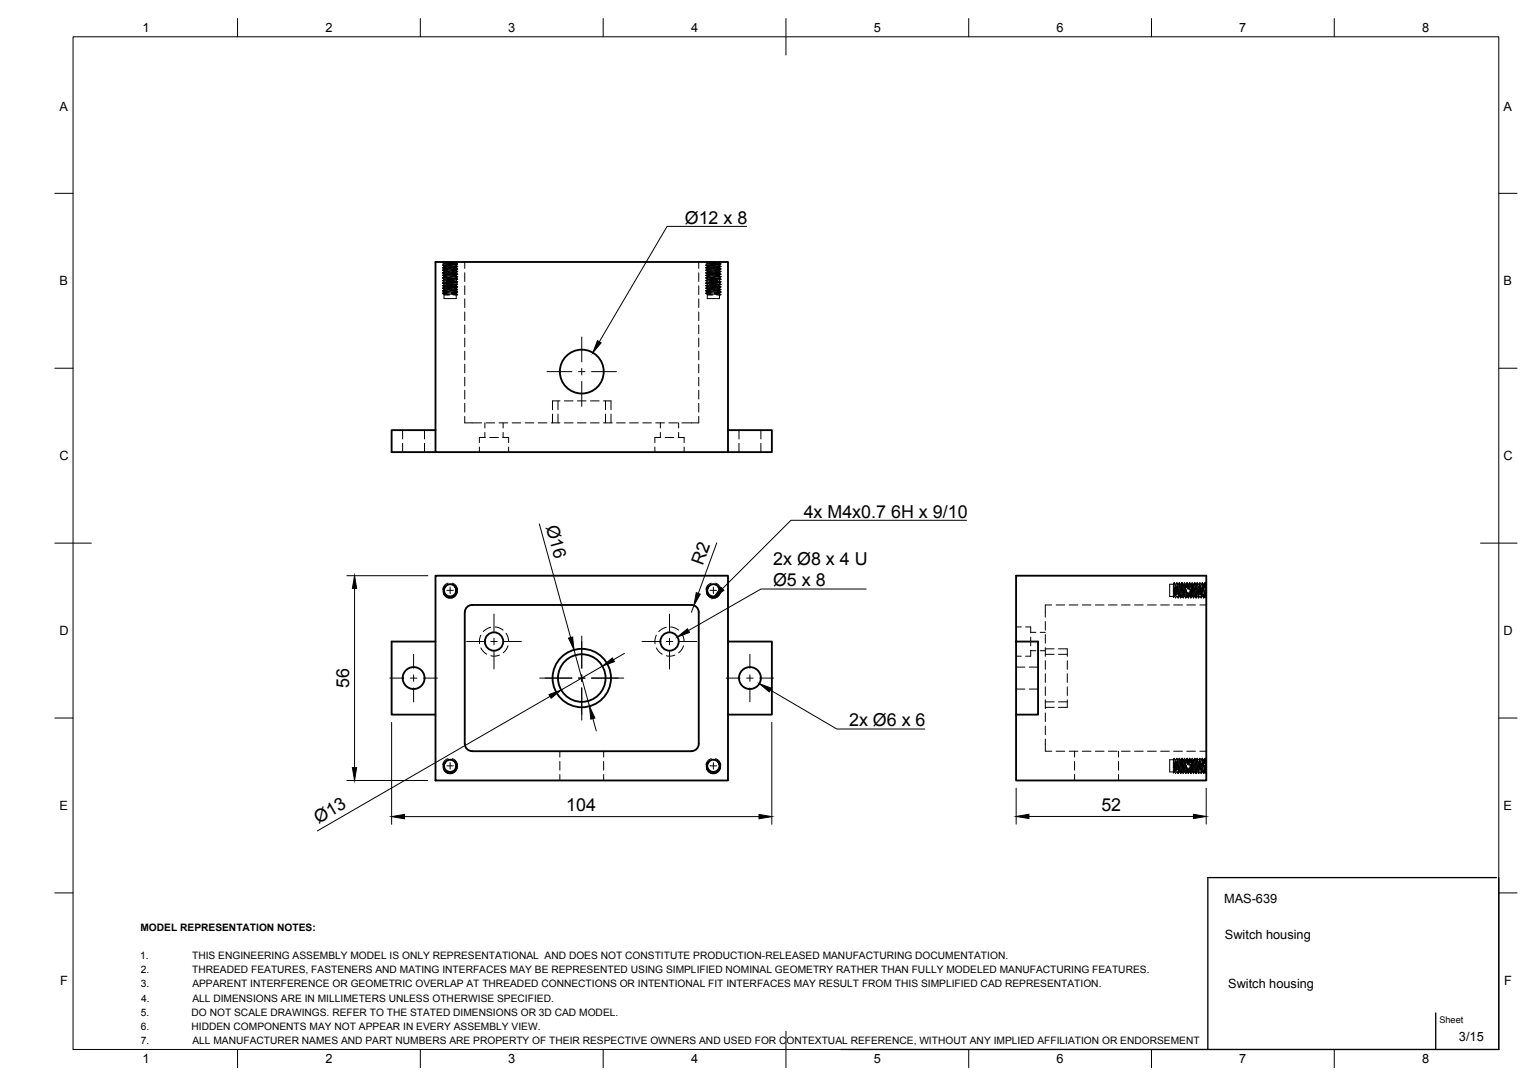
ISO-10303-21;
HEADER;
/* Generated by software containing ST-Developer
 * from STEP Tools, Inc. (www.steptools.com) 
 */

FILE_DESCRIPTION(
/* description */ ('Independent maintained push-to-latch/pull-to-reset mushroom-operator 
CAD. Two opposed spring-loaded ball detents in turned circular seats b
ias both travel stops; direct normally-closed bridge opens6mm when pre
ssed. Rounded palm/pull rim, captured head screw, removable detent clo
sures, native Coil spring families, insulated shared terminals and ord
inary machining features. Manual geometric states and ideal same-mater
ial spring-energy direction only; no electrical/safety certification, 
force/contact dynamics, wear, load or life rating. Requested blue/gray
 visual palette, not safety identification. External wiring/anchors an
d application engineering omitted.'),
/* implementation_level */ '2;1');

FILE_NAME(
/* name */ 'Switch housing.step',
/* time_stamp */ '2026-11-08T17:54:26-08:00',
/* author */ (''),
/* organization */ (''),
/* preprocessor_version */ 'ST-DEVELOPER v20.2',
/* originating_system */ 'Autodesk Translation Framework v15.17.0.0',
/* authorisation */ '');

FILE_SCHEMA (('AUTOMOTIVE_DESIGN { 1 0 10303 214 3 1 1 }'));
ENDSEC;

DATA;
#10=MECHANICAL_DESIGN_GEOMETRIC_PRESENTATION_REPRESENTATION('',(#190),#43980);
#156=SHAPE_REPRESENTATION_RELATIONSHIP('SRR','None',#44056,#173);
#173=ADVANCED_BREP_SHAPE_REPRESENTATION('',(#207),#43963);
#190=STYLED_ITEM('',(#44150),#207);
#207=MANIFOLD_SOLID_BREP('Body1',#11231);
#224=B_SPLINE_SURFACE_WITH_KNOTS('',3,3,((#18348,#18349,#18350,#18351,#18352,
#18353,#18354,#18355,#18356,#18357,#18358,#18359,#18360,#18361,#18362,#18363,
#18364,#18365,#18366,#18367,#18368,#18369,#18370,#18371,#18372,#18373,#18374,
#18375,#18376,#18377,#18378,#18379,#18380,#18381,#18382,#18383,#18384,#18385,
#18386,#18387,#18388,#18389,#18390,#18391,#18392,#18393,#18394,#18395,#18396,
#18397,#18398,#18399,#18400,#18401,#18402,#18403,#18404,#18405,#18406,#18407,
#18408,#18409,#18410,#18411,#18412,#18413,#18414,#18415,#18416,#18417,#18418,
#18419,#18420,#18421,#18422,#18423,#18424,#18425,#18426,#18427,#18428,#18429,
#18430,#18431,#18432,#18433),(#18434,#18435,#18436,#18437,#18438,#18439,
#18440,#18441,#18442,#18443,#18444,#18445,#18446,#18447,#18448,#18449,#18450,
#18451,#18452,#18453,#18454,#18455,#18456,#18457,#18458,#18459,#18460,#18461,
#18462,#18463,#18464,#18465,#18466,#18467,#18468,#18469,#18470,#18471,#18472,
#18473,#18474,#18475,#18476,#18477,#18478,#18479,#18480,#18481,#18482,#18483,
#18484,#18485,#18486,#18487,#18488,#18489,#18490,#18491,#18492,#18493,#18494,
#18495,#18496,#18497,#18498,#18499,#18500,#18501,#18502,#18503,#18504,#18505,
#18506,#18507,#18508,#18509,#18510,#18511,#18512,#18513,#18514,#18515,#18516,
#18517,#18518,#18519),(#18520,#18521,#18522,#18523,#18524,#18525,#18526,
#18527,#18528,#18529,#18530,#18531,#18532,#18533,#18534,#18535,#18536,#18537,
#18538,#18539,#18540,#18541,#18542,#18543,#18544,#18545,#18546,#18547,#18548,
#18549,#18550,#18551,#18552,#18553,#18554,#18555,#18556,#18557,#18558,#18559,
#18560,#18561,#18562,#18563,#18564,#18565,#18566,#18567,#18568,#18569,#18570,
#18571,#18572,#18573,#18574,#18575,#18576,#18577,#18578,#18579,#18580,#18581,
#18582,#18583,#18584,#18585,#18586,#18587,#18588,#18589,#18590,#18591,#18592,
#18593,#18594,#18595,#18596,#18597,#18598,#18599,#18600,#18601,#18602,#18603,
#18604,#18605),(#18606,#18607,#18608,#18609,#18610,#18611,#18612,#18613,
#18614,#18615,#18616,#18617,#18618,#18619,#18620,#18621,#18622,#18623,#18624,
#18625,#18626,#18627,#18628,#18629,#18630,#18631,#18632,#18633,#18634,#18635,
#18636,#18637,#18638,#18639,#18640,#18641,#18642,#18643,#18644,#18645,#18646,
#18647,#18648,#18649,#18650,#18651,#18652,#18653,#18654,#18655,#18656,#18657,
#18658,#18659,#18660,#18661,#18662,#18663,#18664,#18665,#18666,#18667,#18668,
#18669,#18670,#18671,#18672,#18673,#18674,#18675,#18676,#18677,#18678,#18679,
#18680,#18681,#18682,#18683,#18684,#18685,#18686,#18687,#18688,#18689,#18690,
#18691)),.UNSPECIFIED.,.F.,.F.,.F.,(4,4),(4,1,1,1,1,1,1,1,1,1,1,1,1,1,1,
1,1,1,1,1,1,1,1,1,1,1,1,1,1,1,1,1,1,1,1,1,1,1,1,1,1,1,1,1,1,1,1,1,1,1,1,
1,1,1,1,1,1,1,1,1,1,1,1,1,1,1,1,1,1,1,1,1,1,1,1,1,1,1,1,1,1,1,1,4),(0.,
0.0448889834294937),(11.8615800042567,12.8591513772396,13.8567227502226,
14.8542941232055,15.8518654961884,16.8494368691714,17.8470082421543,18.8445796151372,
19.8421509881202,20.8397223611031,21.837293734086,22.834865107069,23.8324364800519,
24.8300078530348,25.8275792260178,26.8251505990007,27.8227219719836,28.8202933449666,
29.8178647179495,30.8154360909324,31.8130074639154,32.8105788368983,33.8081502098812,
34.8057215828642,35.8032929558471,36.80086432883,37.798435701813,38.7960070747959,
39.7935784477789,40.7911498207618,41.7887211937447,42.7862925667277,43.7838639397106,
44.7814353126935,45.7790066856765,46.7765780586594,47.7741494316423,48.7717208046253,
49.7692921776082,50.7668635505911,51.7644349235741,52.762006296557,53.7595776695399,
54.7571490425229,55.7547204155058,56.7522917884887,57.7498631614717,58.7474345344546,
59.7450059074375,60.7425772804205,61.7401486534034,62.7377200263864,63.7352913993693,
64.7328627723522,65.7304341453352,66.7280055183181,67.725576891301,68.723148264284,
69.7207196372669,70.7182910102498,71.7158623832328,72.7134337562157,73.7110051291986,
74.7085765021816,75.7061478751645,76.7037192481474,77.7012906211304,78.6988619941133,
79.6964333670962,80.6940047400792,81.6915761130621,82.689147486045,83.686718859028,
84.6842902320109,85.6818616049939,86.6794329779768,87.6770043509597,88.6745757239427,
89.6721470969256,90.6697184699085,91.6672898428915,92.6648612158744,93.6624325888573,
94.6600039618403),.UNSPECIFIED.);
#225=B_SPLINE_SURFACE_WITH_KNOTS('',3,3,((#18769,#18770,#18771,#18772,#18773,
#18774,#18775,#18776,#18777,#18778,#18779,#18780,#18781,#18782,#18783,#18784,
#18785,#18786,#18787,#18788,#18789,#18790,#18791,#18792,#18793,#18794,#18795,
#18796,#18797,#18798,#18799,#18800,#18801,#18802,#18803,#18804,#18805,#18806,
#18807,#18808,#18809,#18810,#18811,#18812,#18813,#18814,#18815,#18816,#18817,
#18818,#18819,#18820,#18821,#18822,#18823,#18824,#18825,#18826,#18827,#18828,
#18829,#18830,#18831,#18832,#18833,#18834,#18835,#18836,#18837,#18838,#18839,
#18840,#18841,#18842,#18843,#18844,#18845,#18846,#18847,#18848,#18849,#18850,
#18851,#18852,#18853,#18854),(#18855,#18856,#18857,#18858,#18859,#18860,
#18861,#18862,#18863,#18864,#18865,#18866,#18867,#18868,#18869,#18870,#18871,
#18872,#18873,#18874,#18875,#18876,#18877,#18878,#18879,#18880,#18881,#18882,
#18883,#18884,#18885,#18886,#18887,#18888,#18889,#18890,#18891,#18892,#18893,
#18894,#18895,#18896,#18897,#18898,#18899,#18900,#18901,#18902,#18903,#18904,
#18905,#18906,#18907,#18908,#18909,#18910,#18911,#18912,#18913,#18914,#18915,
#18916,#18917,#18918,#18919,#18920,#18921,#18922,#18923,#18924,#18925,#18926,
#18927,#18928,#18929,#18930,#18931,#18932,#18933,#18934,#18935,#18936,#18937,
#18938,#18939,#18940),(#18941,#18942,#18943,#18944,#18945,#18946,#18947,
#18948,#18949,#18950,#18951,#18952,#18953,#18954,#18955,#18956,#18957,#18958,
#18959,#18960,#18961,#18962,#18963,#18964,#18965,#18966,#18967,#18968,#18969,
#18970,#18971,#18972,#18973,#18974,#18975,#18976,#18977,#18978,#18979,#18980,
#18981,#18982,#18983,#18984,#18985,#18986,#18987,#18988,#18989,#18990,#18991,
#18992,#18993,#18994,#18995,#18996,#18997,#18998,#18999,#19000,#19001,#19002,
#19003,#19004,#19005,#19006,#19007,#19008,#19009,#19010,#19011,#19012,#19013,
#19014,#19015,#19016,#19017,#19018,#19019,#19020,#19021,#19022,#19023,#19024,
#19025,#19026),(#19027,#19028,#19029,#19030,#19031,#19032,#19033,#19034,
#19035,#19036,#19037,#19038,#19039,#19040,#19041,#19042,#19043,#19044,#19045,
#19046,#19047,#19048,#19049,#19050,#19051,#19052,#19053,#19054,#19055,#19056,
#19057,#19058,#19059,#19060,#19061,#19062,#19063,#19064,#19065,#19066,#19067,
#19068,#19069,#19070,#19071,#19072,#19073,#19074,#19075,#19076,#19077,#19078,
#19079,#19080,#19081,#19082,#19083,#19084,#19085,#19086,#19087,#19088,#19089,
#19090,#19091,#19092,#19093,#19094,#19095,#19096,#19097,#19098,#19099,#19100,
#19101,#19102,#19103,#19104,#19105,#19106,#19107,#19108,#19109,#19110,#19111,
#19112)),.UNSPECIFIED.,.F.,.F.,.F.,(4,4),(4,1,1,1,1,1,1,1,1,1,1,1,1,1,1,
1,1,1,1,1,1,1,1,1,1,1,1,1,1,1,1,1,1,1,1,1,1,1,1,1,1,1,1,1,1,1,1,1,1,1,1,
1,1,1,1,1,1,1,1,1,1,1,1,1,1,1,1,1,1,1,1,1,1,1,1,1,1,1,1,1,1,1,1,4),(0.,
0.0448889834294937),(14.3981410127769,15.3957123857599,16.3932837587428,
17.3908551317257,18.3884265047087,19.3859978776916,20.3835692506745,21.3811406236575,
22.3787119966404,23.3762833696233,24.3738547426063,25.3714261155892,26.3689974885721,
27.3665688615551,28.364140234538,29.3617116075209,30.3592829805039,31.3568543534868,
32.3544257264697,33.3519970994527,34.3495684724356,35.3471398454185,36.3447112184015,
37.3422825913844,38.3398539643674,39.3374253373503,40.3349967103332,41.3325680833162,
42.3301394562991,43.327710829282,44.325282202265,45.3228535752479,46.3204249482308,
47.3179963212138,48.3155676941967,49.3131390671796,50.3107104401626,51.3082818131455,
52.3058531861284,53.3034245591114,54.3009959320943,55.2985673050772,56.2961386780602,
57.2937100510431,58.291281424026,59.288852797009,60.2864241699919,61.2839955429748,
62.2815669159578,63.2791382889407,64.2767096619236,65.2742810349066,66.2718524078895,
67.2694237808725,68.2669951538554,69.2645665268383,70.2621378998213,71.2597092728042,
72.2572806457871,73.2548520187701,74.252423391753,75.2499947647359,76.2475661377189,
77.2451375107018,78.2427088836847,79.2402802566677,80.2378516296506,81.2354230026336,
82.2329943756165,83.2305657485994,84.2281371215823,85.2257084945653,86.2232798675482,
87.2208512405312,88.2184226135141,89.215993986497,90.21356535948,91.2111367324629,
92.2087081054458,93.2062794784288,94.2038508514117,95.2014222243946,96.1989935973776,
97.1965649703605),.UNSPECIFIED.);
#226=B_SPLINE_SURFACE_WITH_KNOTS('',3,3,((#19321,#19322,#19323,#19324,#19325,
#19326,#19327,#19328,#19329,#19330,#19331,#19332,#19333,#19334,#19335,#19336,
#19337,#19338,#19339,#19340,#19341,#19342,#19343,#19344,#19345,#19346,#19347,
#19348,#19349,#19350,#19351,#19352,#19353,#19354,#19355,#19356,#19357,#19358,
#19359,#19360,#19361,#19362,#19363,#19364,#19365,#19366,#19367,#19368,#19369,
#19370,#19371,#19372,#19373,#19374,#19375,#19376,#19377,#19378,#19379,#19380,
#19381,#19382,#19383,#19384,#19385,#19386,#19387,#19388,#19389,#19390,#19391,
#19392,#19393,#19394,#19395,#19396,#19397,#19398,#19399,#19400,#19401,#19402,
#19403,#19404,#19405,#19406),(#19407,#19408,#19409,#19410,#19411,#19412,
#19413,#19414,#19415,#19416,#19417,#19418,#19419,#19420,#19421,#19422,#19423,
#19424,#19425,#19426,#19427,#19428,#19429,#19430,#19431,#19432,#19433,#19434,
#19435,#19436,#19437,#19438,#19439,#19440,#19441,#19442,#19443,#19444,#19445,
#19446,#19447,#19448,#19449,#19450,#19451,#19452,#19453,#19454,#19455,#19456,
#19457,#19458,#19459,#19460,#19461,#19462,#19463,#19464,#19465,#19466,#19467,
#19468,#19469,#19470,#19471,#19472,#19473,#19474,#19475,#19476,#19477,#19478,
#19479,#19480,#19481,#19482,#19483,#19484,#19485,#19486,#19487,#19488,#19489,
#19490,#19491,#19492),(#19493,#19494,#19495,#19496,#19497,#19498,#19499,
#19500,#19501,#19502,#19503,#19504,#19505,#19506,#19507,#19508,#19509,#19510,
#19511,#19512,#19513,#19514,#19515,#19516,#19517,#19518,#19519,#19520,#19521,
#19522,#19523,#19524,#19525,#19526,#19527,#19528,#19529,#19530,#19531,#19532,
#19533,#19534,#19535,#19536,#19537,#19538,#19539,#19540,#19541,#19542,#19543,
#19544,#19545,#19546,#19547,#19548,#19549,#19550,#19551,#19552,#19553,#19554,
#19555,#19556,#19557,#19558,#19559,#19560,#19561,#19562,#19563,#19564,#19565,
#19566,#19567,#19568,#19569,#19570,#19571,#19572,#19573,#19574,#19575,#19576,
#19577,#19578),(#19579,#19580,#19581,#19582,#19583,#19584,#19585,#19586,
#19587,#19588,#19589,#19590,#19591,#19592,#19593,#19594,#19595,#19596,#19597,
#19598,#19599,#19600,#19601,#19602,#19603,#19604,#19605,#19606,#19607,#19608,
#19609,#19610,#19611,#19612,#19613,#19614,#19615,#19616,#19617,#19618,#19619,
#19620,#19621,#19622,#19623,#19624,#19625,#19626,#19627,#19628,#19629,#19630,
#19631,#19632,#19633,#19634,#19635,#19636,#19637,#19638,#19639,#19640,#19641,
#19642,#19643,#19644,#19645,#19646,#19647,#19648,#19649,#19650,#19651,#19652,
#19653,#19654,#19655,#19656,#19657,#19658,#19659,#19660,#19661,#19662,#19663,
#19664)),.UNSPECIFIED.,.F.,.F.,.F.,(4,4),(4,1,1,1,1,1,1,1,1,1,1,1,1,1,1,
1,1,1,1,1,1,1,1,1,1,1,1,1,1,1,1,1,1,1,1,1,1,1,1,1,1,1,1,1,1,1,1,1,1,1,1,
1,1,1,1,1,1,1,1,1,1,1,1,1,1,1,1,1,1,1,1,1,1,1,1,1,1,1,1,1,1,1,1,4),(0.,
0.0448889834294937),(11.8615800042567,12.8591513772396,13.8567227502225,
14.8542941232055,15.8518654961884,16.8494368691713,17.8470082421543,18.8445796151372,
19.8421509881202,20.8397223611031,21.837293734086,22.834865107069,23.8324364800519,
24.8300078530348,25.8275792260178,26.8251505990007,27.8227219719836,28.8202933449666,
29.8178647179495,30.8154360909324,31.8130074639154,32.8105788368983,33.8081502098812,
34.8057215828642,35.8032929558471,36.80086432883,37.798435701813,38.7960070747959,
39.7935784477788,40.7911498207618,41.7887211937447,42.7862925667276,43.7838639397106,
44.7814353126935,45.7790066856764,46.7765780586594,47.7741494316423,48.7717208046252,
49.7692921776082,50.7668635505911,51.764434923574,52.762006296557,53.7595776695399,
54.7571490425228,55.7547204155058,56.7522917884887,57.7498631614716,58.7474345344546,
59.7450059074375,60.7425772804204,61.7401486534034,62.7377200263863,63.7352913993692,
64.7328627723522,65.7304341453351,66.728005518318,67.725576891301,68.7231482642839,
69.7207196372669,70.7182910102498,71.7158623832327,72.7134337562156,73.7110051291986,
74.7085765021815,75.7061478751644,76.7037192481474,77.7012906211303,78.6988619941132,
79.6964333670962,80.6940047400791,81.6915761130621,82.689147486045,83.6867188590279,
84.6842902320109,85.6818616049938,86.6794329779767,87.6770043509596,88.6745757239426,
89.6721470969255,90.6697184699085,91.6672898428914,92.6648612158743,93.6624325888573,
94.6600039618402),.UNSPECIFIED.);
#227=B_SPLINE_SURFACE_WITH_KNOTS('',3,3,((#19742,#19743,#19744,#19745,#19746,
#19747,#19748,#19749,#19750,#19751,#19752,#19753,#19754,#19755,#19756,#19757,
#19758,#19759,#19760,#19761,#19762,#19763,#19764,#19765,#19766,#19767,#19768,
#19769,#19770,#19771,#19772,#19773,#19774,#19775,#19776,#19777,#19778,#19779,
#19780,#19781,#19782,#19783,#19784,#19785,#19786,#19787,#19788,#19789,#19790,
#19791,#19792,#19793,#19794,#19795,#19796,#19797,#19798,#19799,#19800,#19801,
#19802,#19803,#19804,#19805,#19806,#19807,#19808,#19809,#19810,#19811,#19812,
#19813,#19814,#19815,#19816,#19817,#19818,#19819,#19820,#19821,#19822,#19823,
#19824,#19825,#19826,#19827),(#19828,#19829,#19830,#19831,#19832,#19833,
#19834,#19835,#19836,#19837,#19838,#19839,#19840,#19841,#19842,#19843,#19844,
#19845,#19846,#19847,#19848,#19849,#19850,#19851,#19852,#19853,#19854,#19855,
#19856,#19857,#19858,#19859,#19860,#19861,#19862,#19863,#19864,#19865,#19866,
#19867,#19868,#19869,#19870,#19871,#19872,#19873,#19874,#19875,#19876,#19877,
#19878,#19879,#19880,#19881,#19882,#19883,#19884,#19885,#19886,#19887,#19888,
#19889,#19890,#19891,#19892,#19893,#19894,#19895,#19896,#19897,#19898,#19899,
#19900,#19901,#19902,#19903,#19904,#19905,#19906,#19907,#19908,#19909,#19910,
#19911,#19912,#19913),(#19914,#19915,#19916,#19917,#19918,#19919,#19920,
#19921,#19922,#19923,#19924,#19925,#19926,#19927,#19928,#19929,#19930,#19931,
#19932,#19933,#19934,#19935,#19936,#19937,#19938,#19939,#19940,#19941,#19942,
#19943,#19944,#19945,#19946,#19947,#19948,#19949,#19950,#19951,#19952,#19953,
#19954,#19955,#19956,#19957,#19958,#19959,#19960,#19961,#19962,#19963,#19964,
#19965,#19966,#19967,#19968,#19969,#19970,#19971,#19972,#19973,#19974,#19975,
#19976,#19977,#19978,#19979,#19980,#19981,#19982,#19983,#19984,#19985,#19986,
#19987,#19988,#19989,#19990,#19991,#19992,#19993,#19994,#19995,#19996,#19997,
#19998,#19999),(#20000,#20001,#20002,#20003,#20004,#20005,#20006,#20007,
#20008,#20009,#20010,#20011,#20012,#20013,#20014,#20015,#20016,#20017,#20018,
#20019,#20020,#20021,#20022,#20023,#20024,#20025,#20026,#20027,#20028,#20029,
#20030,#20031,#20032,#20033,#20034,#20035,#20036,#20037,#20038,#20039,#20040,
#20041,#20042,#20043,#20044,#20045,#20046,#20047,#20048,#20049,#20050,#20051,
#20052,#20053,#20054,#20055,#20056,#20057,#20058,#20059,#20060,#20061,#20062,
#20063,#20064,#20065,#20066,#20067,#20068,#20069,#20070,#20071,#20072,#20073,
#20074,#20075,#20076,#20077,#20078,#20079,#20080,#20081,#20082,#20083,#20084,
#20085)),.UNSPECIFIED.,.F.,.F.,.F.,(4,4),(4,1,1,1,1,1,1,1,1,1,1,1,1,1,1,
1,1,1,1,1,1,1,1,1,1,1,1,1,1,1,1,1,1,1,1,1,1,1,1,1,1,1,1,1,1,1,1,1,1,1,1,
1,1,1,1,1,1,1,1,1,1,1,1,1,1,1,1,1,1,1,1,1,1,1,1,1,1,1,1,1,1,1,1,4),(0.,
0.0448889834294937),(14.3981410127769,15.3957123857599,16.3932837587428,
17.3908551317257,18.3884265047087,19.3859978776916,20.3835692506745,21.3811406236575,
22.3787119966404,23.3762833696233,24.3738547426063,25.3714261155892,26.3689974885721,
27.3665688615551,28.364140234538,29.3617116075209,30.3592829805039,31.3568543534868,
32.3544257264697,33.3519970994527,34.3495684724356,35.3471398454185,36.3447112184015,
37.3422825913844,38.3398539643673,39.3374253373503,40.3349967103332,41.3325680833161,
42.3301394562991,43.327710829282,44.3252822022649,45.3228535752479,46.3204249482308,
47.3179963212137,48.3155676941967,49.3131390671796,50.3107104401625,51.3082818131455,
52.3058531861284,53.3034245591113,54.3009959320943,55.2985673050772,56.2961386780601,
57.2937100510431,58.291281424026,59.2888527970089,60.2864241699919,61.2839955429748,
62.2815669159577,63.2791382889407,64.2767096619236,65.2742810349065,66.2718524078895,
67.2694237808724,68.2669951538553,69.2645665268383,70.2621378998212,71.2597092728041,
72.2572806457871,73.25485201877,74.2524233917529,75.2499947647359,76.2475661377188,
77.2451375107017,78.2427088836847,79.2402802566676,80.2378516296505,81.2354230026335,
82.2329943756164,83.2305657485993,84.2281371215823,85.2257084945652,86.2232798675481,
87.2208512405311,88.218422613514,89.2159939864969,90.2135653594799,91.2111367324628,
92.2087081054457,93.2062794784287,94.2038508514116,95.2014222243945,96.1989935973775,
97.1965649703604),.UNSPECIFIED.);
#228=B_SPLINE_SURFACE_WITH_KNOTS('',3,3,((#20294,#20295,#20296,#20297,#20298,
#20299,#20300,#20301,#20302,#20303,#20304,#20305,#20306,#20307,#20308,#20309,
#20310,#20311,#20312,#20313,#20314,#20315,#20316,#20317,#20318,#20319,#20320,
#20321,#20322,#20323,#20324,#20325,#20326,#20327,#20328,#20329,#20330,#20331,
#20332,#20333,#20334,#20335,#20336,#20337,#20338,#20339,#20340,#20341,#20342,
#20343,#20344,#20345,#20346,#20347,#20348,#20349,#20350,#20351,#20352,#20353,
#20354,#20355,#20356,#20357,#20358,#20359,#20360,#20361,#20362,#20363,#20364,
#20365,#20366,#20367,#20368,#20369,#20370,#20371,#20372,#20373,#20374,#20375,
#20376,#20377,#20378,#20379),(#20380,#20381,#20382,#20383,#20384,#20385,
#20386,#20387,#20388,#20389,#20390,#20391,#20392,#20393,#20394,#20395,#20396,
#20397,#20398,#20399,#20400,#20401,#20402,#20403,#20404,#20405,#20406,#20407,
#20408,#20409,#20410,#20411,#20412,#20413,#20414,#20415,#20416,#20417,#20418,
#20419,#20420,#20421,#20422,#20423,#20424,#20425,#20426,#20427,#20428,#20429,
#20430,#20431,#20432,#20433,#20434,#20435,#20436,#20437,#20438,#20439,#20440,
#20441,#20442,#20443,#20444,#20445,#20446,#20447,#20448,#20449,#20450,#20451,
#20452,#20453,#20454,#20455,#20456,#20457,#20458,#20459,#20460,#20461,#20462,
#20463,#20464,#20465),(#20466,#20467,#20468,#20469,#20470,#20471,#20472,
#20473,#20474,#20475,#20476,#20477,#20478,#20479,#20480,#20481,#20482,#20483,
#20484,#20485,#20486,#20487,#20488,#20489,#20490,#20491,#20492,#20493,#20494,
#20495,#20496,#20497,#20498,#20499,#20500,#20501,#20502,#20503,#20504,#20505,
#20506,#20507,#20508,#20509,#20510,#20511,#20512,#20513,#20514,#20515,#20516,
#20517,#20518,#20519,#20520,#20521,#20522,#20523,#20524,#20525,#20526,#20527,
#20528,#20529,#20530,#20531,#20532,#20533,#20534,#20535,#20536,#20537,#20538,
#20539,#20540,#20541,#20542,#20543,#20544,#20545,#20546,#20547,#20548,#20549,
#20550,#20551),(#20552,#20553,#20554,#20555,#20556,#20557,#20558,#20559,
#20560,#20561,#20562,#20563,#20564,#20565,#20566,#20567,#20568,#20569,#20570,
#20571,#20572,#20573,#20574,#20575,#20576,#20577,#20578,#20579,#20580,#20581,
#20582,#20583,#20584,#20585,#20586,#20587,#20588,#20589,#20590,#20591,#20592,
#20593,#20594,#20595,#20596,#20597,#20598,#20599,#20600,#20601,#20602,#20603,
#20604,#20605,#20606,#20607,#20608,#20609,#20610,#20611,#20612,#20613,#20614,
#20615,#20616,#20617,#20618,#20619,#20620,#20621,#20622,#20623,#20624,#20625,
#20626,#20627,#20628,#20629,#20630,#20631,#20632,#20633,#20634,#20635,#20636,
#20637)),.UNSPECIFIED.,.F.,.F.,.F.,(4,4),(4,1,1,1,1,1,1,1,1,1,1,1,1,1,1,
1,1,1,1,1,1,1,1,1,1,1,1,1,1,1,1,1,1,1,1,1,1,1,1,1,1,1,1,1,1,1,1,1,1,1,1,
1,1,1,1,1,1,1,1,1,1,1,1,1,1,1,1,1,1,1,1,1,1,1,1,1,1,1,1,1,1,1,1,4),(0.,
0.0448889834294937),(11.8615800042567,12.8591513772396,13.8567227502225,
14.8542941232055,15.8518654961884,16.8494368691713,17.8470082421543,18.8445796151372,
19.8421509881201,20.8397223611031,21.837293734086,22.8348651070689,23.8324364800519,
24.8300078530348,25.8275792260178,26.8251505990007,27.8227219719836,28.8202933449666,
29.8178647179495,30.8154360909324,31.8130074639154,32.8105788368983,33.8081502098812,
34.8057215828642,35.8032929558471,36.80086432883,37.798435701813,38.7960070747959,
39.7935784477788,40.7911498207618,41.7887211937447,42.7862925667276,43.7838639397106,
44.7814353126935,45.7790066856764,46.7765780586594,47.7741494316423,48.7717208046252,
49.7692921776082,50.7668635505911,51.764434923574,52.762006296557,53.7595776695399,
54.7571490425228,55.7547204155058,56.7522917884887,57.7498631614716,58.7474345344546,
59.7450059074375,60.7425772804204,61.7401486534034,62.7377200263863,63.7352913993692,
64.7328627723522,65.7304341453351,66.728005518318,67.725576891301,68.7231482642839,
69.7207196372668,70.7182910102498,71.7158623832327,72.7134337562156,73.7110051291986,
74.7085765021815,75.7061478751644,76.7037192481474,77.7012906211303,78.6988619941132,
79.6964333670962,80.6940047400791,81.6915761130621,82.689147486045,83.6867188590279,
84.6842902320109,85.6818616049938,86.6794329779767,87.6770043509596,88.6745757239426,
89.6721470969255,90.6697184699085,91.6672898428914,92.6648612158743,93.6624325888573,
94.6600039618402),.UNSPECIFIED.);
#229=B_SPLINE_SURFACE_WITH_KNOTS('',3,3,((#20715,#20716,#20717,#20718,#20719,
#20720,#20721,#20722,#20723,#20724,#20725,#20726,#20727,#20728,#20729,#20730,
#20731,#20732,#20733,#20734,#20735,#20736,#20737,#20738,#20739,#20740,#20741,
#20742,#20743,#20744,#20745,#20746,#20747,#20748,#20749,#20750,#20751,#20752,
#20753,#20754,#20755,#20756,#20757,#20758,#20759,#20760,#20761,#20762,#20763,
#20764,#20765,#20766,#20767,#20768,#20769,#20770,#20771,#20772,#20773,#20774,
#20775,#20776,#20777,#20778,#20779,#20780,#20781,#20782,#20783,#20784,#20785,
#20786,#20787,#20788,#20789,#20790,#20791,#20792,#20793,#20794,#20795,#20796,
#20797,#20798,#20799,#20800),(#20801,#20802,#20803,#20804,#20805,#20806,
#20807,#20808,#20809,#20810,#20811,#20812,#20813,#20814,#20815,#20816,#20817,
#20818,#20819,#20820,#20821,#20822,#20823,#20824,#20825,#20826,#20827,#20828,
#20829,#20830,#20831,#20832,#20833,#20834,#20835,#20836,#20837,#20838,#20839,
#20840,#20841,#20842,#20843,#20844,#20845,#20846,#20847,#20848,#20849,#20850,
#20851,#20852,#20853,#20854,#20855,#20856,#20857,#20858,#20859,#20860,#20861,
#20862,#20863,#20864,#20865,#20866,#20867,#20868,#20869,#20870,#20871,#20872,
#20873,#20874,#20875,#20876,#20877,#20878,#20879,#20880,#20881,#20882,#20883,
#20884,#20885,#20886),(#20887,#20888,#20889,#20890,#20891,#20892,#20893,
#20894,#20895,#20896,#20897,#20898,#20899,#20900,#20901,#20902,#20903,#20904,
#20905,#20906,#20907,#20908,#20909,#20910,#20911,#20912,#20913,#20914,#20915,
#20916,#20917,#20918,#20919,#20920,#20921,#20922,#20923,#20924,#20925,#20926,
#20927,#20928,#20929,#20930,#20931,#20932,#20933,#20934,#20935,#20936,#20937,
#20938,#20939,#20940,#20941,#20942,#20943,#20944,#20945,#20946,#20947,#20948,
#20949,#20950,#20951,#20952,#20953,#20954,#20955,#20956,#20957,#20958,#20959,
#20960,#20961,#20962,#20963,#20964,#20965,#20966,#20967,#20968,#20969,#20970,
#20971,#20972),(#20973,#20974,#20975,#20976,#20977,#20978,#20979,#20980,
#20981,#20982,#20983,#20984,#20985,#20986,#20987,#20988,#20989,#20990,#20991,
#20992,#20993,#20994,#20995,#20996,#20997,#20998,#20999,#21000,#21001,#21002,
#21003,#21004,#21005,#21006,#21007,#21008,#21009,#21010,#21011,#21012,#21013,
#21014,#21015,#21016,#21017,#21018,#21019,#21020,#21021,#21022,#21023,#21024,
#21025,#21026,#21027,#21028,#21029,#21030,#21031,#21032,#21033,#21034,#21035,
#21036,#21037,#21038,#21039,#21040,#21041,#21042,#21043,#21044,#21045,#21046,
#21047,#21048,#21049,#21050,#21051,#21052,#21053,#21054,#21055,#21056,#21057,
#21058)),.UNSPECIFIED.,.F.,.F.,.F.,(4,4),(4,1,1,1,1,1,1,1,1,1,1,1,1,1,1,
1,1,1,1,1,1,1,1,1,1,1,1,1,1,1,1,1,1,1,1,1,1,1,1,1,1,1,1,1,1,1,1,1,1,1,1,
1,1,1,1,1,1,1,1,1,1,1,1,1,1,1,1,1,1,1,1,1,1,1,1,1,1,1,1,1,1,1,1,4),(0.,
0.0448889834294937),(14.3981410127769,15.3957123857599,16.3932837587428,
17.3908551317257,18.3884265047087,19.3859978776916,20.3835692506745,21.3811406236575,
22.3787119966404,23.3762833696233,24.3738547426063,25.3714261155892,26.3689974885721,
27.3665688615551,28.364140234538,29.3617116075209,30.3592829805039,31.3568543534868,
32.3544257264697,33.3519970994527,34.3495684724356,35.3471398454185,36.3447112184015,
37.3422825913844,38.3398539643673,39.3374253373503,40.3349967103332,41.3325680833161,
42.3301394562991,43.327710829282,44.3252822022649,45.3228535752479,46.3204249482308,
47.3179963212137,48.3155676941967,49.3131390671796,50.3107104401625,51.3082818131455,
52.3058531861284,53.3034245591113,54.3009959320943,55.2985673050772,56.2961386780601,
57.2937100510431,58.291281424026,59.2888527970089,60.2864241699919,61.2839955429748,
62.2815669159577,63.2791382889407,64.2767096619236,65.2742810349065,66.2718524078895,
67.2694237808724,68.2669951538553,69.2645665268383,70.2621378998212,71.2597092728041,
72.2572806457871,73.25485201877,74.2524233917529,75.2499947647359,76.2475661377188,
77.2451375107017,78.2427088836847,79.2402802566676,80.2378516296505,81.2354230026335,
82.2329943756164,83.2305657485993,84.2281371215823,85.2257084945652,86.2232798675481,
87.2208512405311,88.218422613514,89.2159939864969,90.2135653594799,91.2111367324628,
92.2087081054457,93.2062794784287,94.2038508514116,95.2014222243945,96.1989935973775,
97.1965649703604),.UNSPECIFIED.);
#230=B_SPLINE_SURFACE_WITH_KNOTS('',3,3,((#21267,#21268,#21269,#21270,#21271,
#21272,#21273,#21274,#21275,#21276,#21277,#21278,#21279,#21280,#21281,#21282,
#21283,#21284,#21285,#21286,#21287,#21288,#21289,#21290,#21291,#21292,#21293,
#21294,#21295,#21296,#21297,#21298,#21299,#21300,#21301,#21302,#21303,#21304,
#21305,#21306,#21307,#21308,#21309,#21310,#21311,#21312,#21313,#21314,#21315,
#21316,#21317,#21318,#21319,#21320,#21321,#21322,#21323,#21324,#21325,#21326,
#21327,#21328,#21329,#21330,#21331,#21332,#21333,#21334,#21335,#21336,#21337,
#21338,#21339,#21340,#21341,#21342,#21343,#21344,#21345,#21346,#21347,#21348,
#21349,#21350,#21351,#21352),(#21353,#21354,#21355,#21356,#21357,#21358,
#21359,#21360,#21361,#21362,#21363,#21364,#21365,#21366,#21367,#21368,#21369,
#21370,#21371,#21372,#21373,#21374,#21375,#21376,#21377,#21378,#21379,#21380,
#21381,#21382,#21383,#21384,#21385,#21386,#21387,#21388,#21389,#21390,#21391,
#21392,#21393,#21394,#21395,#21396,#21397,#21398,#21399,#21400,#21401,#21402,
#21403,#21404,#21405,#21406,#21407,#21408,#21409,#21410,#21411,#21412,#21413,
#21414,#21415,#21416,#21417,#21418,#21419,#21420,#21421,#21422,#21423,#21424,
#21425,#21426,#21427,#21428,#21429,#21430,#21431,#21432,#21433,#21434,#21435,
#21436,#21437,#21438),(#21439,#21440,#21441,#21442,#21443,#21444,#21445,
#21446,#21447,#21448,#21449,#21450,#21451,#21452,#21453,#21454,#21455,#21456,
#21457,#21458,#21459,#21460,#21461,#21462,#21463,#21464,#21465,#21466,#21467,
#21468,#21469,#21470,#21471,#21472,#21473,#21474,#21475,#21476,#21477,#21478,
#21479,#21480,#21481,#21482,#21483,#21484,#21485,#21486,#21487,#21488,#21489,
#21490,#21491,#21492,#21493,#21494,#21495,#21496,#21497,#21498,#21499,#21500,
#21501,#21502,#21503,#21504,#21505,#21506,#21507,#21508,#21509,#21510,#21511,
#21512,#21513,#21514,#21515,#21516,#21517,#21518,#21519,#21520,#21521,#21522,
#21523,#21524),(#21525,#21526,#21527,#21528,#21529,#21530,#21531,#21532,
#21533,#21534,#21535,#21536,#21537,#21538,#21539,#21540,#21541,#21542,#21543,
#21544,#21545,#21546,#21547,#21548,#21549,#21550,#21551,#21552,#21553,#21554,
#21555,#21556,#21557,#21558,#21559,#21560,#21561,#21562,#21563,#21564,#21565,
#21566,#21567,#21568,#21569,#21570,#21571,#21572,#21573,#21574,#21575,#21576,
#21577,#21578,#21579,#21580,#21581,#21582,#21583,#21584,#21585,#21586,#21587,
#21588,#21589,#21590,#21591,#21592,#21593,#21594,#21595,#21596,#21597,#21598,
#21599,#21600,#21601,#21602,#21603,#21604,#21605,#21606,#21607,#21608,#21609,
#21610)),.UNSPECIFIED.,.F.,.F.,.F.,(4,4),(4,1,1,1,1,1,1,1,1,1,1,1,1,1,1,
1,1,1,1,1,1,1,1,1,1,1,1,1,1,1,1,1,1,1,1,1,1,1,1,1,1,1,1,1,1,1,1,1,1,1,1,
1,1,1,1,1,1,1,1,1,1,1,1,1,1,1,1,1,1,1,1,1,1,1,1,1,1,1,1,1,1,1,1,4),(0.,
0.0448889834294937),(11.8615800042567,12.8591513772396,13.8567227502226,
14.8542941232055,15.8518654961884,16.8494368691714,17.8470082421543,18.8445796151372,
19.8421509881202,20.8397223611031,21.837293734086,22.834865107069,23.8324364800519,
24.8300078530348,25.8275792260178,26.8251505990007,27.8227219719836,28.8202933449666,
29.8178647179495,30.8154360909324,31.8130074639154,32.8105788368983,33.8081502098812,
34.8057215828642,35.8032929558471,36.80086432883,37.798435701813,38.7960070747959,
39.7935784477789,40.7911498207618,41.7887211937447,42.7862925667277,43.7838639397106,
44.7814353126935,45.7790066856765,46.7765780586594,47.7741494316423,48.7717208046253,
49.7692921776082,50.7668635505911,51.7644349235741,52.762006296557,53.7595776695399,
54.7571490425229,55.7547204155058,56.7522917884887,57.7498631614717,58.7474345344546,
59.7450059074375,60.7425772804205,61.7401486534034,62.7377200263864,63.7352913993693,
64.7328627723522,65.7304341453352,66.7280055183181,67.725576891301,68.723148264284,
69.7207196372669,70.7182910102498,71.7158623832328,72.7134337562157,73.7110051291986,
74.7085765021816,75.7061478751645,76.7037192481474,77.7012906211304,78.6988619941133,
79.6964333670962,80.6940047400792,81.6915761130621,82.689147486045,83.686718859028,
84.6842902320109,85.6818616049939,86.6794329779768,87.6770043509597,88.6745757239427,
89.6721470969256,90.6697184699085,91.6672898428915,92.6648612158744,93.6624325888573,
94.6600039618403),.UNSPECIFIED.);
#231=B_SPLINE_SURFACE_WITH_KNOTS('',3,3,((#21688,#21689,#21690,#21691,#21692,
#21693,#21694,#21695,#21696,#21697,#21698,#21699,#21700,#21701,#21702,#21703,
#21704,#21705,#21706,#21707,#21708,#21709,#21710,#21711,#21712,#21713,#21714,
#21715,#21716,#21717,#21718,#21719,#21720,#21721,#21722,#21723,#21724,#21725,
#21726,#21727,#21728,#21729,#21730,#21731,#21732,#21733,#21734,#21735,#21736,
#21737,#21738,#21739,#21740,#21741,#21742,#21743,#21744,#21745,#21746,#21747,
#21748,#21749,#21750,#21751,#21752,#21753,#21754,#21755,#21756,#21757,#21758,
#21759,#21760,#21761,#21762,#21763,#21764,#21765,#21766,#21767,#21768,#21769,
#21770,#21771,#21772,#21773),(#21774,#21775,#21776,#21777,#21778,#21779,
#21780,#21781,#21782,#21783,#21784,#21785,#21786,#21787,#21788,#21789,#21790,
#21791,#21792,#21793,#21794,#21795,#21796,#21797,#21798,#21799,#21800,#21801,
#21802,#21803,#21804,#21805,#21806,#21807,#21808,#21809,#21810,#21811,#21812,
#21813,#21814,#21815,#21816,#21817,#21818,#21819,#21820,#21821,#21822,#21823,
#21824,#21825,#21826,#21827,#21828,#21829,#21830,#21831,#21832,#21833,#21834,
#21835,#21836,#21837,#21838,#21839,#21840,#21841,#21842,#21843,#21844,#21845,
#21846,#21847,#21848,#21849,#21850,#21851,#21852,#21853,#21854,#21855,#21856,
#21857,#21858,#21859),(#21860,#21861,#21862,#21863,#21864,#21865,#21866,
#21867,#21868,#21869,#21870,#21871,#21872,#21873,#21874,#21875,#21876,#21877,
#21878,#21879,#21880,#21881,#21882,#21883,#21884,#21885,#21886,#21887,#21888,
#21889,#21890,#21891,#21892,#21893,#21894,#21895,#21896,#21897,#21898,#21899,
#21900,#21901,#21902,#21903,#21904,#21905,#21906,#21907,#21908,#21909,#21910,
#21911,#21912,#21913,#21914,#21915,#21916,#21917,#21918,#21919,#21920,#21921,
#21922,#21923,#21924,#21925,#21926,#21927,#21928,#21929,#21930,#21931,#21932,
#21933,#21934,#21935,#21936,#21937,#21938,#21939,#21940,#21941,#21942,#21943,
#21944,#21945),(#21946,#21947,#21948,#21949,#21950,#21951,#21952,#21953,
#21954,#21955,#21956,#21957,#21958,#21959,#21960,#21961,#21962,#21963,#21964,
#21965,#21966,#21967,#21968,#21969,#21970,#21971,#21972,#21973,#21974,#21975,
#21976,#21977,#21978,#21979,#21980,#21981,#21982,#21983,#21984,#21985,#21986,
#21987,#21988,#21989,#21990,#21991,#21992,#21993,#21994,#21995,#21996,#21997,
#21998,#21999,#22000,#22001,#22002,#22003,#22004,#22005,#22006,#22007,#22008,
#22009,#22010,#22011,#22012,#22013,#22014,#22015,#22016,#22017,#22018,#22019,
#22020,#22021,#22022,#22023,#22024,#22025,#22026,#22027,#22028,#22029,#22030,
#22031)),.UNSPECIFIED.,.F.,.F.,.F.,(4,4),(4,1,1,1,1,1,1,1,1,1,1,1,1,1,1,
1,1,1,1,1,1,1,1,1,1,1,1,1,1,1,1,1,1,1,1,1,1,1,1,1,1,1,1,1,1,1,1,1,1,1,1,
1,1,1,1,1,1,1,1,1,1,1,1,1,1,1,1,1,1,1,1,1,1,1,1,1,1,1,1,1,1,1,1,4),(0.,
0.0448889834294937),(14.3981410127769,15.3957123857599,16.3932837587428,
17.3908551317257,18.3884265047087,19.3859978776916,20.3835692506745,21.3811406236575,
22.3787119966404,23.3762833696233,24.3738547426063,25.3714261155892,26.3689974885721,
27.3665688615551,28.364140234538,29.3617116075209,30.3592829805039,31.3568543534868,
32.3544257264697,33.3519970994527,34.3495684724356,35.3471398454185,36.3447112184015,
37.3422825913844,38.3398539643674,39.3374253373503,40.3349967103332,41.3325680833162,
42.3301394562991,43.327710829282,44.325282202265,45.3228535752479,46.3204249482308,
47.3179963212138,48.3155676941967,49.3131390671796,50.3107104401626,51.3082818131455,
52.3058531861284,53.3034245591114,54.3009959320943,55.2985673050772,56.2961386780602,
57.2937100510431,58.291281424026,59.288852797009,60.2864241699919,61.2839955429748,
62.2815669159578,63.2791382889407,64.2767096619237,65.2742810349066,66.2718524078895,
67.2694237808725,68.2669951538554,69.2645665268383,70.2621378998213,71.2597092728042,
72.2572806457871,73.2548520187701,74.252423391753,75.2499947647359,76.2475661377189,
77.2451375107018,78.2427088836847,79.2402802566677,80.2378516296506,81.2354230026336,
82.2329943756165,83.2305657485994,84.2281371215823,85.2257084945653,86.2232798675482,
87.2208512405312,88.2184226135141,89.215993986497,90.21356535948,91.2111367324629,
92.2087081054458,93.2062794784288,94.2038508514117,95.2014222243946,96.1989935973776,
97.1965649703605),.UNSPECIFIED.);
#258=FACE_BOUND('',#1208,.T.);
#259=FACE_BOUND('',#1212,.T.);
#260=FACE_BOUND('',#1245,.T.);
#261=FACE_BOUND('',#1250,.T.);
#262=FACE_BOUND('',#1254,.T.);
#263=FACE_BOUND('',#1256,.T.);
#264=FACE_BOUND('',#1257,.T.);
#265=FACE_BOUND('',#1258,.T.);
#266=FACE_BOUND('',#1266,.T.);
#267=FACE_BOUND('',#1272,.T.);
#268=FACE_BOUND('',#1275,.T.);
#269=FACE_BOUND('',#1276,.T.);
#270=FACE_BOUND('',#1277,.T.);
#271=FACE_BOUND('',#1278,.T.);
#272=FACE_BOUND('',#1279,.T.);
#273=FACE_BOUND('',#1281,.T.);
#274=FACE_BOUND('',#1282,.T.);
#275=FACE_BOUND('',#1283,.T.);
#276=FACE_BOUND('',#1284,.T.);
#331=PLANE('',#11561);
#332=PLANE('',#11568);
#333=PLANE('',#11575);
#334=PLANE('',#11578);
#335=PLANE('',#11581);
#336=PLANE('',#11584);
#337=PLANE('',#11587);
#338=PLANE('',#11588);
#339=PLANE('',#11589);
#340=PLANE('',#11590);
#341=PLANE('',#11597);
#342=PLANE('',#11598);
#343=PLANE('',#11599);
#344=PLANE('',#11600);
#345=PLANE('',#11601);
#346=PLANE('',#11602);
#347=PLANE('',#11603);
#348=PLANE('',#11604);
#349=PLANE('',#11611);
#350=PLANE('',#11612);
#351=PLANE('',#11619);
#352=PLANE('',#11622);
#353=PLANE('',#11625);
#354=PLANE('',#11626);
#355=PLANE('',#11629);
#356=PLANE('',#11630);
#357=PLANE('',#11631);
#358=PLANE('',#11632);
#359=PLANE('',#11633);
#360=PLANE('',#11634);
#361=PLANE('',#11635);
#484=FACE_OUTER_BOUND('',#1106,.T.);
#485=FACE_OUTER_BOUND('',#1107,.T.);
#486=FACE_OUTER_BOUND('',#1108,.T.);
#487=FACE_OUTER_BOUND('',#1109,.T.);
#488=FACE_OUTER_BOUND('',#1110,.T.);
#489=FACE_OUTER_BOUND('',#1111,.T.);
#490=FACE_OUTER_BOUND('',#1112,.T.);
#491=FACE_OUTER_BOUND('',#1113,.T.);
#492=FACE_OUTER_BOUND('',#1114,.T.);
#493=FACE_OUTER_BOUND('',#1115,.T.);
#494=FACE_OUTER_BOUND('',#1116,.T.);
#495=FACE_OUTER_BOUND('',#1117,.T.);
#496=FACE_OUTER_BOUND('',#1118,.T.);
#497=FACE_OUTER_BOUND('',#1119,.T.);
#498=FACE_OUTER_BOUND('',#1120,.T.);
#499=FACE_OUTER_BOUND('',#1121,.T.);
#500=FACE_OUTER_BOUND('',#1122,.T.);
#501=FACE_OUTER_BOUND('',#1123,.T.);
#502=FACE_OUTER_BOUND('',#1124,.T.);
#503=FACE_OUTER_BOUND('',#1125,.T.);
#504=FACE_OUTER_BOUND('',#1126,.T.);
#505=FACE_OUTER_BOUND('',#1127,.T.);
#506=FACE_OUTER_BOUND('',#1128,.T.);
#507=FACE_OUTER_BOUND('',#1129,.T.);
#508=FACE_OUTER_BOUND('',#1130,.T.);
#509=FACE_OUTER_BOUND('',#1131,.T.);
#510=FACE_OUTER_BOUND('',#1132,.T.);
#511=FACE_OUTER_BOUND('',#1133,.T.);
#512=FACE_OUTER_BOUND('',#1134,.T.);
#513=FACE_OUTER_BOUND('',#1135,.T.);
#514=FACE_OUTER_BOUND('',#1136,.T.);
#515=FACE_OUTER_BOUND('',#1137,.T.);
#516=FACE_OUTER_BOUND('',#1138,.T.);
#517=FACE_OUTER_BOUND('',#1139,.T.);
#518=FACE_OUTER_BOUND('',#1140,.T.);
#519=FACE_OUTER_BOUND('',#1141,.T.);
#520=FACE_OUTER_BOUND('',#1142,.T.);
#521=FACE_OUTER_BOUND('',#1143,.T.);
#522=FACE_OUTER_BOUND('',#1144,.T.);
#523=FACE_OUTER_BOUND('',#1145,.T.);
#524=FACE_OUTER_BOUND('',#1146,.T.);
#525=FACE_OUTER_BOUND('',#1147,.T.);
#526=FACE_OUTER_BOUND('',#1148,.T.);
#527=FACE_OUTER_BOUND('',#1149,.T.);
#528=FACE_OUTER_BOUND('',#1150,.T.);
#529=FACE_OUTER_BOUND('',#1151,.T.);
#530=FACE_OUTER_BOUND('',#1152,.T.);
#531=FACE_OUTER_BOUND('',#1153,.T.);
#532=FACE_OUTER_BOUND('',#1154,.T.);
#533=FACE_OUTER_BOUND('',#1155,.T.);
#534=FACE_OUTER_BOUND('',#1156,.T.);
#535=FACE_OUTER_BOUND('',#1157,.T.);
#536=FACE_OUTER_BOUND('',#1158,.T.);
#537=FACE_OUTER_BOUND('',#1159,.T.);
#538=FACE_OUTER_BOUND('',#1160,.T.);
#539=FACE_OUTER_BOUND('',#1161,.T.);
#540=FACE_OUTER_BOUND('',#1162,.T.);
#541=FACE_OUTER_BOUND('',#1163,.T.);
#542=FACE_OUTER_BOUND('',#1164,.T.);
#543=FACE_OUTER_BOUND('',#1165,.T.);
#544=FACE_OUTER_BOUND('',#1166,.T.);
#545=FACE_OUTER_BOUND('',#1167,.T.);
#546=FACE_OUTER_BOUND('',#1168,.T.);
#547=FACE_OUTER_BOUND('',#1169,.T.);
#548=FACE_OUTER_BOUND('',#1170,.T.);
#549=FACE_OUTER_BOUND('',#1171,.T.);
#550=FACE_OUTER_BOUND('',#1172,.T.);
#551=FACE_OUTER_BOUND('',#1173,.T.);
#552=FACE_OUTER_BOUND('',#1174,.T.);
#553=FACE_OUTER_BOUND('',#1175,.T.);
#554=FACE_OUTER_BOUND('',#1176,.T.);
#555=FACE_OUTER_BOUND('',#1177,.T.);
#556=FACE_OUTER_BOUND('',#1178,.T.);
#557=FACE_OUTER_BOUND('',#1179,.T.);
#558=FACE_OUTER_BOUND('',#1180,.T.);
#559=FACE_OUTER_BOUND('',#1181,.T.);
#560=FACE_OUTER_BOUND('',#1182,.T.);
#561=FACE_OUTER_BOUND('',#1183,.T.);
#562=FACE_OUTER_BOUND('',#1184,.T.);
#563=FACE_OUTER_BOUND('',#1185,.T.);
#564=FACE_OUTER_BOUND('',#1186,.T.);
#565=FACE_OUTER_BOUND('',#1187,.T.);
#566=FACE_OUTER_BOUND('',#1188,.T.);
#567=FACE_OUTER_BOUND('',#1189,.T.);
#568=FACE_OUTER_BOUND('',#1190,.T.);
#569=FACE_OUTER_BOUND('',#1191,.T.);
#570=FACE_OUTER_BOUND('',#1192,.T.);
#571=FACE_OUTER_BOUND('',#1193,.T.);
#572=FACE_OUTER_BOUND('',#1194,.T.);
#573=FACE_OUTER_BOUND('',#1195,.T.);
#574=FACE_OUTER_BOUND('',#1196,.T.);
#575=FACE_OUTER_BOUND('',#1197,.T.);
#576=FACE_OUTER_BOUND('',#1198,.T.);
#577=FACE_OUTER_BOUND('',#1199,.T.);
#578=FACE_OUTER_BOUND('',#1200,.T.);
#579=FACE_OUTER_BOUND('',#1201,.T.);
#580=FACE_OUTER_BOUND('',#1202,.T.);
#581=FACE_OUTER_BOUND('',#1203,.T.);
#582=FACE_OUTER_BOUND('',#1204,.T.);
#583=FACE_OUTER_BOUND('',#1205,.T.);
#584=FACE_OUTER_BOUND('',#1206,.T.);
#585=FACE_OUTER_BOUND('',#1207,.T.);
#586=FACE_OUTER_BOUND('',#1209,.T.);
#587=FACE_OUTER_BOUND('',#1210,.T.);
#588=FACE_OUTER_BOUND('',#1211,.T.);
#589=FACE_OUTER_BOUND('',#1213,.T.);
#590=FACE_OUTER_BOUND('',#1214,.T.);
#591=FACE_OUTER_BOUND('',#1215,.T.);
#592=FACE_OUTER_BOUND('',#1216,.T.);
#593=FACE_OUTER_BOUND('',#1217,.T.);
#594=FACE_OUTER_BOUND('',#1218,.T.);
#595=FACE_OUTER_BOUND('',#1219,.T.);
#596=FACE_OUTER_BOUND('',#1220,.T.);
#597=FACE_OUTER_BOUND('',#1221,.T.);
#598=FACE_OUTER_BOUND('',#1222,.T.);
#599=FACE_OUTER_BOUND('',#1223,.T.);
#600=FACE_OUTER_BOUND('',#1224,.T.);
#601=FACE_OUTER_BOUND('',#1225,.T.);
#602=FACE_OUTER_BOUND('',#1226,.T.);
#603=FACE_OUTER_BOUND('',#1227,.T.);
#604=FACE_OUTER_BOUND('',#1228,.T.);
#605=FACE_OUTER_BOUND('',#1229,.T.);
#606=FACE_OUTER_BOUND('',#1230,.T.);
#607=FACE_OUTER_BOUND('',#1231,.T.);
#608=FACE_OUTER_BOUND('',#1232,.T.);
#609=FACE_OUTER_BOUND('',#1233,.T.);
#610=FACE_OUTER_BOUND('',#1234,.T.);
#611=FACE_OUTER_BOUND('',#1235,.T.);
#612=FACE_OUTER_BOUND('',#1236,.T.);
#613=FACE_OUTER_BOUND('',#1237,.T.);
#614=FACE_OUTER_BOUND('',#1238,.T.);
#615=FACE_OUTER_BOUND('',#1239,.T.);
#616=FACE_OUTER_BOUND('',#1240,.T.);
#617=FACE_OUTER_BOUND('',#1241,.T.);
#618=FACE_OUTER_BOUND('',#1242,.T.);
#619=FACE_OUTER_BOUND('',#1243,.T.);
#620=FACE_OUTER_BOUND('',#1244,.T.);
#621=FACE_OUTER_BOUND('',#1246,.T.);
#622=FACE_OUTER_BOUND('',#1247,.T.);
#623=FACE_OUTER_BOUND('',#1248,.T.);
#624=FACE_OUTER_BOUND('',#1249,.T.);
#625=FACE_OUTER_BOUND('',#1251,.T.);
#626=FACE_OUTER_BOUND('',#1252,.T.);
#627=FACE_OUTER_BOUND('',#1253,.T.);
#628=FACE_OUTER_BOUND('',#1255,.T.);
#629=FACE_OUTER_BOUND('',#1259,.T.);
#630=FACE_OUTER_BOUND('',#1260,.T.);
#631=FACE_OUTER_BOUND('',#1261,.T.);
#632=FACE_OUTER_BOUND('',#1262,.T.);
#633=FACE_OUTER_BOUND('',#1263,.T.);
#634=FACE_OUTER_BOUND('',#1264,.T.);
#635=FACE_OUTER_BOUND('',#1265,.T.);
#636=FACE_OUTER_BOUND('',#1267,.T.);
#637=FACE_OUTER_BOUND('',#1268,.T.);
#638=FACE_OUTER_BOUND('',#1269,.T.);
#639=FACE_OUTER_BOUND('',#1270,.T.);
#640=FACE_OUTER_BOUND('',#1271,.T.);
#641=FACE_OUTER_BOUND('',#1273,.T.);
#642=FACE_OUTER_BOUND('',#1274,.T.);
#643=FACE_OUTER_BOUND('',#1280,.T.);
#1106=EDGE_LOOP('',(#6861,#6862,#6863,#6864,#6865,#6866,#6867,#6868));
#1107=EDGE_LOOP('',(#6869,#6870,#6871,#6872));
#1108=EDGE_LOOP('',(#6873,#6874,#6875,#6876));
#1109=EDGE_LOOP('',(#6877,#6878,#6879,#6880));
#1110=EDGE_LOOP('',(#6881,#6882,#6883,#6884));
#1111=EDGE_LOOP('',(#6885,#6886,#6887,#6888));
#1112=EDGE_LOOP('',(#6889,#6890,#6891,#6892));
#1113=EDGE_LOOP('',(#6893,#6894,#6895,#6896));
#1114=EDGE_LOOP('',(#6897,#6898,#6899,#6900));
#1115=EDGE_LOOP('',(#6901,#6902,#6903,#6904));
#1116=EDGE_LOOP('',(#6905,#6906,#6907,#6908));
#1117=EDGE_LOOP('',(#6909,#6910,#6911,#6912));
#1118=EDGE_LOOP('',(#6913,#6914,#6915,#6916));
#1119=EDGE_LOOP('',(#6917,#6918,#6919,#6920));
#1120=EDGE_LOOP('',(#6921,#6922,#6923,#6924));
#1121=EDGE_LOOP('',(#6925,#6926,#6927,#6928));
#1122=EDGE_LOOP('',(#6929,#6930,#6931,#6932));
#1123=EDGE_LOOP('',(#6933,#6934,#6935,#6936));
#1124=EDGE_LOOP('',(#6937,#6938,#6939,#6940));
#1125=EDGE_LOOP('',(#6941,#6942,#6943,#6944));
#1126=EDGE_LOOP('',(#6945,#6946,#6947,#6948));
#1127=EDGE_LOOP('',(#6949,#6950,#6951,#6952));
#1128=EDGE_LOOP('',(#6953,#6954,#6955,#6956));
#1129=EDGE_LOOP('',(#6957,#6958,#6959,#6960));
#1130=EDGE_LOOP('',(#6961,#6962,#6963,#6964));
#1131=EDGE_LOOP('',(#6965,#6966,#6967,#6968,#6969,#6970,#6971,#6972));
#1132=EDGE_LOOP('',(#6973,#6974,#6975,#6976));
#1133=EDGE_LOOP('',(#6977,#6978,#6979,#6980));
#1134=EDGE_LOOP('',(#6981,#6982,#6983,#6984));
#1135=EDGE_LOOP('',(#6985,#6986,#6987,#6988));
#1136=EDGE_LOOP('',(#6989,#6990,#6991,#6992));
#1137=EDGE_LOOP('',(#6993,#6994,#6995,#6996));
#1138=EDGE_LOOP('',(#6997,#6998,#6999,#7000));
#1139=EDGE_LOOP('',(#7001,#7002,#7003,#7004));
#1140=EDGE_LOOP('',(#7005,#7006,#7007,#7008));
#1141=EDGE_LOOP('',(#7009,#7010,#7011,#7012));
#1142=EDGE_LOOP('',(#7013,#7014,#7015,#7016));
#1143=EDGE_LOOP('',(#7017,#7018,#7019,#7020));
#1144=EDGE_LOOP('',(#7021,#7022,#7023,#7024));
#1145=EDGE_LOOP('',(#7025,#7026,#7027,#7028));
#1146=EDGE_LOOP('',(#7029,#7030,#7031,#7032));
#1147=EDGE_LOOP('',(#7033,#7034,#7035,#7036));
#1148=EDGE_LOOP('',(#7037,#7038,#7039,#7040));
#1149=EDGE_LOOP('',(#7041,#7042,#7043,#7044));
#1150=EDGE_LOOP('',(#7045,#7046,#7047,#7048));
#1151=EDGE_LOOP('',(#7049,#7050,#7051,#7052));
#1152=EDGE_LOOP('',(#7053,#7054,#7055,#7056));
#1153=EDGE_LOOP('',(#7057,#7058,#7059,#7060));
#1154=EDGE_LOOP('',(#7061,#7062,#7063,#7064));
#1155=EDGE_LOOP('',(#7065,#7066,#7067,#7068));
#1156=EDGE_LOOP('',(#7069,#7070,#7071,#7072,#7073,#7074,#7075,#7076));
#1157=EDGE_LOOP('',(#7077,#7078,#7079,#7080));
#1158=EDGE_LOOP('',(#7081,#7082,#7083,#7084));
#1159=EDGE_LOOP('',(#7085,#7086,#7087,#7088));
#1160=EDGE_LOOP('',(#7089,#7090,#7091,#7092));
#1161=EDGE_LOOP('',(#7093,#7094,#7095,#7096));
#1162=EDGE_LOOP('',(#7097,#7098,#7099,#7100));
#1163=EDGE_LOOP('',(#7101,#7102,#7103,#7104));
#1164=EDGE_LOOP('',(#7105,#7106,#7107,#7108));
#1165=EDGE_LOOP('',(#7109,#7110,#7111,#7112));
#1166=EDGE_LOOP('',(#7113,#7114,#7115,#7116));
#1167=EDGE_LOOP('',(#7117,#7118,#7119,#7120));
#1168=EDGE_LOOP('',(#7121,#7122,#7123,#7124));
#1169=EDGE_LOOP('',(#7125,#7126,#7127,#7128));
#1170=EDGE_LOOP('',(#7129,#7130,#7131,#7132));
#1171=EDGE_LOOP('',(#7133,#7134,#7135,#7136));
#1172=EDGE_LOOP('',(#7137,#7138,#7139,#7140));
#1173=EDGE_LOOP('',(#7141,#7142,#7143,#7144));
#1174=EDGE_LOOP('',(#7145,#7146,#7147,#7148));
#1175=EDGE_LOOP('',(#7149,#7150,#7151,#7152));
#1176=EDGE_LOOP('',(#7153,#7154,#7155,#7156));
#1177=EDGE_LOOP('',(#7157,#7158,#7159,#7160));
#1178=EDGE_LOOP('',(#7161,#7162,#7163,#7164));
#1179=EDGE_LOOP('',(#7165,#7166,#7167,#7168));
#1180=EDGE_LOOP('',(#7169,#7170,#7171,#7172));
#1181=EDGE_LOOP('',(#7173,#7174,#7175,#7176,#7177,#7178,#7179,#7180));
#1182=EDGE_LOOP('',(#7181,#7182,#7183,#7184));
#1183=EDGE_LOOP('',(#7185,#7186,#7187,#7188));
#1184=EDGE_LOOP('',(#7189,#7190,#7191,#7192));
#1185=EDGE_LOOP('',(#7193,#7194,#7195,#7196));
#1186=EDGE_LOOP('',(#7197,#7198,#7199,#7200));
#1187=EDGE_LOOP('',(#7201,#7202,#7203,#7204));
#1188=EDGE_LOOP('',(#7205,#7206,#7207,#7208));
#1189=EDGE_LOOP('',(#7209,#7210,#7211,#7212));
#1190=EDGE_LOOP('',(#7213,#7214,#7215,#7216));
#1191=EDGE_LOOP('',(#7217,#7218,#7219,#7220));
#1192=EDGE_LOOP('',(#7221,#7222,#7223,#7224));
#1193=EDGE_LOOP('',(#7225,#7226,#7227,#7228));
#1194=EDGE_LOOP('',(#7229,#7230,#7231,#7232));
#1195=EDGE_LOOP('',(#7233,#7234,#7235,#7236));
#1196=EDGE_LOOP('',(#7237,#7238,#7239,#7240));
#1197=EDGE_LOOP('',(#7241,#7242,#7243,#7244));
#1198=EDGE_LOOP('',(#7245,#7246,#7247,#7248));
#1199=EDGE_LOOP('',(#7249,#7250,#7251,#7252));
#1200=EDGE_LOOP('',(#7253,#7254,#7255,#7256));
#1201=EDGE_LOOP('',(#7257,#7258,#7259,#7260));
#1202=EDGE_LOOP('',(#7261,#7262,#7263,#7264));
#1203=EDGE_LOOP('',(#7265,#7266,#7267,#7268));
#1204=EDGE_LOOP('',(#7269,#7270,#7271,#7272));
#1205=EDGE_LOOP('',(#7273,#7274,#7275,#7276));
#1206=EDGE_LOOP('',(#7277,#7278,#7279,#7280));
#1207=EDGE_LOOP('',(#7281));
#1208=EDGE_LOOP('',(#7282));
#1209=EDGE_LOOP('',(#7283,#7284,#7285,#7286));
#1210=EDGE_LOOP('',(#7287,#7288,#7289,#7290));
#1211=EDGE_LOOP('',(#7291));
#1212=EDGE_LOOP('',(#7292));
#1213=EDGE_LOOP('',(#7293,#7294,#7295,#7296));
#1214=EDGE_LOOP('',(#7297,#7298,#7299,#7300));
#1215=EDGE_LOOP('',(#7301,#7302,#7303,#7304));
#1216=EDGE_LOOP('',(#7305,#7306,#7307,#7308));
#1217=EDGE_LOOP('',(#7309,#7310,#7311,#7312,#7313,#7314,#7315,#7316,#7317,
#7318,#7319,#7320,#7321,#7322,#7323,#7324,#7325,#7326,#7327,#7328,#7329,
#7330,#7331,#7332,#7333,#7334,#7335,#7336,#7337,#7338));
#1218=EDGE_LOOP('',(#7339,#7340,#7341,#7342,#7343,#7344,#7345,#7346,#7347,
#7348,#7349,#7350,#7351,#7352,#7353,#7354,#7355,#7356,#7357,#7358,#7359,
#7360,#7361,#7362,#7363,#7364,#7365,#7366,#7367));
#1219=EDGE_LOOP('',(#7368,#7369,#7370,#7371));
#1220=EDGE_LOOP('',(#7372,#7373,#7374,#7375));
#1221=EDGE_LOOP('',(#7376,#7377,#7378,#7379));
#1222=EDGE_LOOP('',(#7380,#7381,#7382,#7383,#7384,#7385,#7386,#7387,#7388,
#7389,#7390,#7391,#7392,#7393,#7394,#7395,#7396,#7397,#7398,#7399,#7400,
#7401,#7402,#7403,#7404,#7405,#7406,#7407,#7408,#7409));
#1223=EDGE_LOOP('',(#7410,#7411,#7412,#7413,#7414,#7415,#7416,#7417,#7418,
#7419,#7420,#7421,#7422,#7423,#7424,#7425,#7426,#7427,#7428,#7429,#7430,
#7431,#7432,#7433,#7434,#7435,#7436,#7437,#7438));
#1224=EDGE_LOOP('',(#7439,#7440,#7441,#7442));
#1225=EDGE_LOOP('',(#7443,#7444,#7445,#7446));
#1226=EDGE_LOOP('',(#7447,#7448,#7449,#7450));
#1227=EDGE_LOOP('',(#7451,#7452,#7453,#7454,#7455,#7456,#7457,#7458,#7459,
#7460,#7461,#7462,#7463,#7464,#7465,#7466,#7467,#7468,#7469,#7470,#7471,
#7472,#7473,#7474,#7475,#7476,#7477,#7478,#7479,#7480));
#1228=EDGE_LOOP('',(#7481,#7482,#7483,#7484,#7485,#7486,#7487,#7488,#7489,
#7490,#7491,#7492,#7493,#7494,#7495,#7496,#7497,#7498,#7499,#7500,#7501,
#7502,#7503,#7504,#7505,#7506,#7507,#7508,#7509));
#1229=EDGE_LOOP('',(#7510,#7511,#7512,#7513));
#1230=EDGE_LOOP('',(#7514,#7515,#7516,#7517));
#1231=EDGE_LOOP('',(#7518,#7519,#7520,#7521));
#1232=EDGE_LOOP('',(#7522,#7523,#7524,#7525,#7526,#7527,#7528,#7529,#7530,
#7531,#7532,#7533,#7534,#7535,#7536,#7537,#7538,#7539,#7540,#7541,#7542,
#7543,#7544,#7545,#7546,#7547,#7548,#7549,#7550,#7551));
#1233=EDGE_LOOP('',(#7552,#7553,#7554,#7555,#7556,#7557,#7558,#7559,#7560,
#7561,#7562,#7563,#7564,#7565,#7566,#7567,#7568,#7569,#7570,#7571,#7572,
#7573,#7574,#7575,#7576,#7577,#7578,#7579,#7580));
#1234=EDGE_LOOP('',(#7581,#7582,#7583,#7584));
#1235=EDGE_LOOP('',(#7585));
#1236=EDGE_LOOP('',(#7586));
#1237=EDGE_LOOP('',(#7587));
#1238=EDGE_LOOP('',(#7588));
#1239=EDGE_LOOP('',(#7589,#7590,#7591,#7592));
#1240=EDGE_LOOP('',(#7593,#7594,#7595,#7596));
#1241=EDGE_LOOP('',(#7597,#7598,#7599,#7600));
#1242=EDGE_LOOP('',(#7601,#7602,#7603,#7604));
#1243=EDGE_LOOP('',(#7605,#7606,#7607,#7608));
#1244=EDGE_LOOP('',(#7609,#7610,#7611,#7612));
#1245=EDGE_LOOP('',(#7613));
#1246=EDGE_LOOP('',(#7614,#7615,#7616,#7617));
#1247=EDGE_LOOP('',(#7618,#7619,#7620,#7621));
#1248=EDGE_LOOP('',(#7622,#7623,#7624,#7625));
#1249=EDGE_LOOP('',(#7626,#7627,#7628,#7629));
#1250=EDGE_LOOP('',(#7630));
#1251=EDGE_LOOP('',(#7631,#7632,#7633,#7634));
#1252=EDGE_LOOP('',(#7635,#7636,#7637,#7638));
#1253=EDGE_LOOP('',(#7639));
#1254=EDGE_LOOP('',(#7640));
#1255=EDGE_LOOP('',(#7641,#7642,#7643,#7644,#7645,#7646,#7647,#7648));
#1256=EDGE_LOOP('',(#7649));
#1257=EDGE_LOOP('',(#7650));
#1258=EDGE_LOOP('',(#7651));
#1259=EDGE_LOOP('',(#7652,#7653,#7654,#7655));
#1260=EDGE_LOOP('',(#7656,#7657,#7658,#7659));
#1261=EDGE_LOOP('',(#7660,#7661,#7662,#7663));
#1262=EDGE_LOOP('',(#7664,#7665,#7666,#7667));
#1263=EDGE_LOOP('',(#7668,#7669,#7670,#7671));
#1264=EDGE_LOOP('',(#7672));
#1265=EDGE_LOOP('',(#7673,#7674,#7675,#7676));
#1266=EDGE_LOOP('',(#7677));
#1267=EDGE_LOOP('',(#7678,#7679,#7680,#7681));
#1268=EDGE_LOOP('',(#7682,#7683,#7684,#7685));
#1269=EDGE_LOOP('',(#7686,#7687,#7688,#7689));
#1270=EDGE_LOOP('',(#7690,#7691,#7692,#7693,#7694,#7695,#7696,#7697));
#1271=EDGE_LOOP('',(#7698,#7699,#7700,#7701));
#1272=EDGE_LOOP('',(#7702));
#1273=EDGE_LOOP('',(#7703,#7704,#7705,#7706,#7707,#7708,#7709,#7710));
#1274=EDGE_LOOP('',(#7711,#7712,#7713,#7714));
#1275=EDGE_LOOP('',(#7715,#7716,#7717,#7718));
#1276=EDGE_LOOP('',(#7719,#7720,#7721,#7722));
#1277=EDGE_LOOP('',(#7723,#7724,#7725,#7726));
#1278=EDGE_LOOP('',(#7727,#7728,#7729,#7730));
#1279=EDGE_LOOP('',(#7731,#7732,#7733,#7734,#7735,#7736,#7737,#7738));
#1280=EDGE_LOOP('',(#7739,#7740,#7741,#7742,#7743,#7744,#7745,#7746,#7747,
#7748,#7749,#7750));
#1281=EDGE_LOOP('',(#7751));
#1282=EDGE_LOOP('',(#7752));
#1283=EDGE_LOOP('',(#7753));
#1284=EDGE_LOOP('',(#7754));
#1801=CIRCLE('',#11439,0.1666);
#1802=CIRCLE('',#11440,0.1666);
#1803=CIRCLE('',#11452,0.1666);
#1804=CIRCLE('',#11454,0.205475000000001);
#1805=CIRCLE('',#11467,0.205475000000001);
#1806=CIRCLE('',#11469,0.1666);
#1807=CIRCLE('',#11470,0.1666);
#1808=CIRCLE('',#11482,0.1666);
#1809=CIRCLE('',#11484,0.205475000000001);
#1810=CIRCLE('',#11497,0.205475000000001);
#1811=CIRCLE('',#11499,0.1666);
#1812=CIRCLE('',#11500,0.1666);
#1813=CIRCLE('',#11512,0.1666);
#1814=CIRCLE('',#11514,0.205475);
#1815=CIRCLE('',#11527,0.205475);
#1816=CIRCLE('',#11529,0.1666);
#1817=CIRCLE('',#11530,0.1666);
#1818=CIRCLE('',#11542,0.1666);
#1819=CIRCLE('',#11544,0.205475);
#1820=CIRCLE('',#11557,0.205475);
#1821=CIRCLE('',#11559,0.6);
#1822=CIRCLE('',#11560,0.6);
#1823=CIRCLE('',#11562,0.4);
#1824=CIRCLE('',#11563,0.25);
#1825=CIRCLE('',#11565,0.4);
#1826=CIRCLE('',#11567,0.25);
#1827=CIRCLE('',#11569,0.4);
#1828=CIRCLE('',#11570,0.25);
#1829=CIRCLE('',#11572,0.4);
#1830=CIRCLE('',#11574,0.25);
#1831=CIRCLE('',#11592,0.3);
#1832=CIRCLE('',#11593,0.3);
#1833=CIRCLE('',#11595,0.3);
#1834=CIRCLE('',#11596,0.3);
#1835=CIRCLE('',#11606,0.65);
#1836=CIRCLE('',#11607,0.65);
#1837=CIRCLE('',#11609,0.8);
#1838=CIRCLE('',#11610,0.8);
#1839=CIRCLE('',#11613,0.2);
#1840=CIRCLE('',#11614,0.2);
#1841=CIRCLE('',#11615,0.2);
#1842=CIRCLE('',#11616,0.2);
#1843=CIRCLE('',#11618,0.2);
#1844=CIRCLE('',#11621,0.2);
#1845=CIRCLE('',#11624,0.2);
#1846=CIRCLE('',#11628,0.2);
#1992=B_SPLINE_CURVE_WITH_KNOTS('',3,(#14568,#14569,#14570,#14571,#14572,
#14573,#14574,#14575,#14576,#14577,#14578,#14579,#14580,#14581,#14582,#14583,
#14584,#14585,#14586,#14587,#14588,#14589),.UNSPECIFIED.,.F.,.F.,(4,3,3,
3,3,3,3,4),(76.7080459413271,76.812995719686,77.8105670926689,78.8081384656519,
79.8057098386348,80.8032812116178,81.8008525846007,82.7984239575837),
 .UNSPECIFIED.);
#1993=B_SPLINE_CURVE_WITH_KNOTS('',3,(#14593,#14594,#14595,#14596,#14597,
#14598,#14599),.UNSPECIFIED.,.F.,.F.,(4,3,4),(-80.7838110923091,-79.8057098386348,
-79.2446069498473),.UNSPECIFIED.);
#1994=B_SPLINE_CURVE_WITH_KNOTS('',3,(#14603,#14604,#14605,#14606,#14607,
#14608,#14609,#14610,#14611,#14612,#14613,#14614,#14615,#14616,#14617,#14618,
#14619,#14620,#14621,#14622,#14623,#14624),.UNSPECIFIED.,.F.,.F.,(4,3,3,
3,3,3,3,4),(-79.2446069498473,-78.8081384656519,-77.8105670926689,-76.812995719686,
-75.815424346703,-74.8178529737201,-73.8202816007372,-72.9614216426678),
 .UNSPECIFIED.);
#1995=B_SPLINE_CURVE_WITH_KNOTS('',3,(#14629,#14630,#14631,#14632,#14633,
#14634,#14635,#14636,#14637,#14638,#14639,#14640,#14641,#14642,#14643,#14644,
#14645,#14646,#14647,#14648,#14649,#14650),.UNSPECIFIED.,.F.,.F.,(4,3,3,
3,3,3,3,4),(70.4248606341475,70.8275674817883,71.8251388547713,72.8227102277543,
73.8202816007372,74.8178529737201,75.815424346703,76.7080459413271),
 .UNSPECIFIED.);
#1996=B_SPLINE_CURVE_WITH_KNOTS('',3,(#14651,#14652,#14653,#14654,#14655,
#14656,#14657,#14658,#14659,#14660,#14661,#14662,#14663,#14664,#14665,#14666,
#14667,#14668,#14669,#14670,#14671,#14672,#14673,#14674,#14675),
 .UNSPECIFIED.,.F.,.F.,(4,3,3,3,3,3,3,3,4),(-72.9614216426678,-72.8227102277542,
-71.8251388547713,-70.8275674817884,-69.8299961088054,-68.8324247358225,
-67.8348533628396,-66.8372819898566,-66.6782363354882),.UNSPECIFIED.);
#1997=B_SPLINE_CURVE_WITH_KNOTS('',3,(#14680,#14681,#14682,#14683,#14684,
#14685,#14686,#14687,#14688,#14689,#14690,#14691,#14692,#14693,#14694,#14695,
#14696,#14697,#14698,#14699,#14700,#14701),.UNSPECIFIED.,.F.,.F.,(4,3,3,
3,3,3,3,4),(64.1416753269678,64.8421392438907,65.8397106168737,66.8372819898566,
67.8348533628396,68.8324247358225,69.8299961088054,70.4248606341475),
 .UNSPECIFIED.);
#1998=B_SPLINE_CURVE_WITH_KNOTS('',3,(#14702,#14703,#14704,#14705,#14706,
#14707,#14708,#14709,#14710,#14711,#14712,#14713,#14714,#14715,#14716,#14717,
#14718,#14719,#14720,#14721,#14722,#14723),.UNSPECIFIED.,.F.,.F.,(4,3,3,
3,3,3,3,4),(-66.6782363354882,-65.8397106168737,-64.8421392438908,-63.8445678709078,
-62.8469964979249,-61.849425124942,-60.851853751959,-60.3950510283085),
 .UNSPECIFIED.);
#1999=B_SPLINE_CURVE_WITH_KNOTS('',3,(#14728,#14729,#14730,#14731,#14732,
#14733,#14734,#14735,#14736,#14737,#14738,#14739,#14740,#14741,#14742,#14743,
#14744,#14745,#14746,#14747,#14748,#14749),.UNSPECIFIED.,.F.,.F.,(4,3,3,
3,3,3,3,4),(57.8584900197882,58.8567110059931,59.8542823789761,60.851853751959,
61.849425124942,62.8469964979249,63.8445678709078,64.1416753269678),
 .UNSPECIFIED.);
#2000=B_SPLINE_CURVE_WITH_KNOTS('',3,(#14750,#14751,#14752,#14753,#14754,
#14755,#14756,#14757,#14758,#14759,#14760,#14761,#14762,#14763,#14764,#14765,
#14766,#14767,#14768,#14769,#14770,#14771),.UNSPECIFIED.,.F.,.F.,(4,3,3,
3,3,3,3,4),(-60.3950510283085,-59.8542823789761,-58.8567110059932,-57.8591396330102,
-56.8615682600273,-55.8639968870443,-54.8664255140614,-54.1118657211289),
 .UNSPECIFIED.);
#2001=B_SPLINE_CURVE_WITH_KNOTS('',3,(#14776,#14777,#14778,#14779,#14780,
#14781,#14782,#14783,#14784,#14785,#14786,#14787,#14788,#14789,#14790,#14791,
#14792,#14793,#14794,#14795,#14796,#14797),.UNSPECIFIED.,.F.,.F.,(4,3,3,
3,3,3,3,4),(51.5753047126086,51.8737113951126,52.8712827680955,53.8688541410785,
54.8664255140614,55.8639968870444,56.8615682600273,57.8584900197882),
 .UNSPECIFIED.);
#2002=B_SPLINE_CURVE_WITH_KNOTS('',3,(#14798,#14799,#14800,#14801,#14802,
#14803,#14804,#14805,#14806,#14807,#14808,#14809,#14810,#14811,#14812,#14813,
#14814,#14815,#14816,#14817,#14818,#14819,#14820,#14821,#14822),
 .UNSPECIFIED.,.F.,.F.,(4,3,3,3,3,3,3,3,4),(-54.1118657211289,-53.8688541410785,
-52.8712827680955,-51.8737113951126,-50.8761400221297,-49.8785686491467,
-48.8809972761638,-47.8834259031809,-47.8286804139493),.UNSPECIFIED.);
#2003=B_SPLINE_CURVE_WITH_KNOTS('',3,(#14827,#14828,#14829,#14830,#14831,
#14832,#14833,#14834,#14835,#14836,#14837,#14838,#14839,#14840,#14841,#14842,
#14843,#14844,#14845,#14846,#14847,#14848),.UNSPECIFIED.,.F.,.F.,(4,3,3,
3,3,3,3,4),(45.2921194054291,45.888283157215,46.8858545301979,47.8834259031809,
48.8809972761638,49.8785686491467,50.8761400221297,51.5753047126086),
 .UNSPECIFIED.);
#2004=B_SPLINE_CURVE_WITH_KNOTS('',3,(#14849,#14850,#14851,#14852,#14853,
#14854,#14855,#14856,#14857,#14858,#14859,#14860,#14861,#14862,#14863,#14864,
#14865,#14866,#14867,#14868,#14869,#14870),.UNSPECIFIED.,.F.,.F.,(4,3,3,
3,3,3,3,4),(-47.8286804139493,-46.8858545301979,-45.888283157215,-44.8907117842321,
-43.8931404112491,-42.8955690382662,-41.8979976652833,-41.5454951067698),
 .UNSPECIFIED.);
#2005=B_SPLINE_CURVE_WITH_KNOTS('',3,(#14875,#14876,#14877,#14878,#14879,
#14880,#14881,#14882,#14883,#14884,#14885,#14886,#14887,#14888,#14889,#14890,
#14891,#14892,#14893,#14894,#14895,#14896),.UNSPECIFIED.,.F.,.F.,(4,3,3,
3,3,3,3,4),(39.0089340982495,39.9028549193174,40.9004262923003,41.8979976652833,
42.8955690382662,43.8931404112491,44.8907117842321,45.2921194054291),
 .UNSPECIFIED.);
#2006=B_SPLINE_CURVE_WITH_KNOTS('',3,(#14897,#14898,#14899,#14900,#14901,
#14902,#14903,#14904,#14905,#14906,#14907,#14908,#14909,#14910,#14911,#14912,
#14913,#14914,#14915,#14916,#14917,#14918),.UNSPECIFIED.,.F.,.F.,(4,3,3,
3,3,3,3,4),(-41.5454951067698,-40.9004262923003,-39.9028549193174,-38.9052835463345,
-37.9077121733515,-36.9101408003686,-35.9125694273856,-35.2623097995902),
 .UNSPECIFIED.);
#2007=B_SPLINE_CURVE_WITH_KNOTS('',3,(#14923,#14924,#14925,#14926,#14927,
#14928,#14929,#14930,#14931,#14932,#14933,#14934,#14935,#14936,#14937,#14938,
#14939,#14940,#14941,#14942,#14943,#14944,#14945,#14946,#14947),
 .UNSPECIFIED.,.F.,.F.,(4,3,3,3,3,3,3,3,4),(32.7257487910699,32.9198553084368,
33.9174266814198,34.9149980544027,35.9125694273856,36.9101408003686,37.9077121733515,
38.9052835463345,39.0089340982495),.UNSPECIFIED.);
#2008=B_SPLINE_CURVE_WITH_KNOTS('',3,(#14948,#14949,#14950,#14951,#14952,
#14953,#14954,#14955,#14956,#14957,#14958,#14959,#14960,#14961,#14962,#14963,
#14964,#14965,#14966,#14967,#14968,#14969),.UNSPECIFIED.,.F.,.F.,(4,3,3,
3,3,3,3,4),(-35.2623097995902,-34.9149980544027,-33.9174266814198,-32.9198553084368,
-31.9222839354539,-30.924712562471,-29.927141189488,-28.9791244924106),
 .UNSPECIFIED.);
#2009=B_SPLINE_CURVE_WITH_KNOTS('',3,(#14974,#14975,#14976,#14977,#14978,
#14979,#14980,#14981,#14982,#14983,#14984,#14985,#14986,#14987,#14988,#14989,
#14990,#14991,#14992,#14993,#14994,#14995),.UNSPECIFIED.,.F.,.F.,(4,3,3,
3,3,3,3,4),(26.4425634838903,26.9344270705392,27.9319984435222,28.9295698165051,
29.927141189488,30.924712562471,31.9222839354539,32.7257487910699),
 .UNSPECIFIED.);
#2010=B_SPLINE_CURVE_WITH_KNOTS('',3,(#14996,#14997,#14998,#14999,#15000,
#15001,#15002,#15003,#15004,#15005,#15006,#15007,#15008,#15009,#15010,#15011,
#15012,#15013,#15014,#15015,#15016,#15017,#15018,#15019,#15020),
 .UNSPECIFIED.,.F.,.F.,(4,3,3,3,3,3,3,3,4),(-28.9791244924106,-28.9295698165051,
-27.9319984435222,-26.9344270705392,-25.9368556975563,-24.9392843245734,
-23.9417129515904,-22.9441415786075,-22.695939185231),.UNSPECIFIED.);
#2011=B_SPLINE_CURVE_WITH_KNOTS('',3,(#15025,#15026,#15027,#15028,#15029,
#15030,#15031,#15032,#15033,#15034,#15035,#15036,#15037,#15038,#15039,#15040,
#15041,#15042,#15043,#15044,#15045,#15046),.UNSPECIFIED.,.F.,.F.,(4,3,3,
3,3,3,3,4),(20.1593781767107,20.9489988326416,21.9465702056246,22.9441415786075,
23.9417129515904,24.9392843245734,25.9368556975563,26.4425634838903),
 .UNSPECIFIED.);
#2012=B_SPLINE_CURVE_WITH_KNOTS('',3,(#15047,#15048,#15049,#15050,#15051,
#15052,#15053,#15054,#15055,#15056,#15057,#15058,#15059,#15060,#15061,#15062,
#15063,#15064,#15065,#15066,#15067,#15068),.UNSPECIFIED.,.F.,.F.,(4,3,3,
3,3,3,3,4),(-22.695939185231,-21.9465702056246,-20.9489988326416,-19.9514274596587,
-18.9538560866758,-17.9562847136928,-16.9587133407099,-16.4127538780514),
 .UNSPECIFIED.);
#2013=B_SPLINE_CURVE_WITH_KNOTS('',3,(#15073,#15074,#15075,#15076,#15077,
#15078,#15079,#15080,#15081,#15082,#15083,#15084,#15085,#15086,#15087,#15088,
#15089,#15090,#15091,#15092,#15093,#15094,#15095,#15096,#15097),
 .UNSPECIFIED.,.F.,.F.,(4,3,3,3,3,3,3,3,4),(13.8761928695311,13.9659992217611,
14.963570594744,15.961141967727,16.9587133407099,17.9562847136928,18.9538560866758,
19.9514274596587,20.1593781767107),.UNSPECIFIED.);
#2014=B_SPLINE_CURVE_WITH_KNOTS('',3,(#15098,#15099,#15100,#15101,#15102,
#15103,#15104,#15105,#15106,#15107,#15108,#15109,#15110,#15111,#15112,#15113,
#15114,#15115,#15116,#15117,#15118,#15119),.UNSPECIFIED.,.F.,.F.,(4,3,3,
3,3,3,3,4),(-16.4127538780514,-15.9611419677269,-14.963570594744,-13.9659992217611,
-12.9684278487781,-11.9708564757952,-10.9732851028123,-10.1295685708718),
 .UNSPECIFIED.);
#2015=B_SPLINE_CURVE_WITH_KNOTS('',3,(#15125,#15126,#15127,#15128,#15129,
#15130,#15131,#15132,#15133,#15134,#15135,#15136,#15137),.UNSPECIFIED.,
 .F.,.F.,(4,3,3,3,4),(-3.84638326369226,-2.9927141189488,-1.99514274596587,
-0.997571372982931,0.),.UNSPECIFIED.);
#2016=B_SPLINE_CURVE_WITH_KNOTS('',3,(#15140,#15141,#15142,#15143,#15144,
#15145,#15146,#15147,#15148,#15149,#15150,#15151,#15152,#15153,#15154,#15155,
#15156,#15157,#15158),.UNSPECIFIED.,.F.,.F.,(4,3,3,3,3,3,4),(2.01461286527457,
2.9927141189488,3.99028549193174,4.98785686491468,5.98542823789761,6.98299961088054,
7.59300756235157),.UNSPECIFIED.);
#2017=B_SPLINE_CURVE_WITH_KNOTS('',3,(#15164,#15165,#15166,#15167,#15168,
#15169,#15170),.UNSPECIFIED.,.F.,.F.,(4,1,1,1,4),(91.106186954104,91.6672898428915,
92.6648612158744,93.6624325888573,94.6600039618403),.UNSPECIFIED.);
#2018=B_SPLINE_CURVE_WITH_KNOTS('',3,(#15173,#15174,#15175,#15176,#15177,
#15178,#15179,#15180),.UNSPECIFIED.,.F.,.F.,(4,1,1,1,1,4),(91.106186954104,
91.2111367324629,92.2087081054458,93.2062794784288,94.2038508514117,95.181952105086),
 .UNSPECIFIED.);
#2019=B_SPLINE_CURVE_WITH_KNOTS('',3,(#15185,#15186,#15187,#15188,#15189,
#15190,#15191,#15192,#15193,#15194),.UNSPECIFIED.,.F.,.F.,(4,1,1,1,1,1,
1,4),(84.8230016469244,85.6818616049939,86.6794329779768,87.6770043509597,
88.6745757239427,89.6721470969256,90.6697184699085,91.106186954104),
 .UNSPECIFIED.);
#2020=B_SPLINE_CURVE_WITH_KNOTS('',3,(#15195,#15196,#15197,#15198,#15199,
#15200,#15201,#15202,#15203,#15204),.UNSPECIFIED.,.F.,.F.,(4,1,1,1,1,1,
1,4),(84.8230016469244,85.2257084945653,86.2232798675482,87.2208512405312,
88.2184226135141,89.215993986497,90.21356535948,91.106186954104),
 .UNSPECIFIED.);
#2021=B_SPLINE_CURVE_WITH_KNOTS('',3,(#15209,#15210,#15211,#15212,#15213,
#15214,#15215,#15216,#15217,#15218,#15219),.UNSPECIFIED.,.F.,.F.,(4,1,1,
1,1,1,1,1,4),(78.5398163397448,78.6988619941133,79.6964333670962,80.6940047400792,
81.6915761130621,82.689147486045,83.686718859028,84.6842902320109,84.8230016469244),
 .UNSPECIFIED.);
#2022=B_SPLINE_CURVE_WITH_KNOTS('',3,(#15220,#15221,#15222,#15223,#15224,
#15225,#15226,#15227,#15228,#15229),.UNSPECIFIED.,.F.,.F.,(4,1,1,1,1,1,
1,4),(78.5398163397448,79.2402802566677,80.2378516296506,81.2354230026336,
82.2329943756165,83.2305657485994,84.2281371215823,84.8230016469244),
 .UNSPECIFIED.);
#2023=B_SPLINE_CURVE_WITH_KNOTS('',3,(#15234,#15235,#15236,#15237,#15238,
#15239,#15240,#15241,#15242,#15243),.UNSPECIFIED.,.F.,.F.,(4,1,1,1,1,1,
1,4),(72.2566310325652,72.7134337562157,73.7110051291986,74.7085765021816,
75.7061478751645,76.7037192481474,77.7012906211304,78.5398163397448),
 .UNSPECIFIED.);
#2024=B_SPLINE_CURVE_WITH_KNOTS('',3,(#15244,#15245,#15246,#15247,#15248,
#15249,#15250,#15251,#15252,#15253,#15254),.UNSPECIFIED.,.F.,.F.,(4,1,1,
1,1,1,1,1,4),(72.2566310325652,72.2572806457871,73.2548520187701,74.252423391753,
75.2499947647359,76.2475661377189,77.2451375107018,78.2427088836847,78.5398163397448),
 .UNSPECIFIED.);
#2025=B_SPLINE_CURVE_WITH_KNOTS('',3,(#15259,#15260,#15261,#15262,#15263,
#15264,#15265,#15266,#15267,#15268),.UNSPECIFIED.,.F.,.F.,(4,1,1,1,1,1,
1,4),(65.9734457253856,66.7280055183181,67.725576891301,68.723148264284,
69.7207196372669,70.7182910102498,71.7158623832328,72.2566310325652),
 .UNSPECIFIED.);
#2026=B_SPLINE_CURVE_WITH_KNOTS('',3,(#15269,#15270,#15271,#15272,#15273,
#15274,#15275,#15276,#15277,#15278),.UNSPECIFIED.,.F.,.F.,(4,1,1,1,1,1,
1,4),(65.9734457253856,66.2718524078895,67.2694237808725,68.2669951538554,
69.2645665268383,70.2621378998213,71.2597092728042,72.2566310325652),
 .UNSPECIFIED.);
#2027=B_SPLINE_CURVE_WITH_KNOTS('',3,(#15283,#15284,#15285,#15286,#15287,
#15288,#15289,#15290,#15291,#15292,#15293),.UNSPECIFIED.,.F.,.F.,(4,1,1,
1,1,1,1,1,4),(59.690260418206,59.7450059074375,60.7425772804205,61.7401486534034,
62.7377200263864,63.7352913993693,64.7328627723522,65.7304341453352,65.9734457253856),
 .UNSPECIFIED.);
#2028=B_SPLINE_CURVE_WITH_KNOTS('',3,(#15294,#15295,#15296,#15297,#15298,
#15299,#15300,#15301,#15302,#15303),.UNSPECIFIED.,.F.,.F.,(4,1,1,1,1,1,
1,4),(59.690260418206,60.2864241699919,61.2839955429748,62.2815669159578,
63.2791382889407,64.2767096619237,65.2742810349066,65.9734457253856),
 .UNSPECIFIED.);
#2029=B_SPLINE_CURVE_WITH_KNOTS('',3,(#15308,#15309,#15310,#15311,#15312,
#15313,#15314,#15315,#15316,#15317),.UNSPECIFIED.,.F.,.F.,(4,1,1,1,1,1,
1,4),(53.4070751110264,53.7595776695399,54.7571490425229,55.7547204155058,
56.7522917884887,57.7498631614717,58.7474345344546,59.690260418206),
 .UNSPECIFIED.);
#2030=B_SPLINE_CURVE_WITH_KNOTS('',3,(#15318,#15319,#15320,#15321,#15322,
#15323,#15324,#15325,#15326,#15327),.UNSPECIFIED.,.F.,.F.,(4,1,1,1,1,1,
1,4),(53.4070751110264,54.3009959320943,55.2985673050772,56.2961386780602,
57.2937100510431,58.291281424026,59.288852797009,59.690260418206),
 .UNSPECIFIED.);
#2031=B_SPLINE_CURVE_WITH_KNOTS('',3,(#15332,#15333,#15334,#15335,#15336,
#15337,#15338,#15339,#15340,#15341),.UNSPECIFIED.,.F.,.F.,(4,1,1,1,1,1,
1,4),(47.1238898038469,47.7741494316423,48.7717208046253,49.7692921776082,
50.7668635505911,51.7644349235741,52.762006296557,53.4070751110264),
 .UNSPECIFIED.);
#2032=B_SPLINE_CURVE_WITH_KNOTS('',3,(#15342,#15343,#15344,#15345,#15346,
#15347,#15348,#15349,#15350,#15351,#15352),.UNSPECIFIED.,.F.,.F.,(4,1,1,
1,1,1,1,1,4),(47.1238898038469,47.3179963212138,48.3155676941967,49.3131390671796,
50.3107104401626,51.3082818131455,52.3058531861284,53.3034245591114,53.4070751110264),
 .UNSPECIFIED.);
#2033=B_SPLINE_CURVE_WITH_KNOTS('',3,(#15357,#15358,#15359,#15360,#15361,
#15362,#15363,#15364,#15365,#15366),.UNSPECIFIED.,.F.,.F.,(4,1,1,1,1,1,
1,4),(40.8407044966673,41.7887211937447,42.7862925667277,43.7838639397106,
44.7814353126935,45.7790066856765,46.7765780586594,47.1238898038469),
 .UNSPECIFIED.);
#2034=B_SPLINE_CURVE_WITH_KNOTS('',3,(#15367,#15368,#15369,#15370,#15371,
#15372,#15373,#15374,#15375,#15376),.UNSPECIFIED.,.F.,.F.,(4,1,1,1,1,1,
1,4),(40.8407044966673,41.3325680833162,42.3301394562991,43.327710829282,
44.325282202265,45.3228535752479,46.3204249482308,47.1238898038469),
 .UNSPECIFIED.);
#2035=B_SPLINE_CURVE_WITH_KNOTS('',3,(#15381,#15382,#15383,#15384,#15385,
#15386,#15387,#15388,#15389,#15390,#15391),.UNSPECIFIED.,.F.,.F.,(4,1,1,
1,1,1,1,1,4),(34.5575191894876,34.8057215828642,35.8032929558471,36.80086432883,
37.798435701813,38.7960070747959,39.7935784477789,40.7911498207618,40.8407044966673),
 .UNSPECIFIED.);
#2036=B_SPLINE_CURVE_WITH_KNOTS('',3,(#15392,#15393,#15394,#15395,#15396,
#15397,#15398,#15399,#15400,#15401),.UNSPECIFIED.,.F.,.F.,(4,1,1,1,1,1,
1,4),(34.5575191894876,35.3471398454185,36.3447112184015,37.3422825913844,
38.3398539643674,39.3374253373503,40.3349967103332,40.8407044966673),
 .UNSPECIFIED.);
#2037=B_SPLINE_CURVE_WITH_KNOTS('',3,(#15406,#15407,#15408,#15409,#15410,
#15411,#15412,#15413,#15414,#15415),.UNSPECIFIED.,.F.,.F.,(4,1,1,1,1,1,
1,4),(28.2743338823081,28.8202933449666,29.8178647179495,30.8154360909324,
31.8130074639154,32.8105788368983,33.8081502098812,34.5575191894876),
 .UNSPECIFIED.);
#2038=B_SPLINE_CURVE_WITH_KNOTS('',3,(#15416,#15417,#15418,#15419,#15420,
#15421,#15422,#15423,#15424,#15425,#15426),.UNSPECIFIED.,.F.,.F.,(4,1,1,
1,1,1,1,1,4),(28.2743338823081,28.364140234538,29.3617116075209,30.3592829805039,
31.3568543534868,32.3544257264697,33.3519970994527,34.3495684724356,34.5575191894876),
 .UNSPECIFIED.);
#2039=B_SPLINE_CURVE_WITH_KNOTS('',3,(#15431,#15432,#15433,#15434,#15435,
#15436,#15437,#15438,#15439,#15440),.UNSPECIFIED.,.F.,.F.,(4,1,1,1,1,1,
1,4),(21.9911485751285,22.834865107069,23.8324364800519,24.8300078530348,
25.8275792260178,26.8251505990007,27.8227219719836,28.2743338823081),
 .UNSPECIFIED.);
#2040=B_SPLINE_CURVE_WITH_KNOTS('',3,(#15441,#15442,#15443,#15444,#15445,
#15446,#15447,#15448,#15449,#15450),.UNSPECIFIED.,.F.,.F.,(4,1,1,1,1,1,
1,4),(21.9911485751285,22.3787119966404,23.3762833696233,24.3738547426063,
25.3714261155892,26.3689974885721,27.3665688615551,28.2743338823081),
 .UNSPECIFIED.);
#2041=B_SPLINE_CURVE_WITH_KNOTS('',3,(#15456,#15457,#15458,#15459,#15460),
 .UNSPECIFIED.,.F.,.F.,(4,1,4),(14.3981410127769,15.3957123857599,15.7079632679489),
 .UNSPECIFIED.);
#2042=B_SPLINE_CURVE_WITH_KNOTS('',3,(#15463,#15464,#15465,#15466,#15467),
 .UNSPECIFIED.,.F.,.F.,(4,1,4),(13.8761928695312,14.8542941232055,15.7079632679489),
 .UNSPECIFIED.);
#2043=B_SPLINE_CURVE_WITH_KNOTS('',3,(#15473,#15474,#15475,#15476,#15477,
#15478,#15479,#15480,#15481,#15482,#15483,#15484,#15485,#15486,#15487,#15488,
#15489,#15490,#15491,#15492,#15493,#15494),.UNSPECIFIED.,.F.,.F.,(4,3,3,
3,3,3,3,4),(76.7080459413271,76.8129957196859,77.8105670926688,78.8081384656517,
79.8057098386347,80.8032812116176,81.8008525846006,82.7984239575835),
 .UNSPECIFIED.);
#2044=B_SPLINE_CURVE_WITH_KNOTS('',3,(#15498,#15499,#15500,#15501,#15502,
#15503,#15504),.UNSPECIFIED.,.F.,.F.,(4,3,4),(-80.783811092309,-79.8057098386347,
-79.2446069498473),.UNSPECIFIED.);
#2045=B_SPLINE_CURVE_WITH_KNOTS('',3,(#15508,#15509,#15510,#15511,#15512,
#15513,#15514,#15515,#15516,#15517,#15518,#15519,#15520,#15521,#15522,#15523,
#15524,#15525,#15526,#15527,#15528,#15529),.UNSPECIFIED.,.F.,.F.,(4,3,3,
3,3,3,3,4),(-79.2446069498473,-78.8081384656518,-77.8105670926688,-76.8129957196859,
-75.815424346703,-74.81785297372,-73.8202816007371,-72.9614216426678),
 .UNSPECIFIED.);
#2046=B_SPLINE_CURVE_WITH_KNOTS('',3,(#15534,#15535,#15536,#15537,#15538,
#15539,#15540,#15541,#15542,#15543,#15544,#15545,#15546,#15547,#15548,#15549,
#15550,#15551,#15552,#15553,#15554,#15555),.UNSPECIFIED.,.F.,.F.,(4,3,3,
3,3,3,3,4),(70.4248606341475,70.8275674817883,71.8251388547712,72.8227102277542,
73.8202816007371,74.81785297372,75.815424346703,76.7080459413271),
 .UNSPECIFIED.);
#2047=B_SPLINE_CURVE_WITH_KNOTS('',3,(#15556,#15557,#15558,#15559,#15560,
#15561,#15562,#15563,#15564,#15565,#15566,#15567,#15568,#15569,#15570,#15571,
#15572,#15573,#15574,#15575,#15576,#15577,#15578,#15579,#15580),
 .UNSPECIFIED.,.F.,.F.,(4,3,3,3,3,3,3,3,4),(-72.9614216426678,-72.8227102277542,
-71.8251388547712,-70.8275674817883,-69.8299961088054,-68.8324247358224,
-67.8348533628395,-66.8372819898566,-66.6782363354882),.UNSPECIFIED.);
#2048=B_SPLINE_CURVE_WITH_KNOTS('',3,(#15585,#15586,#15587,#15588,#15589,
#15590,#15591,#15592,#15593,#15594,#15595,#15596,#15597,#15598,#15599,#15600,
#15601,#15602,#15603,#15604,#15605,#15606),.UNSPECIFIED.,.F.,.F.,(4,3,3,
3,3,3,3,4),(64.1416753269678,64.8421392438907,65.8397106168736,66.8372819898565,
67.8348533628395,68.8324247358224,69.8299961088054,70.4248606341475),
 .UNSPECIFIED.);
#2049=B_SPLINE_CURVE_WITH_KNOTS('',3,(#15607,#15608,#15609,#15610,#15611,
#15612,#15613,#15614,#15615,#15616,#15617,#15618,#15619,#15620,#15621,#15622,
#15623,#15624,#15625,#15626,#15627,#15628),.UNSPECIFIED.,.F.,.F.,(4,3,3,
3,3,3,3,4),(-66.6782363354882,-65.8397106168736,-64.8421392438907,-63.8445678709078,
-62.8469964979248,-61.8494251249419,-60.851853751959,-60.3950510283085),
 .UNSPECIFIED.);
#2050=B_SPLINE_CURVE_WITH_KNOTS('',3,(#15633,#15634,#15635,#15636,#15637,
#15638,#15639,#15640,#15641,#15642,#15643,#15644,#15645,#15646,#15647,#15648,
#15649,#15650,#15651,#15652,#15653,#15654),.UNSPECIFIED.,.F.,.F.,(4,3,3,
3,3,3,3,4),(57.8584900197882,58.8567110059931,59.854282378976,60.851853751959,
61.8494251249419,62.8469964979248,63.8445678709078,64.1416753269678),
 .UNSPECIFIED.);
#2051=B_SPLINE_CURVE_WITH_KNOTS('',3,(#15655,#15656,#15657,#15658,#15659,
#15660,#15661,#15662,#15663,#15664,#15665,#15666,#15667,#15668,#15669,#15670,
#15671,#15672,#15673,#15674,#15675,#15676),.UNSPECIFIED.,.F.,.F.,(4,3,3,
3,3,3,3,4),(-60.3950510283085,-59.854282378976,-58.8567110059931,-57.8591396330102,
-56.8615682600272,-55.8639968870443,-54.8664255140614,-54.1118657211289),
 .UNSPECIFIED.);
#2052=B_SPLINE_CURVE_WITH_KNOTS('',3,(#15681,#15682,#15683,#15684,#15685,
#15686,#15687,#15688,#15689,#15690,#15691,#15692,#15693,#15694,#15695,#15696,
#15697,#15698,#15699,#15700,#15701,#15702),.UNSPECIFIED.,.F.,.F.,(4,3,3,
3,3,3,3,4),(51.5753047126086,51.8737113951126,52.8712827680955,53.8688541410784,
54.8664255140613,55.8639968870443,56.8615682600272,57.8584900197882),
 .UNSPECIFIED.);
#2053=B_SPLINE_CURVE_WITH_KNOTS('',3,(#15703,#15704,#15705,#15706,#15707,
#15708,#15709,#15710,#15711,#15712,#15713,#15714,#15715,#15716,#15717,#15718,
#15719,#15720,#15721,#15722,#15723,#15724,#15725,#15726,#15727),
 .UNSPECIFIED.,.F.,.F.,(4,3,3,3,3,3,3,3,4),(-54.1118657211289,-53.8688541410784,
-52.8712827680955,-51.8737113951126,-50.8761400221296,-49.8785686491467,
-48.8809972761638,-47.8834259031808,-47.8286804139494),.UNSPECIFIED.);
#2054=B_SPLINE_CURVE_WITH_KNOTS('',3,(#15732,#15733,#15734,#15735,#15736,
#15737,#15738,#15739,#15740,#15741,#15742,#15743,#15744,#15745,#15746,#15747,
#15748,#15749,#15750,#15751,#15752,#15753),.UNSPECIFIED.,.F.,.F.,(4,3,3,
3,3,3,3,4),(45.2921194054291,45.8882831572149,46.8858545301979,47.8834259031808,
48.8809972761637,49.8785686491467,50.8761400221296,51.5753047126086),
 .UNSPECIFIED.);
#2055=B_SPLINE_CURVE_WITH_KNOTS('',3,(#15754,#15755,#15756,#15757,#15758,
#15759,#15760,#15761,#15762,#15763,#15764,#15765,#15766,#15767,#15768,#15769,
#15770,#15771,#15772,#15773,#15774,#15775),.UNSPECIFIED.,.F.,.F.,(4,3,3,
3,3,3,3,4),(-47.8286804139494,-46.8858545301979,-45.888283157215,-44.890711784232,
-43.8931404112491,-42.8955690382662,-41.8979976652832,-41.5454951067698),
 .UNSPECIFIED.);
#2056=B_SPLINE_CURVE_WITH_KNOTS('',3,(#15780,#15781,#15782,#15783,#15784,
#15785,#15786,#15787,#15788,#15789,#15790,#15791,#15792,#15793,#15794,#15795,
#15796,#15797,#15798,#15799,#15800,#15801),.UNSPECIFIED.,.F.,.F.,(4,3,3,
3,3,3,3,4),(39.0089340982495,39.9028549193173,40.9004262923003,41.8979976652832,
42.8955690382661,43.8931404112491,44.890711784232,45.2921194054291),
 .UNSPECIFIED.);
#2057=B_SPLINE_CURVE_WITH_KNOTS('',3,(#15802,#15803,#15804,#15805,#15806,
#15807,#15808,#15809,#15810,#15811,#15812,#15813,#15814,#15815,#15816,#15817,
#15818,#15819,#15820,#15821,#15822,#15823),.UNSPECIFIED.,.F.,.F.,(4,3,3,
3,3,3,3,4),(-41.5454951067698,-40.9004262923003,-39.9028549193174,-38.9052835463344,
-37.9077121733515,-36.9101408003686,-35.9125694273856,-35.2623097995902),
 .UNSPECIFIED.);
#2058=B_SPLINE_CURVE_WITH_KNOTS('',3,(#15828,#15829,#15830,#15831,#15832,
#15833,#15834,#15835,#15836,#15837,#15838,#15839,#15840,#15841,#15842,#15843,
#15844,#15845,#15846,#15847,#15848,#15849,#15850,#15851,#15852),
 .UNSPECIFIED.,.F.,.F.,(4,3,3,3,3,3,3,3,4),(32.7257487910699,32.9198553084368,
33.9174266814197,34.9149980544027,35.9125694273856,36.9101408003685,37.9077121733515,
38.9052835463344,39.0089340982495),.UNSPECIFIED.);
#2059=B_SPLINE_CURVE_WITH_KNOTS('',3,(#15853,#15854,#15855,#15856,#15857,
#15858,#15859,#15860,#15861,#15862,#15863,#15864,#15865,#15866,#15867,#15868,
#15869,#15870,#15871,#15872,#15873,#15874),.UNSPECIFIED.,.F.,.F.,(4,3,3,
3,3,3,3,4),(-35.2623097995902,-34.9149980544027,-33.9174266814198,-32.9198553084368,
-31.9222839354539,-30.924712562471,-29.927141189488,-28.9791244924106),
 .UNSPECIFIED.);
#2060=B_SPLINE_CURVE_WITH_KNOTS('',3,(#15879,#15880,#15881,#15882,#15883,
#15884,#15885,#15886,#15887,#15888,#15889,#15890,#15891,#15892,#15893,#15894,
#15895,#15896,#15897,#15898,#15899,#15900),.UNSPECIFIED.,.F.,.F.,(4,3,3,
3,3,3,3,4),(26.4425634838903,26.9344270705392,27.9319984435221,28.9295698165051,
29.927141189488,30.9247125624709,31.9222839354539,32.7257487910699),
 .UNSPECIFIED.);
#2061=B_SPLINE_CURVE_WITH_KNOTS('',3,(#15901,#15902,#15903,#15904,#15905,
#15906,#15907,#15908,#15909,#15910,#15911,#15912,#15913,#15914,#15915,#15916,
#15917,#15918,#15919,#15920,#15921,#15922,#15923,#15924,#15925),
 .UNSPECIFIED.,.F.,.F.,(4,3,3,3,3,3,3,3,4),(-28.9791244924106,-28.9295698165051,
-27.9319984435222,-26.9344270705392,-25.9368556975563,-24.9392843245733,
-23.9417129515904,-22.9441415786075,-22.695939185231),.UNSPECIFIED.);
#2062=B_SPLINE_CURVE_WITH_KNOTS('',3,(#15930,#15931,#15932,#15933,#15934,
#15935,#15936,#15937,#15938,#15939,#15940,#15941,#15942,#15943,#15944,#15945,
#15946,#15947,#15948,#15949,#15950,#15951),.UNSPECIFIED.,.F.,.F.,(4,3,3,
3,3,3,3,4),(20.1593781767107,20.9489988326416,21.9465702056245,22.9441415786075,
23.9417129515904,24.9392843245733,25.9368556975563,26.4425634838903),
 .UNSPECIFIED.);
#2063=B_SPLINE_CURVE_WITH_KNOTS('',3,(#15952,#15953,#15954,#15955,#15956,
#15957,#15958,#15959,#15960,#15961,#15962,#15963,#15964,#15965,#15966,#15967,
#15968,#15969,#15970,#15971,#15972,#15973),.UNSPECIFIED.,.F.,.F.,(4,3,3,
3,3,3,3,4),(-22.695939185231,-21.9465702056245,-20.9489988326416,-19.9514274596587,
-18.9538560866757,-17.9562847136928,-16.9587133407099,-16.4127538780514),
 .UNSPECIFIED.);
#2064=B_SPLINE_CURVE_WITH_KNOTS('',3,(#15978,#15979,#15980,#15981,#15982,
#15983,#15984,#15985,#15986,#15987,#15988,#15989,#15990,#15991,#15992,#15993,
#15994,#15995,#15996,#15997,#15998,#15999,#16000,#16001,#16002),
 .UNSPECIFIED.,.F.,.F.,(4,3,3,3,3,3,3,3,4),(13.8761928695311,13.9659992217611,
14.963570594744,15.9611419677269,16.9587133407099,17.9562847136928,18.9538560866757,
19.9514274596587,20.1593781767107),.UNSPECIFIED.);
#2065=B_SPLINE_CURVE_WITH_KNOTS('',3,(#16003,#16004,#16005,#16006,#16007,
#16008,#16009,#16010,#16011,#16012,#16013,#16014,#16015,#16016,#16017,#16018,
#16019,#16020,#16021,#16022,#16023,#16024),.UNSPECIFIED.,.F.,.F.,(4,3,3,
3,3,3,3,4),(-16.4127538780514,-15.9611419677269,-14.963570594744,-13.9659992217611,
-12.9684278487781,-11.9708564757952,-10.9732851028123,-10.1295685708718),
 .UNSPECIFIED.);
#2066=B_SPLINE_CURVE_WITH_KNOTS('',3,(#16030,#16031,#16032,#16033,#16034,
#16035,#16036,#16037,#16038,#16039,#16040,#16041,#16042),.UNSPECIFIED.,
 .F.,.F.,(4,3,3,3,4),(-3.84638326369226,-2.9927141189488,-1.99514274596587,
-0.997571372982934,0.),.UNSPECIFIED.);
#2067=B_SPLINE_CURVE_WITH_KNOTS('',3,(#16045,#16046,#16047,#16048,#16049,
#16050,#16051,#16052,#16053,#16054,#16055,#16056,#16057,#16058,#16059,#16060,
#16061,#16062,#16063),.UNSPECIFIED.,.F.,.F.,(4,3,3,3,3,3,4),(2.01461286527457,
2.9927141189488,3.99028549193173,4.98785686491467,5.9854282378976,6.98299961088054,
7.59300756235157),.UNSPECIFIED.);
#2068=B_SPLINE_CURVE_WITH_KNOTS('',3,(#16069,#16070,#16071,#16072,#16073,
#16074,#16075),.UNSPECIFIED.,.F.,.F.,(4,1,1,1,4),(91.106186954104,91.6672898428914,
92.6648612158743,93.6624325888573,94.6600039618402),.UNSPECIFIED.);
#2069=B_SPLINE_CURVE_WITH_KNOTS('',3,(#16078,#16079,#16080,#16081,#16082,
#16083,#16084,#16085),.UNSPECIFIED.,.F.,.F.,(4,1,1,1,1,4),(91.106186954104,
91.2111367324628,92.2087081054457,93.2062794784287,94.2038508514116,95.1819521050859),
 .UNSPECIFIED.);
#2070=B_SPLINE_CURVE_WITH_KNOTS('',3,(#16090,#16091,#16092,#16093,#16094,
#16095,#16096,#16097,#16098,#16099),.UNSPECIFIED.,.F.,.F.,(4,1,1,1,1,1,
1,4),(84.8230016469244,85.6818616049938,86.6794329779767,87.6770043509596,
88.6745757239426,89.6721470969255,90.6697184699085,91.106186954104),
 .UNSPECIFIED.);
#2071=B_SPLINE_CURVE_WITH_KNOTS('',3,(#16100,#16101,#16102,#16103,#16104,
#16105,#16106,#16107,#16108,#16109),.UNSPECIFIED.,.F.,.F.,(4,1,1,1,1,1,
1,4),(84.8230016469244,85.2257084945652,86.2232798675481,87.2208512405311,
88.218422613514,89.2159939864969,90.2135653594799,91.106186954104),
 .UNSPECIFIED.);
#2072=B_SPLINE_CURVE_WITH_KNOTS('',3,(#16114,#16115,#16116,#16117,#16118,
#16119,#16120,#16121,#16122,#16123,#16124),.UNSPECIFIED.,.F.,.F.,(4,1,1,
1,1,1,1,1,4),(78.5398163397448,78.6988619941132,79.6964333670962,80.6940047400791,
81.6915761130621,82.689147486045,83.6867188590279,84.6842902320109,84.8230016469244),
 .UNSPECIFIED.);
#2073=B_SPLINE_CURVE_WITH_KNOTS('',3,(#16125,#16126,#16127,#16128,#16129,
#16130,#16131,#16132,#16133,#16134),.UNSPECIFIED.,.F.,.F.,(4,1,1,1,1,1,
1,4),(78.5398163397448,79.2402802566676,80.2378516296505,81.2354230026335,
82.2329943756164,83.2305657485993,84.2281371215823,84.8230016469244),
 .UNSPECIFIED.);
#2074=B_SPLINE_CURVE_WITH_KNOTS('',3,(#16139,#16140,#16141,#16142,#16143,
#16144,#16145,#16146,#16147,#16148),.UNSPECIFIED.,.F.,.F.,(4,1,1,1,1,1,
1,4),(72.2566310325652,72.7134337562156,73.7110051291986,74.7085765021815,
75.7061478751644,76.7037192481474,77.7012906211303,78.5398163397448),
 .UNSPECIFIED.);
#2075=B_SPLINE_CURVE_WITH_KNOTS('',3,(#16149,#16150,#16151,#16152,#16153,
#16154,#16155,#16156,#16157,#16158,#16159),.UNSPECIFIED.,.F.,.F.,(4,1,1,
1,1,1,1,1,4),(72.2566310325652,72.2572806457871,73.25485201877,74.2524233917529,
75.2499947647359,76.2475661377188,77.2451375107017,78.2427088836847,78.5398163397448),
 .UNSPECIFIED.);
#2076=B_SPLINE_CURVE_WITH_KNOTS('',3,(#16164,#16165,#16166,#16167,#16168,
#16169,#16170,#16171,#16172,#16173),.UNSPECIFIED.,.F.,.F.,(4,1,1,1,1,1,
1,4),(65.9734457253856,66.728005518318,67.725576891301,68.7231482642839,
69.7207196372668,70.7182910102498,71.7158623832327,72.2566310325652),
 .UNSPECIFIED.);
#2077=B_SPLINE_CURVE_WITH_KNOTS('',3,(#16174,#16175,#16176,#16177,#16178,
#16179,#16180,#16181,#16182,#16183),.UNSPECIFIED.,.F.,.F.,(4,1,1,1,1,1,
1,4),(65.9734457253856,66.2718524078895,67.2694237808724,68.2669951538553,
69.2645665268383,70.2621378998212,71.2597092728041,72.2566310325652),
 .UNSPECIFIED.);
#2078=B_SPLINE_CURVE_WITH_KNOTS('',3,(#16188,#16189,#16190,#16191,#16192,
#16193,#16194,#16195,#16196,#16197,#16198),.UNSPECIFIED.,.F.,.F.,(4,1,1,
1,1,1,1,1,4),(59.690260418206,59.7450059074375,60.7425772804204,61.7401486534034,
62.7377200263863,63.7352913993692,64.7328627723522,65.7304341453351,65.9734457253856),
 .UNSPECIFIED.);
#2079=B_SPLINE_CURVE_WITH_KNOTS('',3,(#16199,#16200,#16201,#16202,#16203,
#16204,#16205,#16206,#16207,#16208),.UNSPECIFIED.,.F.,.F.,(4,1,1,1,1,1,
1,4),(59.690260418206,60.2864241699919,61.2839955429748,62.2815669159577,
63.2791382889407,64.2767096619236,65.2742810349065,65.9734457253856),
 .UNSPECIFIED.);
#2080=B_SPLINE_CURVE_WITH_KNOTS('',3,(#16213,#16214,#16215,#16216,#16217,
#16218,#16219,#16220,#16221,#16222),.UNSPECIFIED.,.F.,.F.,(4,1,1,1,1,1,
1,4),(53.4070751110264,53.7595776695399,54.7571490425228,55.7547204155058,
56.7522917884887,57.7498631614716,58.7474345344546,59.690260418206),
 .UNSPECIFIED.);
#2081=B_SPLINE_CURVE_WITH_KNOTS('',3,(#16223,#16224,#16225,#16226,#16227,
#16228,#16229,#16230,#16231,#16232),.UNSPECIFIED.,.F.,.F.,(4,1,1,1,1,1,
1,4),(53.4070751110264,54.3009959320943,55.2985673050772,56.2961386780601,
57.2937100510431,58.291281424026,59.2888527970089,59.690260418206),
 .UNSPECIFIED.);
#2082=B_SPLINE_CURVE_WITH_KNOTS('',3,(#16237,#16238,#16239,#16240,#16241,
#16242,#16243,#16244,#16245,#16246),.UNSPECIFIED.,.F.,.F.,(4,1,1,1,1,1,
1,4),(47.1238898038469,47.7741494316423,48.7717208046252,49.7692921776082,
50.7668635505911,51.764434923574,52.762006296557,53.4070751110264),
 .UNSPECIFIED.);
#2083=B_SPLINE_CURVE_WITH_KNOTS('',3,(#16247,#16248,#16249,#16250,#16251,
#16252,#16253,#16254,#16255,#16256,#16257),.UNSPECIFIED.,.F.,.F.,(4,1,1,
1,1,1,1,1,4),(47.1238898038469,47.3179963212137,48.3155676941967,49.3131390671796,
50.3107104401625,51.3082818131455,52.3058531861284,53.3034245591113,53.4070751110264),
 .UNSPECIFIED.);
#2084=B_SPLINE_CURVE_WITH_KNOTS('',3,(#16262,#16263,#16264,#16265,#16266,
#16267,#16268,#16269,#16270,#16271),.UNSPECIFIED.,.F.,.F.,(4,1,1,1,1,1,
1,4),(40.8407044966673,41.7887211937447,42.7862925667276,43.7838639397106,
44.7814353126935,45.7790066856764,46.7765780586594,47.1238898038469),
 .UNSPECIFIED.);
#2085=B_SPLINE_CURVE_WITH_KNOTS('',3,(#16272,#16273,#16274,#16275,#16276,
#16277,#16278,#16279,#16280,#16281),.UNSPECIFIED.,.F.,.F.,(4,1,1,1,1,1,
1,4),(40.8407044966673,41.3325680833161,42.3301394562991,43.327710829282,
44.3252822022649,45.3228535752479,46.3204249482308,47.1238898038469),
 .UNSPECIFIED.);
#2086=B_SPLINE_CURVE_WITH_KNOTS('',3,(#16286,#16287,#16288,#16289,#16290,
#16291,#16292,#16293,#16294,#16295,#16296),.UNSPECIFIED.,.F.,.F.,(4,1,1,
1,1,1,1,1,4),(34.5575191894876,34.8057215828642,35.8032929558471,36.80086432883,
37.798435701813,38.7960070747959,39.7935784477788,40.7911498207618,40.8407044966673),
 .UNSPECIFIED.);
#2087=B_SPLINE_CURVE_WITH_KNOTS('',3,(#16297,#16298,#16299,#16300,#16301,
#16302,#16303,#16304,#16305,#16306),.UNSPECIFIED.,.F.,.F.,(4,1,1,1,1,1,
1,4),(34.5575191894876,35.3471398454185,36.3447112184015,37.3422825913844,
38.3398539643673,39.3374253373503,40.3349967103332,40.8407044966673),
 .UNSPECIFIED.);
#2088=B_SPLINE_CURVE_WITH_KNOTS('',3,(#16311,#16312,#16313,#16314,#16315,
#16316,#16317,#16318,#16319,#16320),.UNSPECIFIED.,.F.,.F.,(4,1,1,1,1,1,
1,4),(28.2743338823081,28.8202933449666,29.8178647179495,30.8154360909324,
31.8130074639154,32.8105788368983,33.8081502098812,34.5575191894876),
 .UNSPECIFIED.);
#2089=B_SPLINE_CURVE_WITH_KNOTS('',3,(#16321,#16322,#16323,#16324,#16325,
#16326,#16327,#16328,#16329,#16330,#16331),.UNSPECIFIED.,.F.,.F.,(4,1,1,
1,1,1,1,1,4),(28.2743338823081,28.364140234538,29.3617116075209,30.3592829805039,
31.3568543534868,32.3544257264697,33.3519970994527,34.3495684724356,34.5575191894876),
 .UNSPECIFIED.);
#2090=B_SPLINE_CURVE_WITH_KNOTS('',3,(#16336,#16337,#16338,#16339,#16340,
#16341,#16342,#16343,#16344,#16345),.UNSPECIFIED.,.F.,.F.,(4,1,1,1,1,1,
1,4),(21.9911485751285,22.8348651070689,23.8324364800519,24.8300078530348,
25.8275792260178,26.8251505990007,27.8227219719836,28.2743338823081),
 .UNSPECIFIED.);
#2091=B_SPLINE_CURVE_WITH_KNOTS('',3,(#16346,#16347,#16348,#16349,#16350,
#16351,#16352,#16353,#16354,#16355),.UNSPECIFIED.,.F.,.F.,(4,1,1,1,1,1,
1,4),(21.9911485751285,22.3787119966404,23.3762833696233,24.3738547426063,
25.3714261155892,26.3689974885721,27.3665688615551,28.2743338823081),
 .UNSPECIFIED.);
#2092=B_SPLINE_CURVE_WITH_KNOTS('',3,(#16361,#16362,#16363,#16364,#16365),
 .UNSPECIFIED.,.F.,.F.,(4,1,4),(14.3981410127769,15.3957123857599,15.7079632679489),
 .UNSPECIFIED.);
#2093=B_SPLINE_CURVE_WITH_KNOTS('',3,(#16368,#16369,#16370,#16371,#16372),
 .UNSPECIFIED.,.F.,.F.,(4,1,4),(13.8761928695312,14.8542941232055,15.7079632679489),
 .UNSPECIFIED.);
#2094=B_SPLINE_CURVE_WITH_KNOTS('',3,(#16378,#16379,#16380,#16381,#16382,
#16383,#16384,#16385,#16386,#16387,#16388,#16389,#16390,#16391,#16392,#16393,
#16394,#16395,#16396,#16397,#16398,#16399),.UNSPECIFIED.,.F.,.F.,(4,3,3,
3,3,3,3,4),(76.708045941327,76.8129957196859,77.8105670926688,78.8081384656518,
79.8057098386347,80.8032812116176,81.8008525846006,82.7984239575835),
 .UNSPECIFIED.);
#2095=B_SPLINE_CURVE_WITH_KNOTS('',3,(#16403,#16404,#16405,#16406,#16407,
#16408,#16409),.UNSPECIFIED.,.F.,.F.,(4,3,4),(-80.783811092309,-79.8057098386347,
-79.2446069498473),.UNSPECIFIED.);
#2096=B_SPLINE_CURVE_WITH_KNOTS('',3,(#16413,#16414,#16415,#16416,#16417,
#16418,#16419,#16420,#16421,#16422,#16423,#16424,#16425,#16426,#16427,#16428,
#16429,#16430,#16431,#16432,#16433,#16434),.UNSPECIFIED.,.F.,.F.,(4,3,3,
3,3,3,3,4),(-79.2446069498473,-78.8081384656518,-77.8105670926688,-76.8129957196859,
-75.815424346703,-74.81785297372,-73.8202816007371,-72.9614216426678),
 .UNSPECIFIED.);
#2097=B_SPLINE_CURVE_WITH_KNOTS('',3,(#16439,#16440,#16441,#16442,#16443,
#16444,#16445,#16446,#16447,#16448,#16449,#16450,#16451,#16452,#16453,#16454,
#16455,#16456,#16457,#16458,#16459,#16460),.UNSPECIFIED.,.F.,.F.,(4,3,3,
3,3,3,3,4),(70.4248606341475,70.8275674817883,71.8251388547712,72.8227102277542,
73.8202816007371,74.81785297372,75.815424346703,76.708045941327),
 .UNSPECIFIED.);
#2098=B_SPLINE_CURVE_WITH_KNOTS('',3,(#16461,#16462,#16463,#16464,#16465,
#16466,#16467,#16468,#16469,#16470,#16471,#16472,#16473,#16474,#16475,#16476,
#16477,#16478,#16479,#16480,#16481,#16482,#16483,#16484,#16485),
 .UNSPECIFIED.,.F.,.F.,(4,3,3,3,3,3,3,3,4),(-72.9614216426678,-72.8227102277542,
-71.8251388547712,-70.8275674817883,-69.8299961088054,-68.8324247358224,
-67.8348533628395,-66.8372819898566,-66.6782363354882),.UNSPECIFIED.);
#2099=B_SPLINE_CURVE_WITH_KNOTS('',3,(#16490,#16491,#16492,#16493,#16494,
#16495,#16496,#16497,#16498,#16499,#16500,#16501,#16502,#16503,#16504,#16505,
#16506,#16507,#16508,#16509,#16510,#16511),.UNSPECIFIED.,.F.,.F.,(4,3,3,
3,3,3,3,4),(64.1416753269678,64.8421392438907,65.8397106168736,66.8372819898565,
67.8348533628395,68.8324247358224,69.8299961088054,70.4248606341475),
 .UNSPECIFIED.);
#2100=B_SPLINE_CURVE_WITH_KNOTS('',3,(#16512,#16513,#16514,#16515,#16516,
#16517,#16518,#16519,#16520,#16521,#16522,#16523,#16524,#16525,#16526,#16527,
#16528,#16529,#16530,#16531,#16532,#16533),.UNSPECIFIED.,.F.,.F.,(4,3,3,
3,3,3,3,4),(-66.6782363354882,-65.8397106168736,-64.8421392438907,-63.8445678709078,
-62.8469964979248,-61.8494251249419,-60.851853751959,-60.3950510283085),
 .UNSPECIFIED.);
#2101=B_SPLINE_CURVE_WITH_KNOTS('',3,(#16538,#16539,#16540,#16541,#16542,
#16543,#16544,#16545,#16546,#16547,#16548,#16549,#16550,#16551,#16552,#16553,
#16554,#16555,#16556,#16557,#16558,#16559),.UNSPECIFIED.,.F.,.F.,(4,3,3,
3,3,3,3,4),(57.8584900197882,58.8567110059931,59.854282378976,60.8518537519589,
61.8494251249419,62.8469964979248,63.8445678709078,64.1416753269678),
 .UNSPECIFIED.);
#2102=B_SPLINE_CURVE_WITH_KNOTS('',3,(#16560,#16561,#16562,#16563,#16564,
#16565,#16566,#16567,#16568,#16569,#16570,#16571,#16572,#16573,#16574,#16575,
#16576,#16577,#16578,#16579,#16580,#16581),.UNSPECIFIED.,.F.,.F.,(4,3,3,
3,3,3,3,4),(-60.3950510283085,-59.854282378976,-58.8567110059931,-57.8591396330102,
-56.8615682600272,-55.8639968870443,-54.8664255140614,-54.1118657211289),
 .UNSPECIFIED.);
#2103=B_SPLINE_CURVE_WITH_KNOTS('',3,(#16586,#16587,#16588,#16589,#16590,
#16591,#16592,#16593,#16594,#16595,#16596,#16597,#16598,#16599,#16600,#16601,
#16602,#16603,#16604,#16605,#16606,#16607),.UNSPECIFIED.,.F.,.F.,(4,3,3,
3,3,3,3,4),(51.5753047126087,51.8737113951126,52.8712827680955,53.8688541410784,
54.8664255140614,55.8639968870443,56.8615682600272,57.8584900197882),
 .UNSPECIFIED.);
#2104=B_SPLINE_CURVE_WITH_KNOTS('',3,(#16608,#16609,#16610,#16611,#16612,
#16613,#16614,#16615,#16616,#16617,#16618,#16619,#16620,#16621,#16622,#16623,
#16624,#16625,#16626,#16627,#16628,#16629,#16630,#16631,#16632),
 .UNSPECIFIED.,.F.,.F.,(4,3,3,3,3,3,3,3,4),(-54.1118657211289,-53.8688541410784,
-52.8712827680955,-51.8737113951126,-50.8761400221296,-49.8785686491467,
-48.8809972761638,-47.8834259031808,-47.8286804139493),.UNSPECIFIED.);
#2105=B_SPLINE_CURVE_WITH_KNOTS('',3,(#16637,#16638,#16639,#16640,#16641,
#16642,#16643,#16644,#16645,#16646,#16647,#16648,#16649,#16650,#16651,#16652,
#16653,#16654,#16655,#16656,#16657,#16658),.UNSPECIFIED.,.F.,.F.,(4,3,3,
3,3,3,3,4),(45.2921194054291,45.888283157215,46.8858545301979,47.8834259031808,
48.8809972761637,49.8785686491467,50.8761400221296,51.5753047126087),
 .UNSPECIFIED.);
#2106=B_SPLINE_CURVE_WITH_KNOTS('',3,(#16659,#16660,#16661,#16662,#16663,
#16664,#16665,#16666,#16667,#16668,#16669,#16670,#16671,#16672,#16673,#16674,
#16675,#16676,#16677,#16678,#16679,#16680),.UNSPECIFIED.,.F.,.F.,(4,3,3,
3,3,3,3,4),(-47.8286804139493,-46.8858545301979,-45.888283157215,-44.890711784232,
-43.8931404112491,-42.8955690382662,-41.8979976652832,-41.5454951067698),
 .UNSPECIFIED.);
#2107=B_SPLINE_CURVE_WITH_KNOTS('',3,(#16685,#16686,#16687,#16688,#16689,
#16690,#16691,#16692,#16693,#16694,#16695,#16696,#16697,#16698,#16699,#16700,
#16701,#16702,#16703,#16704,#16705,#16706),.UNSPECIFIED.,.F.,.F.,(4,3,3,
3,3,3,3,4),(39.0089340982495,39.9028549193174,40.9004262923003,41.8979976652832,
42.8955690382662,43.8931404112491,44.890711784232,45.2921194054291),
 .UNSPECIFIED.);
#2108=B_SPLINE_CURVE_WITH_KNOTS('',3,(#16707,#16708,#16709,#16710,#16711,
#16712,#16713,#16714,#16715,#16716,#16717,#16718,#16719,#16720,#16721,#16722,
#16723,#16724,#16725,#16726,#16727,#16728),.UNSPECIFIED.,.F.,.F.,(4,3,3,
3,3,3,3,4),(-41.5454951067698,-40.9004262923003,-39.9028549193174,-38.9052835463344,
-37.9077121733515,-36.9101408003686,-35.9125694273856,-35.2623097995902),
 .UNSPECIFIED.);
#2109=B_SPLINE_CURVE_WITH_KNOTS('',3,(#16733,#16734,#16735,#16736,#16737,
#16738,#16739,#16740,#16741,#16742,#16743,#16744,#16745,#16746,#16747,#16748,
#16749,#16750,#16751,#16752,#16753,#16754,#16755,#16756,#16757),
 .UNSPECIFIED.,.F.,.F.,(4,3,3,3,3,3,3,3,4),(32.7257487910699,32.9198553084368,
33.9174266814197,34.9149980544027,35.9125694273856,36.9101408003685,37.9077121733515,
38.9052835463344,39.0089340982495),.UNSPECIFIED.);
#2110=B_SPLINE_CURVE_WITH_KNOTS('',3,(#16758,#16759,#16760,#16761,#16762,
#16763,#16764,#16765,#16766,#16767,#16768,#16769,#16770,#16771,#16772,#16773,
#16774,#16775,#16776,#16777,#16778,#16779),.UNSPECIFIED.,.F.,.F.,(4,3,3,
3,3,3,3,4),(-35.2623097995902,-34.9149980544027,-33.9174266814198,-32.9198553084368,
-31.9222839354539,-30.924712562471,-29.927141189488,-28.9791244924106),
 .UNSPECIFIED.);
#2111=B_SPLINE_CURVE_WITH_KNOTS('',3,(#16784,#16785,#16786,#16787,#16788,
#16789,#16790,#16791,#16792,#16793,#16794,#16795,#16796,#16797,#16798,#16799,
#16800,#16801,#16802,#16803,#16804,#16805),.UNSPECIFIED.,.F.,.F.,(4,3,3,
3,3,3,3,4),(26.4425634838903,26.9344270705392,27.9319984435221,28.9295698165051,
29.927141189488,30.9247125624709,31.9222839354539,32.7257487910699),
 .UNSPECIFIED.);
#2112=B_SPLINE_CURVE_WITH_KNOTS('',3,(#16806,#16807,#16808,#16809,#16810,
#16811,#16812,#16813,#16814,#16815,#16816,#16817,#16818,#16819,#16820,#16821,
#16822,#16823,#16824,#16825,#16826,#16827,#16828,#16829,#16830),
 .UNSPECIFIED.,.F.,.F.,(4,3,3,3,3,3,3,3,4),(-28.9791244924106,-28.9295698165051,
-27.9319984435222,-26.9344270705392,-25.9368556975563,-24.9392843245734,
-23.9417129515904,-22.9441415786075,-22.695939185231),.UNSPECIFIED.);
#2113=B_SPLINE_CURVE_WITH_KNOTS('',3,(#16835,#16836,#16837,#16838,#16839,
#16840,#16841,#16842,#16843,#16844,#16845,#16846,#16847,#16848,#16849,#16850,
#16851,#16852,#16853,#16854,#16855,#16856),.UNSPECIFIED.,.F.,.F.,(4,3,3,
3,3,3,3,4),(20.1593781767107,20.9489988326416,21.9465702056245,22.9441415786075,
23.9417129515904,24.9392843245733,25.9368556975563,26.4425634838903),
 .UNSPECIFIED.);
#2114=B_SPLINE_CURVE_WITH_KNOTS('',3,(#16857,#16858,#16859,#16860,#16861,
#16862,#16863,#16864,#16865,#16866,#16867,#16868,#16869,#16870,#16871,#16872,
#16873,#16874,#16875,#16876,#16877,#16878),.UNSPECIFIED.,.F.,.F.,(4,3,3,
3,3,3,3,4),(-22.695939185231,-21.9465702056245,-20.9489988326416,-19.9514274596587,
-18.9538560866757,-17.9562847136928,-16.9587133407099,-16.4127538780514),
 .UNSPECIFIED.);
#2115=B_SPLINE_CURVE_WITH_KNOTS('',3,(#16883,#16884,#16885,#16886,#16887,
#16888,#16889,#16890,#16891,#16892,#16893,#16894,#16895,#16896,#16897,#16898,
#16899,#16900,#16901,#16902,#16903,#16904,#16905,#16906,#16907),
 .UNSPECIFIED.,.F.,.F.,(4,3,3,3,3,3,3,3,4),(13.8761928695311,13.9659992217611,
14.963570594744,15.9611419677269,16.9587133407099,17.9562847136928,18.9538560866757,
19.9514274596587,20.1593781767107),.UNSPECIFIED.);
#2116=B_SPLINE_CURVE_WITH_KNOTS('',3,(#16908,#16909,#16910,#16911,#16912,
#16913,#16914,#16915,#16916,#16917,#16918,#16919,#16920,#16921,#16922,#16923,
#16924,#16925,#16926,#16927,#16928,#16929),.UNSPECIFIED.,.F.,.F.,(4,3,3,
3,3,3,3,4),(-16.4127538780514,-15.9611419677269,-14.963570594744,-13.9659992217611,
-12.9684278487781,-11.9708564757952,-10.9732851028123,-10.1295685708718),
 .UNSPECIFIED.);
#2117=B_SPLINE_CURVE_WITH_KNOTS('',3,(#16935,#16936,#16937,#16938,#16939,
#16940,#16941,#16942,#16943,#16944,#16945,#16946,#16947),.UNSPECIFIED.,
 .F.,.F.,(4,3,3,3,4),(-3.84638326369226,-2.9927141189488,-1.99514274596587,
-0.997571372982934,0.),.UNSPECIFIED.);
#2118=B_SPLINE_CURVE_WITH_KNOTS('',3,(#16950,#16951,#16952,#16953,#16954,
#16955,#16956,#16957,#16958,#16959,#16960,#16961,#16962,#16963,#16964,#16965,
#16966,#16967,#16968),.UNSPECIFIED.,.F.,.F.,(4,3,3,3,3,3,4),(2.01461286527449,
2.9927141189488,3.99028549193174,4.98785686491467,5.9854282378976,6.98299961088054,
7.59300756235157),.UNSPECIFIED.);
#2119=B_SPLINE_CURVE_WITH_KNOTS('',3,(#16974,#16975,#16976,#16977,#16978,
#16979,#16980),.UNSPECIFIED.,.F.,.F.,(4,1,1,1,4),(91.106186954104,91.6672898428914,
92.6648612158743,93.6624325888573,94.6600039618402),.UNSPECIFIED.);
#2120=B_SPLINE_CURVE_WITH_KNOTS('',3,(#16983,#16984,#16985,#16986,#16987,
#16988,#16989,#16990),.UNSPECIFIED.,.F.,.F.,(4,1,1,1,1,4),(91.106186954104,
91.2111367324628,92.2087081054457,93.2062794784287,94.2038508514116,95.1819521050859),
 .UNSPECIFIED.);
#2121=B_SPLINE_CURVE_WITH_KNOTS('',3,(#16995,#16996,#16997,#16998,#16999,
#17000,#17001,#17002,#17003,#17004),.UNSPECIFIED.,.F.,.F.,(4,1,1,1,1,1,
1,4),(84.8230016469245,85.6818616049938,86.6794329779767,87.6770043509596,
88.6745757239426,89.6721470969255,90.6697184699085,91.106186954104),
 .UNSPECIFIED.);
#2122=B_SPLINE_CURVE_WITH_KNOTS('',3,(#17005,#17006,#17007,#17008,#17009,
#17010,#17011,#17012,#17013,#17014),.UNSPECIFIED.,.F.,.F.,(4,1,1,1,1,1,
1,4),(84.8230016469244,85.2257084945652,86.2232798675481,87.2208512405311,
88.218422613514,89.2159939864969,90.2135653594799,91.106186954104),
 .UNSPECIFIED.);
#2123=B_SPLINE_CURVE_WITH_KNOTS('',3,(#17019,#17020,#17021,#17022,#17023,
#17024,#17025,#17026,#17027,#17028,#17029),.UNSPECIFIED.,.F.,.F.,(4,1,1,
1,1,1,1,1,4),(78.5398163397448,78.6988619941132,79.6964333670962,80.6940047400791,
81.6915761130621,82.689147486045,83.6867188590279,84.6842902320109,84.8230016469245),
 .UNSPECIFIED.);
#2124=B_SPLINE_CURVE_WITH_KNOTS('',3,(#17030,#17031,#17032,#17033,#17034,
#17035,#17036,#17037,#17038,#17039),.UNSPECIFIED.,.F.,.F.,(4,1,1,1,1,1,
1,4),(78.5398163397448,79.2402802566676,80.2378516296505,81.2354230026335,
82.2329943756164,83.2305657485993,84.2281371215823,84.8230016469244),
 .UNSPECIFIED.);
#2125=B_SPLINE_CURVE_WITH_KNOTS('',3,(#17044,#17045,#17046,#17047,#17048,
#17049,#17050,#17051,#17052,#17053),.UNSPECIFIED.,.F.,.F.,(4,1,1,1,1,1,
1,4),(72.2566310325652,72.7134337562156,73.7110051291986,74.7085765021815,
75.7061478751644,76.7037192481474,77.7012906211303,78.5398163397448),
 .UNSPECIFIED.);
#2126=B_SPLINE_CURVE_WITH_KNOTS('',3,(#17054,#17055,#17056,#17057,#17058,
#17059,#17060,#17061,#17062,#17063,#17064),.UNSPECIFIED.,.F.,.F.,(4,1,1,
1,1,1,1,1,4),(72.2566310325652,72.2572806457871,73.25485201877,74.2524233917529,
75.2499947647359,76.2475661377188,77.2451375107017,78.2427088836847,78.5398163397448),
 .UNSPECIFIED.);
#2127=B_SPLINE_CURVE_WITH_KNOTS('',3,(#17069,#17070,#17071,#17072,#17073,
#17074,#17075,#17076,#17077,#17078),.UNSPECIFIED.,.F.,.F.,(4,1,1,1,1,1,
1,4),(65.9734457253856,66.728005518318,67.725576891301,68.7231482642839,
69.7207196372669,70.7182910102498,71.7158623832327,72.2566310325652),
 .UNSPECIFIED.);
#2128=B_SPLINE_CURVE_WITH_KNOTS('',3,(#17079,#17080,#17081,#17082,#17083,
#17084,#17085,#17086,#17087,#17088),.UNSPECIFIED.,.F.,.F.,(4,1,1,1,1,1,
1,4),(65.9734457253856,66.2718524078895,67.2694237808724,68.2669951538553,
69.2645665268383,70.2621378998212,71.2597092728041,72.2566310325652),
 .UNSPECIFIED.);
#2129=B_SPLINE_CURVE_WITH_KNOTS('',3,(#17093,#17094,#17095,#17096,#17097,
#17098,#17099,#17100,#17101,#17102,#17103),.UNSPECIFIED.,.F.,.F.,(4,1,1,
1,1,1,1,1,4),(59.690260418206,59.7450059074375,60.7425772804204,61.7401486534034,
62.7377200263863,63.7352913993692,64.7328627723522,65.7304341453351,65.9734457253856),
 .UNSPECIFIED.);
#2130=B_SPLINE_CURVE_WITH_KNOTS('',3,(#17104,#17105,#17106,#17107,#17108,
#17109,#17110,#17111,#17112,#17113),.UNSPECIFIED.,.F.,.F.,(4,1,1,1,1,1,
1,4),(59.690260418206,60.2864241699919,61.2839955429748,62.2815669159577,
63.2791382889407,64.2767096619236,65.2742810349065,65.9734457253856),
 .UNSPECIFIED.);
#2131=B_SPLINE_CURVE_WITH_KNOTS('',3,(#17118,#17119,#17120,#17121,#17122,
#17123,#17124,#17125,#17126,#17127),.UNSPECIFIED.,.F.,.F.,(4,1,1,1,1,1,
1,4),(53.4070751110265,53.7595776695399,54.7571490425228,55.7547204155058,
56.7522917884887,57.7498631614716,58.7474345344546,59.690260418206),
 .UNSPECIFIED.);
#2132=B_SPLINE_CURVE_WITH_KNOTS('',3,(#17128,#17129,#17130,#17131,#17132,
#17133,#17134,#17135,#17136,#17137),.UNSPECIFIED.,.F.,.F.,(4,1,1,1,1,1,
1,4),(53.4070751110264,54.3009959320943,55.2985673050772,56.2961386780601,
57.2937100510431,58.291281424026,59.2888527970089,59.690260418206),
 .UNSPECIFIED.);
#2133=B_SPLINE_CURVE_WITH_KNOTS('',3,(#17142,#17143,#17144,#17145,#17146,
#17147,#17148,#17149,#17150,#17151),.UNSPECIFIED.,.F.,.F.,(4,1,1,1,1,1,
1,4),(47.1238898038469,47.7741494316423,48.7717208046252,49.7692921776082,
50.7668635505911,51.764434923574,52.762006296557,53.4070751110265),
 .UNSPECIFIED.);
#2134=B_SPLINE_CURVE_WITH_KNOTS('',3,(#17152,#17153,#17154,#17155,#17156,
#17157,#17158,#17159,#17160,#17161,#17162),.UNSPECIFIED.,.F.,.F.,(4,1,1,
1,1,1,1,1,4),(47.1238898038469,47.3179963212137,48.3155676941967,49.3131390671796,
50.3107104401625,51.3082818131455,52.3058531861284,53.3034245591113,53.4070751110264),
 .UNSPECIFIED.);
#2135=B_SPLINE_CURVE_WITH_KNOTS('',3,(#17167,#17168,#17169,#17170,#17171,
#17172,#17173,#17174,#17175,#17176),.UNSPECIFIED.,.F.,.F.,(4,1,1,1,1,1,
1,4),(40.8407044966673,41.7887211937447,42.7862925667276,43.7838639397106,
44.7814353126935,45.7790066856764,46.7765780586594,47.1238898038469),
 .UNSPECIFIED.);
#2136=B_SPLINE_CURVE_WITH_KNOTS('',3,(#17177,#17178,#17179,#17180,#17181,
#17182,#17183,#17184,#17185,#17186),.UNSPECIFIED.,.F.,.F.,(4,1,1,1,1,1,
1,4),(40.8407044966673,41.3325680833161,42.3301394562991,43.327710829282,
44.3252822022649,45.3228535752479,46.3204249482308,47.1238898038469),
 .UNSPECIFIED.);
#2137=B_SPLINE_CURVE_WITH_KNOTS('',3,(#17191,#17192,#17193,#17194,#17195,
#17196,#17197,#17198,#17199,#17200,#17201),.UNSPECIFIED.,.F.,.F.,(4,1,1,
1,1,1,1,1,4),(34.5575191894876,34.8057215828642,35.8032929558471,36.80086432883,
37.798435701813,38.7960070747959,39.7935784477788,40.7911498207618,40.8407044966673),
 .UNSPECIFIED.);
#2138=B_SPLINE_CURVE_WITH_KNOTS('',3,(#17202,#17203,#17204,#17205,#17206,
#17207,#17208,#17209,#17210,#17211),.UNSPECIFIED.,.F.,.F.,(4,1,1,1,1,1,
1,4),(34.5575191894876,35.3471398454185,36.3447112184015,37.3422825913844,
38.3398539643673,39.3374253373503,40.3349967103332,40.8407044966673),
 .UNSPECIFIED.);
#2139=B_SPLINE_CURVE_WITH_KNOTS('',3,(#17216,#17217,#17218,#17219,#17220,
#17221,#17222,#17223,#17224,#17225),.UNSPECIFIED.,.F.,.F.,(4,1,1,1,1,1,
1,4),(28.2743338823081,28.8202933449666,29.8178647179495,30.8154360909324,
31.8130074639154,32.8105788368983,33.8081502098812,34.5575191894876),
 .UNSPECIFIED.);
#2140=B_SPLINE_CURVE_WITH_KNOTS('',3,(#17226,#17227,#17228,#17229,#17230,
#17231,#17232,#17233,#17234,#17235,#17236),.UNSPECIFIED.,.F.,.F.,(4,1,1,
1,1,1,1,1,4),(28.2743338823081,28.364140234538,29.3617116075209,30.3592829805039,
31.3568543534868,32.3544257264697,33.3519970994527,34.3495684724356,34.5575191894876),
 .UNSPECIFIED.);
#2141=B_SPLINE_CURVE_WITH_KNOTS('',3,(#17241,#17242,#17243,#17244,#17245,
#17246,#17247,#17248,#17249,#17250),.UNSPECIFIED.,.F.,.F.,(4,1,1,1,1,1,
1,4),(21.9911485751285,22.834865107069,23.8324364800519,24.8300078530348,
25.8275792260178,26.8251505990007,27.8227219719836,28.2743338823081),
 .UNSPECIFIED.);
#2142=B_SPLINE_CURVE_WITH_KNOTS('',3,(#17251,#17252,#17253,#17254,#17255,
#17256,#17257,#17258,#17259,#17260),.UNSPECIFIED.,.F.,.F.,(4,1,1,1,1,1,
1,4),(21.9911485751285,22.3787119966404,23.3762833696233,24.3738547426063,
25.3714261155892,26.3689974885721,27.3665688615551,28.2743338823081),
 .UNSPECIFIED.);
#2143=B_SPLINE_CURVE_WITH_KNOTS('',3,(#17266,#17267,#17268,#17269,#17270),
 .UNSPECIFIED.,.F.,.F.,(4,1,4),(14.3981410127769,15.3957123857599,15.7079632679489),
 .UNSPECIFIED.);
#2144=B_SPLINE_CURVE_WITH_KNOTS('',3,(#17273,#17274,#17275,#17276,#17277),
 .UNSPECIFIED.,.F.,.F.,(4,1,4),(13.8761928695312,14.8542941232055,15.7079632679489),
 .UNSPECIFIED.);
#2145=B_SPLINE_CURVE_WITH_KNOTS('',3,(#17283,#17284,#17285,#17286,#17287,
#17288,#17289,#17290,#17291,#17292,#17293,#17294,#17295,#17296,#17297,#17298,
#17299,#17300,#17301,#17302,#17303,#17304),.UNSPECIFIED.,.F.,.F.,(4,3,3,
3,3,3,3,4),(76.708045941327,76.812995719686,77.8105670926689,78.8081384656519,
79.8057098386348,80.8032812116177,81.8008525846006,82.7984239575836),
 .UNSPECIFIED.);
#2146=B_SPLINE_CURVE_WITH_KNOTS('',3,(#17308,#17309,#17310,#17311,#17312,
#17313,#17314),.UNSPECIFIED.,.F.,.F.,(4,3,4),(-80.7838110923091,-79.8057098386348,
-79.2446069498473),.UNSPECIFIED.);
#2147=B_SPLINE_CURVE_WITH_KNOTS('',3,(#17318,#17319,#17320,#17321,#17322,
#17323,#17324,#17325,#17326,#17327,#17328,#17329,#17330,#17331,#17332,#17333,
#17334,#17335,#17336,#17337,#17338,#17339),.UNSPECIFIED.,.F.,.F.,(4,3,3,
3,3,3,3,4),(-79.2446069498473,-78.8081384656519,-77.8105670926689,-76.812995719686,
-75.815424346703,-74.8178529737201,-73.8202816007372,-72.9614216426678),
 .UNSPECIFIED.);
#2148=B_SPLINE_CURVE_WITH_KNOTS('',3,(#17344,#17345,#17346,#17347,#17348,
#17349,#17350,#17351,#17352,#17353,#17354,#17355,#17356,#17357,#17358,#17359,
#17360,#17361,#17362,#17363,#17364,#17365),.UNSPECIFIED.,.F.,.F.,(4,3,3,
3,3,3,3,4),(70.4248606341475,70.8275674817884,71.8251388547713,72.8227102277542,
73.8202816007372,74.8178529737201,75.815424346703,76.708045941327),
 .UNSPECIFIED.);
#2149=B_SPLINE_CURVE_WITH_KNOTS('',3,(#17366,#17367,#17368,#17369,#17370,
#17371,#17372,#17373,#17374,#17375,#17376,#17377,#17378,#17379,#17380,#17381,
#17382,#17383,#17384,#17385,#17386,#17387,#17388,#17389,#17390),
 .UNSPECIFIED.,.F.,.F.,(4,3,3,3,3,3,3,3,4),(-72.9614216426678,-72.8227102277542,
-71.8251388547713,-70.8275674817884,-69.8299961088054,-68.8324247358225,
-67.8348533628396,-66.8372819898566,-66.6782363354882),.UNSPECIFIED.);
#2150=B_SPLINE_CURVE_WITH_KNOTS('',3,(#17395,#17396,#17397,#17398,#17399,
#17400,#17401,#17402,#17403,#17404,#17405,#17406,#17407,#17408,#17409,#17410,
#17411,#17412,#17413,#17414,#17415,#17416),.UNSPECIFIED.,.F.,.F.,(4,3,3,
3,3,3,3,4),(64.1416753269678,64.8421392438907,65.8397106168737,66.8372819898566,
67.8348533628396,68.8324247358225,69.8299961088054,70.4248606341475),
 .UNSPECIFIED.);
#2151=B_SPLINE_CURVE_WITH_KNOTS('',3,(#17417,#17418,#17419,#17420,#17421,
#17422,#17423,#17424,#17425,#17426,#17427,#17428,#17429,#17430,#17431,#17432,
#17433,#17434,#17435,#17436,#17437,#17438),.UNSPECIFIED.,.F.,.F.,(4,3,3,
3,3,3,3,4),(-66.6782363354882,-65.8397106168737,-64.8421392438908,-63.8445678709078,
-62.8469964979249,-61.849425124942,-60.851853751959,-60.3950510283085),
 .UNSPECIFIED.);
#2152=B_SPLINE_CURVE_WITH_KNOTS('',3,(#17443,#17444,#17445,#17446,#17447,
#17448,#17449,#17450,#17451,#17452,#17453,#17454,#17455,#17456,#17457,#17458,
#17459,#17460,#17461,#17462,#17463,#17464),.UNSPECIFIED.,.F.,.F.,(4,3,3,
3,3,3,3,4),(57.8584900197882,58.8567110059932,59.8542823789761,60.851853751959,
61.849425124942,62.8469964979249,63.8445678709078,64.1416753269678),
 .UNSPECIFIED.);
#2153=B_SPLINE_CURVE_WITH_KNOTS('',3,(#17465,#17466,#17467,#17468,#17469,
#17470,#17471,#17472,#17473,#17474,#17475,#17476,#17477,#17478,#17479,#17480,
#17481,#17482,#17483,#17484,#17485,#17486),.UNSPECIFIED.,.F.,.F.,(4,3,3,
3,3,3,3,4),(-60.3950510283085,-59.8542823789761,-58.8567110059932,-57.8591396330102,
-56.8615682600273,-55.8639968870443,-54.8664255140614,-54.1118657211289),
 .UNSPECIFIED.);
#2154=B_SPLINE_CURVE_WITH_KNOTS('',3,(#17491,#17492,#17493,#17494,#17495,
#17496,#17497,#17498,#17499,#17500,#17501,#17502,#17503,#17504,#17505,#17506,
#17507,#17508,#17509,#17510,#17511,#17512),.UNSPECIFIED.,.F.,.F.,(4,3,3,
3,3,3,3,4),(51.5753047126087,51.8737113951126,52.8712827680955,53.8688541410785,
54.8664255140614,55.8639968870443,56.8615682600273,57.8584900197882),
 .UNSPECIFIED.);
#2155=B_SPLINE_CURVE_WITH_KNOTS('',3,(#17513,#17514,#17515,#17516,#17517,
#17518,#17519,#17520,#17521,#17522,#17523,#17524,#17525,#17526,#17527,#17528,
#17529,#17530,#17531,#17532,#17533,#17534,#17535,#17536,#17537),
 .UNSPECIFIED.,.F.,.F.,(4,3,3,3,3,3,3,3,4),(-54.1118657211289,-53.8688541410785,
-52.8712827680955,-51.8737113951126,-50.8761400221297,-49.8785686491467,
-48.8809972761638,-47.8834259031809,-47.8286804139493),.UNSPECIFIED.);
#2156=B_SPLINE_CURVE_WITH_KNOTS('',3,(#17542,#17543,#17544,#17545,#17546,
#17547,#17548,#17549,#17550,#17551,#17552,#17553,#17554,#17555,#17556,#17557,
#17558,#17559,#17560,#17561,#17562,#17563),.UNSPECIFIED.,.F.,.F.,(4,3,3,
3,3,3,3,4),(45.2921194054291,45.888283157215,46.8858545301979,47.8834259031809,
48.8809972761638,49.8785686491467,50.8761400221297,51.5753047126087),
 .UNSPECIFIED.);
#2157=B_SPLINE_CURVE_WITH_KNOTS('',3,(#17564,#17565,#17566,#17567,#17568,
#17569,#17570,#17571,#17572,#17573,#17574,#17575,#17576,#17577,#17578,#17579,
#17580,#17581,#17582,#17583,#17584,#17585),.UNSPECIFIED.,.F.,.F.,(4,3,3,
3,3,3,3,4),(-47.8286804139493,-46.8858545301979,-45.888283157215,-44.8907117842321,
-43.8931404112491,-42.8955690382662,-41.8979976652833,-41.5454951067698),
 .UNSPECIFIED.);
#2158=B_SPLINE_CURVE_WITH_KNOTS('',3,(#17590,#17591,#17592,#17593,#17594,
#17595,#17596,#17597,#17598,#17599,#17600,#17601,#17602,#17603,#17604,#17605,
#17606,#17607,#17608,#17609,#17610,#17611),.UNSPECIFIED.,.F.,.F.,(4,3,3,
3,3,3,3,4),(39.0089340982495,39.9028549193174,40.9004262923003,41.8979976652833,
42.8955690382662,43.8931404112491,44.8907117842321,45.2921194054291),
 .UNSPECIFIED.);
#2159=B_SPLINE_CURVE_WITH_KNOTS('',3,(#17612,#17613,#17614,#17615,#17616,
#17617,#17618,#17619,#17620,#17621,#17622,#17623,#17624,#17625,#17626,#17627,
#17628,#17629,#17630,#17631,#17632,#17633),.UNSPECIFIED.,.F.,.F.,(4,3,3,
3,3,3,3,4),(-41.5454951067698,-40.9004262923003,-39.9028549193174,-38.9052835463345,
-37.9077121733515,-36.9101408003686,-35.9125694273856,-35.2623097995902),
 .UNSPECIFIED.);
#2160=B_SPLINE_CURVE_WITH_KNOTS('',3,(#17638,#17639,#17640,#17641,#17642,
#17643,#17644,#17645,#17646,#17647,#17648,#17649,#17650,#17651,#17652,#17653,
#17654,#17655,#17656,#17657,#17658,#17659,#17660,#17661,#17662),
 .UNSPECIFIED.,.F.,.F.,(4,3,3,3,3,3,3,3,4),(32.7257487910699,32.9198553084369,
33.9174266814198,34.9149980544027,35.9125694273857,36.9101408003686,37.9077121733515,
38.9052835463345,39.0089340982495),.UNSPECIFIED.);
#2161=B_SPLINE_CURVE_WITH_KNOTS('',3,(#17663,#17664,#17665,#17666,#17667,
#17668,#17669,#17670,#17671,#17672,#17673,#17674,#17675,#17676,#17677,#17678,
#17679,#17680,#17681,#17682,#17683,#17684),.UNSPECIFIED.,.F.,.F.,(4,3,3,
3,3,3,3,4),(-35.2623097995902,-34.9149980544027,-33.9174266814198,-32.9198553084368,
-31.9222839354539,-30.924712562471,-29.927141189488,-28.9791244924106),
 .UNSPECIFIED.);
#2162=B_SPLINE_CURVE_WITH_KNOTS('',3,(#17689,#17690,#17691,#17692,#17693,
#17694,#17695,#17696,#17697,#17698,#17699,#17700,#17701,#17702,#17703,#17704,
#17705,#17706,#17707,#17708,#17709,#17710),.UNSPECIFIED.,.F.,.F.,(4,3,3,
3,3,3,3,4),(26.4425634838903,26.9344270705392,27.9319984435222,28.9295698165051,
29.927141189488,30.924712562471,31.9222839354539,32.7257487910699),
 .UNSPECIFIED.);
#2163=B_SPLINE_CURVE_WITH_KNOTS('',3,(#17711,#17712,#17713,#17714,#17715,
#17716,#17717,#17718,#17719,#17720,#17721,#17722,#17723,#17724,#17725,#17726,
#17727,#17728,#17729,#17730,#17731,#17732,#17733,#17734,#17735),
 .UNSPECIFIED.,.F.,.F.,(4,3,3,3,3,3,3,3,4),(-28.9791244924106,-28.9295698165051,
-27.9319984435222,-26.9344270705392,-25.9368556975563,-24.9392843245734,
-23.9417129515904,-22.9441415786075,-22.695939185231),.UNSPECIFIED.);
#2164=B_SPLINE_CURVE_WITH_KNOTS('',3,(#17740,#17741,#17742,#17743,#17744,
#17745,#17746,#17747,#17748,#17749,#17750,#17751,#17752,#17753,#17754,#17755,
#17756,#17757,#17758,#17759,#17760,#17761),.UNSPECIFIED.,.F.,.F.,(4,3,3,
3,3,3,3,4),(20.1593781767107,20.9489988326416,21.9465702056246,22.9441415786075,
23.9417129515904,24.9392843245734,25.9368556975563,26.4425634838903),
 .UNSPECIFIED.);
#2165=B_SPLINE_CURVE_WITH_KNOTS('',3,(#17762,#17763,#17764,#17765,#17766,
#17767,#17768,#17769,#17770,#17771,#17772,#17773,#17774,#17775,#17776,#17777,
#17778,#17779,#17780,#17781,#17782,#17783),.UNSPECIFIED.,.F.,.F.,(4,3,3,
3,3,3,3,4),(-22.695939185231,-21.9465702056246,-20.9489988326416,-19.9514274596587,
-18.9538560866758,-17.9562847136928,-16.9587133407099,-16.4127538780514),
 .UNSPECIFIED.);
#2166=B_SPLINE_CURVE_WITH_KNOTS('',3,(#17788,#17789,#17790,#17791,#17792,
#17793,#17794,#17795,#17796,#17797,#17798,#17799,#17800,#17801,#17802,#17803,
#17804,#17805,#17806,#17807,#17808,#17809,#17810,#17811,#17812),
 .UNSPECIFIED.,.F.,.F.,(4,3,3,3,3,3,3,3,4),(13.8761928695311,13.9659992217611,
14.963570594744,15.961141967727,16.9587133407099,17.9562847136928,18.9538560866758,
19.9514274596587,20.1593781767107),.UNSPECIFIED.);
#2167=B_SPLINE_CURVE_WITH_KNOTS('',3,(#17813,#17814,#17815,#17816,#17817,
#17818,#17819,#17820,#17821,#17822,#17823,#17824,#17825,#17826,#17827,#17828,
#17829,#17830,#17831,#17832,#17833,#17834),.UNSPECIFIED.,.F.,.F.,(4,3,3,
3,3,3,3,4),(-16.4127538780514,-15.961141967727,-14.963570594744,-13.9659992217611,
-12.9684278487782,-11.9708564757952,-10.9732851028123,-10.1295685708718),
 .UNSPECIFIED.);
#2168=B_SPLINE_CURVE_WITH_KNOTS('',3,(#17840,#17841,#17842,#17843,#17844,
#17845,#17846,#17847,#17848,#17849,#17850,#17851,#17852),.UNSPECIFIED.,
 .F.,.F.,(4,3,3,3,4),(-3.84638326369226,-2.9927141189488,-1.99514274596587,
-0.997571372982934,0.),.UNSPECIFIED.);
#2169=B_SPLINE_CURVE_WITH_KNOTS('',3,(#17855,#17856,#17857,#17858,#17859,
#17860,#17861,#17862,#17863,#17864,#17865,#17866,#17867,#17868,#17869,#17870,
#17871,#17872,#17873),.UNSPECIFIED.,.F.,.F.,(4,3,3,3,3,3,4),(2.01461286527449,
2.99271411894881,3.99028549193174,4.98785686491468,5.98542823789761,6.98299961088054,
7.59300756235157),.UNSPECIFIED.);
#2170=B_SPLINE_CURVE_WITH_KNOTS('',3,(#17879,#17880,#17881,#17882,#17883,
#17884,#17885),.UNSPECIFIED.,.F.,.F.,(4,1,1,1,4),(91.106186954104,91.6672898428915,
92.6648612158744,93.6624325888573,94.6600039618403),.UNSPECIFIED.);
#2171=B_SPLINE_CURVE_WITH_KNOTS('',3,(#17888,#17889,#17890,#17891,#17892,
#17893,#17894,#17895),.UNSPECIFIED.,.F.,.F.,(4,1,1,1,1,4),(91.106186954104,
91.2111367324629,92.2087081054458,93.2062794784288,94.2038508514117,95.181952105086),
 .UNSPECIFIED.);
#2172=B_SPLINE_CURVE_WITH_KNOTS('',3,(#17900,#17901,#17902,#17903,#17904,
#17905,#17906,#17907,#17908,#17909),.UNSPECIFIED.,.F.,.F.,(4,1,1,1,1,1,
1,4),(84.8230016469245,85.6818616049939,86.6794329779768,87.6770043509597,
88.6745757239427,89.6721470969256,90.6697184699085,91.106186954104),
 .UNSPECIFIED.);
#2173=B_SPLINE_CURVE_WITH_KNOTS('',3,(#17910,#17911,#17912,#17913,#17914,
#17915,#17916,#17917,#17918,#17919),.UNSPECIFIED.,.F.,.F.,(4,1,1,1,1,1,
1,4),(84.8230016469244,85.2257084945653,86.2232798675482,87.2208512405312,
88.2184226135141,89.215993986497,90.21356535948,91.106186954104),
 .UNSPECIFIED.);
#2174=B_SPLINE_CURVE_WITH_KNOTS('',3,(#17924,#17925,#17926,#17927,#17928,
#17929,#17930,#17931,#17932,#17933,#17934),.UNSPECIFIED.,.F.,.F.,(4,1,1,
1,1,1,1,1,4),(78.5398163397448,78.6988619941133,79.6964333670962,80.6940047400792,
81.6915761130621,82.689147486045,83.686718859028,84.6842902320109,84.8230016469245),
 .UNSPECIFIED.);
#2175=B_SPLINE_CURVE_WITH_KNOTS('',3,(#17935,#17936,#17937,#17938,#17939,
#17940,#17941,#17942,#17943,#17944),.UNSPECIFIED.,.F.,.F.,(4,1,1,1,1,1,
1,4),(78.5398163397448,79.2402802566677,80.2378516296506,81.2354230026336,
82.2329943756165,83.2305657485994,84.2281371215823,84.8230016469244),
 .UNSPECIFIED.);
#2176=B_SPLINE_CURVE_WITH_KNOTS('',3,(#17949,#17950,#17951,#17952,#17953,
#17954,#17955,#17956,#17957,#17958),.UNSPECIFIED.,.F.,.F.,(4,1,1,1,1,1,
1,4),(72.2566310325652,72.7134337562157,73.7110051291986,74.7085765021816,
75.7061478751645,76.7037192481474,77.7012906211304,78.5398163397448),
 .UNSPECIFIED.);
#2177=B_SPLINE_CURVE_WITH_KNOTS('',3,(#17959,#17960,#17961,#17962,#17963,
#17964,#17965,#17966,#17967,#17968,#17969),.UNSPECIFIED.,.F.,.F.,(4,1,1,
1,1,1,1,1,4),(72.2566310325652,72.2572806457871,73.2548520187701,74.252423391753,
75.2499947647359,76.2475661377189,77.2451375107018,78.2427088836847,78.5398163397448),
 .UNSPECIFIED.);
#2178=B_SPLINE_CURVE_WITH_KNOTS('',3,(#17974,#17975,#17976,#17977,#17978,
#17979,#17980,#17981,#17982,#17983),.UNSPECIFIED.,.F.,.F.,(4,1,1,1,1,1,
1,4),(65.9734457253856,66.7280055183181,67.725576891301,68.723148264284,
69.7207196372669,70.7182910102498,71.7158623832328,72.2566310325652),
 .UNSPECIFIED.);
#2179=B_SPLINE_CURVE_WITH_KNOTS('',3,(#17984,#17985,#17986,#17987,#17988,
#17989,#17990,#17991,#17992,#17993),.UNSPECIFIED.,.F.,.F.,(4,1,1,1,1,1,
1,4),(65.9734457253856,66.2718524078895,67.2694237808725,68.2669951538554,
69.2645665268383,70.2621378998213,71.2597092728042,72.2566310325652),
 .UNSPECIFIED.);
#2180=B_SPLINE_CURVE_WITH_KNOTS('',3,(#17998,#17999,#18000,#18001,#18002,
#18003,#18004,#18005,#18006,#18007,#18008),.UNSPECIFIED.,.F.,.F.,(4,1,1,
1,1,1,1,1,4),(59.690260418206,59.7450059074375,60.7425772804205,61.7401486534034,
62.7377200263864,63.7352913993693,64.7328627723522,65.7304341453352,65.9734457253856),
 .UNSPECIFIED.);
#2181=B_SPLINE_CURVE_WITH_KNOTS('',3,(#18009,#18010,#18011,#18012,#18013,
#18014,#18015,#18016,#18017,#18018),.UNSPECIFIED.,.F.,.F.,(4,1,1,1,1,1,
1,4),(59.690260418206,60.2864241699919,61.2839955429748,62.2815669159578,
63.2791382889407,64.2767096619236,65.2742810349066,65.9734457253856),
 .UNSPECIFIED.);
#2182=B_SPLINE_CURVE_WITH_KNOTS('',3,(#18023,#18024,#18025,#18026,#18027,
#18028,#18029,#18030,#18031,#18032),.UNSPECIFIED.,.F.,.F.,(4,1,1,1,1,1,
1,4),(53.4070751110265,53.7595776695399,54.7571490425229,55.7547204155058,
56.7522917884887,57.7498631614717,58.7474345344546,59.690260418206),
 .UNSPECIFIED.);
#2183=B_SPLINE_CURVE_WITH_KNOTS('',3,(#18033,#18034,#18035,#18036,#18037,
#18038,#18039,#18040,#18041,#18042),.UNSPECIFIED.,.F.,.F.,(4,1,1,1,1,1,
1,4),(53.4070751110264,54.3009959320943,55.2985673050772,56.2961386780602,
57.2937100510431,58.291281424026,59.288852797009,59.690260418206),
 .UNSPECIFIED.);
#2184=B_SPLINE_CURVE_WITH_KNOTS('',3,(#18047,#18048,#18049,#18050,#18051,
#18052,#18053,#18054,#18055,#18056),.UNSPECIFIED.,.F.,.F.,(4,1,1,1,1,1,
1,4),(47.1238898038469,47.7741494316423,48.7717208046253,49.7692921776082,
50.7668635505911,51.7644349235741,52.762006296557,53.4070751110265),
 .UNSPECIFIED.);
#2185=B_SPLINE_CURVE_WITH_KNOTS('',3,(#18057,#18058,#18059,#18060,#18061,
#18062,#18063,#18064,#18065,#18066,#18067),.UNSPECIFIED.,.F.,.F.,(4,1,1,
1,1,1,1,1,4),(47.1238898038469,47.3179963212138,48.3155676941967,49.3131390671796,
50.3107104401626,51.3082818131455,52.3058531861284,53.3034245591114,53.4070751110264),
 .UNSPECIFIED.);
#2186=B_SPLINE_CURVE_WITH_KNOTS('',3,(#18072,#18073,#18074,#18075,#18076,
#18077,#18078,#18079,#18080,#18081),.UNSPECIFIED.,.F.,.F.,(4,1,1,1,1,1,
1,4),(40.8407044966673,41.7887211937447,42.7862925667277,43.7838639397106,
44.7814353126935,45.7790066856765,46.7765780586594,47.1238898038469),
 .UNSPECIFIED.);
#2187=B_SPLINE_CURVE_WITH_KNOTS('',3,(#18082,#18083,#18084,#18085,#18086,
#18087,#18088,#18089,#18090,#18091),.UNSPECIFIED.,.F.,.F.,(4,1,1,1,1,1,
1,4),(40.8407044966673,41.3325680833162,42.3301394562991,43.327710829282,
44.325282202265,45.3228535752479,46.3204249482308,47.1238898038469),
 .UNSPECIFIED.);
#2188=B_SPLINE_CURVE_WITH_KNOTS('',3,(#18096,#18097,#18098,#18099,#18100,
#18101,#18102,#18103,#18104,#18105,#18106),.UNSPECIFIED.,.F.,.F.,(4,1,1,
1,1,1,1,1,4),(34.5575191894876,34.8057215828642,35.8032929558471,36.80086432883,
37.798435701813,38.7960070747959,39.7935784477789,40.7911498207618,40.8407044966673),
 .UNSPECIFIED.);
#2189=B_SPLINE_CURVE_WITH_KNOTS('',3,(#18107,#18108,#18109,#18110,#18111,
#18112,#18113,#18114,#18115,#18116),.UNSPECIFIED.,.F.,.F.,(4,1,1,1,1,1,
1,4),(34.5575191894876,35.3471398454185,36.3447112184015,37.3422825913844,
38.3398539643674,39.3374253373503,40.3349967103332,40.8407044966673),
 .UNSPECIFIED.);
#2190=B_SPLINE_CURVE_WITH_KNOTS('',3,(#18121,#18122,#18123,#18124,#18125,
#18126,#18127,#18128,#18129,#18130),.UNSPECIFIED.,.F.,.F.,(4,1,1,1,1,1,
1,4),(28.2743338823081,28.8202933449666,29.8178647179495,30.8154360909324,
31.8130074639154,32.8105788368983,33.8081502098812,34.5575191894876),
 .UNSPECIFIED.);
#2191=B_SPLINE_CURVE_WITH_KNOTS('',3,(#18131,#18132,#18133,#18134,#18135,
#18136,#18137,#18138,#18139,#18140,#18141),.UNSPECIFIED.,.F.,.F.,(4,1,1,
1,1,1,1,1,4),(28.2743338823081,28.364140234538,29.3617116075209,30.3592829805039,
31.3568543534868,32.3544257264697,33.3519970994527,34.3495684724356,34.5575191894876),
 .UNSPECIFIED.);
#2192=B_SPLINE_CURVE_WITH_KNOTS('',3,(#18146,#18147,#18148,#18149,#18150,
#18151,#18152,#18153,#18154,#18155),.UNSPECIFIED.,.F.,.F.,(4,1,1,1,1,1,
1,4),(21.9911485751285,22.834865107069,23.8324364800519,24.8300078530348,
25.8275792260178,26.8251505990007,27.8227219719836,28.2743338823081),
 .UNSPECIFIED.);
#2193=B_SPLINE_CURVE_WITH_KNOTS('',3,(#18156,#18157,#18158,#18159,#18160,
#18161,#18162,#18163,#18164,#18165),.UNSPECIFIED.,.F.,.F.,(4,1,1,1,1,1,
1,4),(21.9911485751285,22.3787119966404,23.3762833696233,24.3738547426063,
25.3714261155892,26.3689974885721,27.3665688615551,28.2743338823081),
 .UNSPECIFIED.);
#2194=B_SPLINE_CURVE_WITH_KNOTS('',3,(#18171,#18172,#18173,#18174,#18175),
 .UNSPECIFIED.,.F.,.F.,(4,1,4),(14.3981410127769,15.3957123857599,15.7079632679489),
 .UNSPECIFIED.);
#2195=B_SPLINE_CURVE_WITH_KNOTS('',3,(#18178,#18179,#18180,#18181,#18182),
 .UNSPECIFIED.,.F.,.F.,(4,1,4),(13.8761928695312,14.8542941232055,15.7079632679489),
 .UNSPECIFIED.);
#2196=B_SPLINE_CURVE_WITH_KNOTS('',3,(#18216,#18217,#18218,#18219,#18220,
#18221,#18222,#18223,#18224,#18225,#18226,#18227,#18228,#18229,#18230,#18231,
#18232,#18233,#18234,#18235,#18236,#18237,#18238,#18239,#18240,#18241,#18242,
#18243,#18244,#18245,#18246,#18247,#18248,#18249,#18250,#18251,#18252,#18253,
#18254,#18255,#18256,#18257,#18258,#18259,#18260,#18261,#18262,#18263,#18264,
#18265,#18266,#18267,#18268,#18269,#18270),.UNSPECIFIED.,.F.,.F.,(4,3,3,
3,3,3,3,3,3,3,3,3,3,3,3,3,3,3,4),(-0.378621596831442,-0.353562246097462,
-0.339726792951542,-0.324795397581524,-0.299967980662127,-0.289118724731059,
-0.252370044287308,-0.234474300298533,-0.219335629396853,-0.200829495678085,
-0.174827324623006,-0.15584693665932,-0.144923737522316,-0.109696956092963,
-0.0896699638623999,-0.0773387259299598,-0.0372142298588392,-0.00401661180490446,
0.),.UNSPECIFIED.);
#2197=B_SPLINE_CURVE_WITH_KNOTS('',3,(#18271,#18272,#18273,#18274,#18275,
#18276,#18277,#18278,#18279,#18280,#18281,#18282,#18283,#18284,#18285,#18286,
#18287,#18288,#18289,#18290,#18291,#18292,#18293,#18294,#18295,#18296,#18297,
#18298,#18299,#18300,#18301,#18302,#18303,#18304,#18305,#18306,#18307,#18308,
#18309,#18310,#18311,#18312,#18313,#18314,#18315,#18316,#18317,#18318,#18319,
#18320,#18321,#18322,#18323,#18324,#18325),.UNSPECIFIED.,.F.,.F.,(4,3,3,
3,3,3,3,3,3,3,3,3,3,3,3,3,3,3,4),(-0.376940817211619,-0.351602437043448,
-0.332519408379845,-0.318228058131088,-0.288333449384516,-0.272718117105765,
-0.234505377427356,-0.216962131374135,-0.205493408420767,-0.180854828870943,
-0.153734180151122,-0.136643041471865,-0.126205700111191,-0.0954718773410078,
-0.0666269097764766,-0.0558557551097461,-0.0219614248579871,-0.00327040903045905,
0.),.UNSPECIFIED.);
#2198=B_SPLINE_CURVE_WITH_KNOTS('',3,(#18327,#18328,#18329,#18330,#18331,
#18332,#18333,#18334,#18335,#18336,#18337),.UNSPECIFIED.,.F.,.F.,(4,1,1,
1,1,1,1,1,4),(15.7079632679489,15.8518654961884,16.8494368691714,17.8470082421543,
18.8445796151372,19.8421509881202,20.8397223611031,21.837293734086,21.9911485751285),
 .UNSPECIFIED.);
#2199=B_SPLINE_CURVE_WITH_KNOTS('',3,(#18338,#18339,#18340,#18341,#18342,
#18343,#18344,#18345,#18346,#18347),.UNSPECIFIED.,.F.,.F.,(4,1,1,1,1,1,
1,4),(15.7079632679489,16.3932837587428,17.3908551317257,18.3884265047087,
19.3859978776916,20.3835692506745,21.3811406236575,21.9911485751285),
 .UNSPECIFIED.);
#2200=B_SPLINE_CURVE_WITH_KNOTS('',3,(#18692,#18693,#18694,#18695,#18696,
#18697,#18698,#18699,#18700,#18701,#18702,#18703,#18704,#18705,#18706,#18707,
#18708,#18709,#18710,#18711,#18712,#18713,#18714,#18715,#18716,#18717,#18718,
#18719,#18720,#18721,#18722,#18723,#18724,#18725,#18726,#18727,#18728,#18729,
#18730,#18731,#18732,#18733,#18734,#18735,#18736,#18737,#18738,#18739,#18740,
#18741,#18742,#18743),.UNSPECIFIED.,.F.,.F.,(4,3,3,3,3,3,3,3,3,3,3,3,3,
3,3,3,3,4),(0.,0.0336910847235707,0.0587346654534766,0.0734852364994148,
0.109792238871862,0.132864830837164,0.143632030356024,0.17720525627004,
0.195911997060402,0.20761397219,0.244895171883038,0.269599304636634,0.282507756557061,
0.310158174405463,0.327757797512771,0.342580165552076,0.372940760482292,
0.376940817211643),.UNSPECIFIED.);
#2201=B_SPLINE_CURVE_WITH_KNOTS('',3,(#18744,#18745,#18746,#18747,#18748,
#18749,#18750,#18751,#18752,#18753,#18754,#18755,#18756,#18757,#18758,#18759,
#18760,#18761,#18762,#18763,#18764,#18765,#18766,#18767,#18768),
 .UNSPECIFIED.,.F.,.F.,(4,3,3,3,3,3,3,3,4),(-10.1295685708718,-9.97571372982935,
-8.97814235684642,-7.98057098386348,-6.98299961088054,-5.98542823789761,
-4.98785686491468,-3.99028549193174,-3.84638326369226),.UNSPECIFIED.);
#2202=B_SPLINE_CURVE_WITH_KNOTS('',3,(#19113,#19114,#19115,#19116,#19117,
#19118,#19119,#19120,#19121,#19122,#19123,#19124,#19125,#19126,#19127,#19128,
#19129,#19130,#19131,#19132,#19133,#19134),.UNSPECIFIED.,.F.,.F.,(4,3,3,
3,3,3,3,4),(7.59300756235157,7.98057098386348,8.97814235684642,9.97571372982935,
10.9732851028123,11.9708564757952,12.9684278487781,13.8761928695311),
 .UNSPECIFIED.);
#2203=B_SPLINE_CURVE_WITH_KNOTS('',3,(#19135,#19136,#19137,#19138,#19139,
#19140,#19141,#19142,#19143,#19144,#19145,#19146,#19147,#19148,#19149,#19150,
#19151,#19152,#19153,#19154,#19155,#19156,#19157,#19158,#19159,#19160,#19161,
#19162,#19163,#19164,#19165,#19166,#19167,#19168,#19169,#19170,#19171,#19172,
#19173,#19174,#19175,#19176,#19177,#19178,#19179,#19180,#19181,#19182,#19183,
#19184,#19185,#19186),.UNSPECIFIED.,.F.,.F.,(4,3,3,3,3,3,3,3,3,3,3,3,3,
3,3,3,3,4),(0.,0.039679134584082,0.0597937574063347,0.077198275206118,0.0898304469160062,
0.128492621633409,0.153526594220962,0.165101500237275,0.197163594226419,
0.224452129979101,0.234160526966568,0.26945519714964,0.287578609071477,
0.305421511169844,0.333081607138838,0.347224899232131,0.375339207698859,
0.378621596831424),.UNSPECIFIED.);
#2204=B_SPLINE_CURVE_WITH_KNOTS('',3,(#19189,#19190,#19191,#19192,#19193,
#19194,#19195,#19196,#19197,#19198,#19199,#19200,#19201,#19202,#19203,#19204,
#19205,#19206,#19207,#19208,#19209,#19210,#19211,#19212,#19213,#19214,#19215,
#19216,#19217,#19218,#19219,#19220,#19221,#19222,#19223,#19224,#19225,#19226,
#19227,#19228,#19229,#19230,#19231,#19232,#19233,#19234,#19235,#19236,#19237,
#19238,#19239,#19240,#19241,#19242,#19243),.UNSPECIFIED.,.F.,.F.,(4,3,3,
3,3,3,3,3,3,3,3,3,3,3,3,3,3,3,4),(-0.378621596831421,-0.35356224610225,
-0.339726792605717,-0.324795397019123,-0.299967964935665,-0.289118709747788,
-0.252370025571504,-0.234474277842488,-0.219335629751949,-0.200829495678081,
-0.174827335946658,-0.155846980593001,-0.144923798098897,-0.109697001525397,
-0.0896700514919927,-0.0773387576028108,-0.0372142610763827,-0.00401661180489582,
0.),.UNSPECIFIED.);
#2205=B_SPLINE_CURVE_WITH_KNOTS('',3,(#19244,#19245,#19246,#19247,#19248,
#19249,#19250,#19251,#19252,#19253,#19254,#19255,#19256,#19257,#19258,#19259,
#19260,#19261,#19262,#19263,#19264,#19265,#19266,#19267,#19268,#19269,#19270,
#19271,#19272,#19273,#19274,#19275,#19276,#19277,#19278,#19279,#19280,#19281,
#19282,#19283,#19284,#19285,#19286,#19287,#19288,#19289,#19290,#19291,#19292,
#19293,#19294,#19295,#19296,#19297,#19298),.UNSPECIFIED.,.F.,.F.,(4,3,3,
3,3,3,3,3,3,3,3,3,3,3,3,3,3,3,4),(-0.376940817211658,-0.35160243790482,
-0.332519425088979,-0.318228074800829,-0.288333550643748,-0.272718146690274,
-0.234505396639293,-0.21696217861614,-0.205493442096022,-0.18085482887096,
-0.153734148588707,-0.136642726461199,-0.12620501784944,-0.095471365644694,
-0.0666260826793201,-0.0558555936353674,-0.021961250336811,-0.00327040903045685,
0.),.UNSPECIFIED.);
#2206=B_SPLINE_CURVE_WITH_KNOTS('',3,(#19300,#19301,#19302,#19303,#19304,
#19305,#19306,#19307,#19308,#19309,#19310),.UNSPECIFIED.,.F.,.F.,(4,1,1,
1,1,1,1,1,4),(15.7079632679489,15.8518654961884,16.8494368691713,17.8470082421543,
18.8445796151372,19.8421509881202,20.8397223611031,21.837293734086,21.9911485751285),
 .UNSPECIFIED.);
#2207=B_SPLINE_CURVE_WITH_KNOTS('',3,(#19311,#19312,#19313,#19314,#19315,
#19316,#19317,#19318,#19319,#19320),.UNSPECIFIED.,.F.,.F.,(4,1,1,1,1,1,
1,4),(15.7079632679489,16.3932837587428,17.3908551317257,18.3884265047087,
19.3859978776916,20.3835692506745,21.3811406236575,21.9911485751285),
 .UNSPECIFIED.);
#2208=B_SPLINE_CURVE_WITH_KNOTS('',3,(#19665,#19666,#19667,#19668,#19669,
#19670,#19671,#19672,#19673,#19674,#19675,#19676,#19677,#19678,#19679,#19680,
#19681,#19682,#19683,#19684,#19685,#19686,#19687,#19688,#19689,#19690,#19691,
#19692,#19693,#19694,#19695,#19696,#19697,#19698,#19699,#19700,#19701,#19702,
#19703,#19704,#19705,#19706,#19707,#19708,#19709,#19710,#19711,#19712,#19713,
#19714,#19715,#19716),.UNSPECIFIED.,.F.,.F.,(4,3,3,3,3,3,3,3,3,3,3,3,3,
3,3,3,3,4),(0.,0.0336910497355155,0.058734651365868,0.0734852344555961,
0.109792226014928,0.132864806965475,0.143631988775342,0.17720525627004,
0.1959120018626,0.20761397470913,0.244895197064516,0.269599368515367,0.282507810536056,
0.310158254371969,0.327758642889101,0.342580296989548,0.372940760482291,
0.376940817211643),.UNSPECIFIED.);
#2209=B_SPLINE_CURVE_WITH_KNOTS('',3,(#19717,#19718,#19719,#19720,#19721,
#19722,#19723,#19724,#19725,#19726,#19727,#19728,#19729,#19730,#19731,#19732,
#19733,#19734,#19735,#19736,#19737,#19738,#19739,#19740,#19741),
 .UNSPECIFIED.,.F.,.F.,(4,3,3,3,3,3,3,3,4),(-10.1295685708718,-9.97571372982934,
-8.97814235684641,-7.98057098386347,-6.98299961088054,-5.9854282378976,
-4.98785686491467,-3.99028549193173,-3.84638326369226),.UNSPECIFIED.);
#2210=B_SPLINE_CURVE_WITH_KNOTS('',3,(#20086,#20087,#20088,#20089,#20090,
#20091,#20092,#20093,#20094,#20095,#20096,#20097,#20098,#20099,#20100,#20101,
#20102,#20103,#20104,#20105,#20106,#20107),.UNSPECIFIED.,.F.,.F.,(4,3,3,
3,3,3,3,4),(7.59300756235157,7.98057098386347,8.9781423568464,9.97571372982934,
10.9732851028123,11.9708564757952,12.9684278487781,13.8761928695311),
 .UNSPECIFIED.);
#2211=B_SPLINE_CURVE_WITH_KNOTS('',3,(#20108,#20109,#20110,#20111,#20112,
#20113,#20114,#20115,#20116,#20117,#20118,#20119,#20120,#20121,#20122,#20123,
#20124,#20125,#20126,#20127,#20128,#20129,#20130,#20131,#20132,#20133,#20134,
#20135,#20136,#20137,#20138,#20139,#20140,#20141,#20142,#20143,#20144,#20145,
#20146,#20147,#20148,#20149,#20150,#20151,#20152,#20153,#20154,#20155,#20156,
#20157,#20158,#20159),.UNSPECIFIED.,.F.,.F.,(4,3,3,3,3,3,3,3,3,3,3,3,3,
3,3,3,3,4),(0.,0.0396791423592224,0.0597938176449427,0.0771989368507012,
0.0898305980572942,0.128492765250004,0.153526730198623,0.165101530608957,
0.197163594226419,0.224452126331546,0.234160522045081,0.269455193458526,
0.287578665402526,0.305421500398064,0.333081575029239,0.347224893982947,
0.375339207698863,0.378621596831429),.UNSPECIFIED.);
#2212=B_SPLINE_CURVE_WITH_KNOTS('',3,(#20162,#20163,#20164,#20165,#20166,
#20167,#20168,#20169,#20170,#20171,#20172,#20173,#20174,#20175,#20176,#20177,
#20178,#20179,#20180,#20181,#20182,#20183,#20184,#20185,#20186,#20187,#20188,
#20189,#20190,#20191,#20192,#20193,#20194,#20195,#20196,#20197,#20198,#20199,
#20200,#20201,#20202,#20203,#20204,#20205,#20206,#20207,#20208,#20209,#20210,
#20211,#20212,#20213,#20214,#20215,#20216),.UNSPECIFIED.,.F.,.F.,(4,3,3,
3,3,3,3,3,3,3,3,3,3,3,3,3,3,3,4),(-0.378621596831421,-0.353562246109156,
-0.3397267922352,-0.324795396410533,-0.299967947923947,-0.289118693566506,
-0.252370005353849,-0.234474253593686,-0.219335630122499,-0.200829495678059,
-0.174827348196324,-0.155847028127452,-0.144923863657138,-0.109697050694078,
-0.089670146324546,-0.0773387918294275,-0.0372142948109077,-0.00401661180489871,
0.),.UNSPECIFIED.);
#2213=B_SPLINE_CURVE_WITH_KNOTS('',3,(#20217,#20218,#20219,#20220,#20221,
#20222,#20223,#20224,#20225,#20226,#20227,#20228,#20229,#20230,#20231,#20232,
#20233,#20234,#20235,#20236,#20237,#20238,#20239,#20240,#20241,#20242,#20243,
#20244,#20245,#20246,#20247,#20248,#20249,#20250,#20251,#20252,#20253,#20254,
#20255,#20256,#20257,#20258,#20259,#20260,#20261,#20262,#20263,#20264,#20265,
#20266,#20267,#20268,#20269,#20270,#20271),.UNSPECIFIED.,.F.,.F.,(4,3,3,
3,3,3,3,3,3,3,3,3,3,3,3,3,3,3,4),(-0.376940817211661,-0.351602437644044,
-0.332519420023622,-0.318228069756221,-0.288333520013757,-0.272718137738777,
-0.234505390822111,-0.216962164313794,-0.205493431901863,-0.180854828870961,
-0.15373415812608,-0.13664282164838,-0.126205224016848,-0.0954715202702509,
-0.0666263326168646,-0.0558556424387309,-0.0219613030816618,-0.00327040903045922,
0.),.UNSPECIFIED.);
#2214=B_SPLINE_CURVE_WITH_KNOTS('',3,(#20273,#20274,#20275,#20276,#20277,
#20278,#20279,#20280,#20281,#20282,#20283),.UNSPECIFIED.,.F.,.F.,(4,1,1,
1,1,1,1,1,4),(15.7079632679489,15.8518654961884,16.8494368691713,17.8470082421543,
18.8445796151372,19.8421509881201,20.8397223611031,21.837293734086,21.9911485751285),
 .UNSPECIFIED.);
#2215=B_SPLINE_CURVE_WITH_KNOTS('',3,(#20284,#20285,#20286,#20287,#20288,
#20289,#20290,#20291,#20292,#20293),.UNSPECIFIED.,.F.,.F.,(4,1,1,1,1,1,
1,4),(15.7079632679489,16.3932837587428,17.3908551317257,18.3884265047087,
19.3859978776916,20.3835692506745,21.3811406236575,21.9911485751285),
 .UNSPECIFIED.);
#2216=B_SPLINE_CURVE_WITH_KNOTS('',3,(#20638,#20639,#20640,#20641,#20642,
#20643,#20644,#20645,#20646,#20647,#20648,#20649,#20650,#20651,#20652,#20653,
#20654,#20655,#20656,#20657,#20658,#20659,#20660,#20661,#20662,#20663,#20664,
#20665,#20666,#20667,#20668,#20669,#20670,#20671,#20672,#20673,#20674,#20675,
#20676,#20677,#20678,#20679,#20680,#20681,#20682,#20683,#20684,#20685,#20686,
#20687,#20688,#20689),.UNSPECIFIED.,.F.,.F.,(4,3,3,3,3,3,3,3,3,3,3,3,3,
3,3,3,3,4),(0.,0.0336910603093437,0.0587346556237836,0.0734852350726252,
0.109792229900142,0.132864814179886,0.143632001341265,0.177205256270027,
0.195912000411831,0.207613973950097,0.244895189457593,0.269599349217699,
0.282507794231336,0.310158230215905,0.327758387489592,0.342580257274108,
0.372940760482283,0.376940817211633),.UNSPECIFIED.);
#2217=B_SPLINE_CURVE_WITH_KNOTS('',3,(#20690,#20691,#20692,#20693,#20694,
#20695,#20696,#20697,#20698,#20699,#20700,#20701,#20702,#20703,#20704,#20705,
#20706,#20707,#20708,#20709,#20710,#20711,#20712,#20713,#20714),
 .UNSPECIFIED.,.F.,.F.,(4,3,3,3,3,3,3,3,4),(-10.1295685708718,-9.97571372982934,
-8.97814235684641,-7.98057098386347,-6.98299961088054,-5.9854282378976,
-4.98785686491467,-3.99028549193173,-3.84638326369226),.UNSPECIFIED.);
#2218=B_SPLINE_CURVE_WITH_KNOTS('',3,(#21059,#21060,#21061,#21062,#21063,
#21064,#21065,#21066,#21067,#21068,#21069,#21070,#21071,#21072,#21073,#21074,
#21075,#21076,#21077,#21078,#21079,#21080),.UNSPECIFIED.,.F.,.F.,(4,3,3,
3,3,3,3,4),(7.59300756235157,7.98057098386347,8.9781423568464,9.97571372982934,
10.9732851028123,11.9708564757952,12.9684278487781,13.8761928695311),
 .UNSPECIFIED.);
#2219=B_SPLINE_CURVE_WITH_KNOTS('',3,(#21081,#21082,#21083,#21084,#21085,
#21086,#21087,#21088,#21089,#21090,#21091,#21092,#21093,#21094,#21095,#21096,
#21097,#21098,#21099,#21100,#21101,#21102,#21103,#21104,#21105,#21106,#21107,
#21108,#21109,#21110,#21111,#21112,#21113,#21114,#21115,#21116,#21117,#21118,
#21119,#21120,#21121,#21122,#21123,#21124,#21125,#21126,#21127,#21128,#21129,
#21130,#21131,#21132),.UNSPECIFIED.,.F.,.F.,(4,3,3,3,3,3,3,3,3,3,3,3,3,
3,3,3,3,4),(0.,0.0396791507684394,0.0597938827984087,0.0771996525601983,
0.0898307615993676,0.128492920651297,0.153526877334627,0.165101563474246,
0.197163594226425,0.22445212238587,0.234160516714088,0.269455189460283,
0.287578726323234,0.30542148874616,0.333081540294033,0.34722488830939,0.375339207698871,
0.378621596831437),.UNSPECIFIED.);
#2220=B_SPLINE_CURVE_WITH_KNOTS('',3,(#21135,#21136,#21137,#21138,#21139,
#21140,#21141,#21142,#21143,#21144,#21145,#21146,#21147,#21148,#21149,#21150,
#21151,#21152,#21153,#21154,#21155,#21156,#21157,#21158,#21159,#21160,#21161,
#21162,#21163,#21164,#21165,#21166,#21167,#21168,#21169,#21170,#21171,#21172,
#21173,#21174,#21175,#21176,#21177,#21178,#21179,#21180,#21181,#21182,#21183,
#21184,#21185,#21186,#21187,#21188,#21189),.UNSPECIFIED.,.F.,.F.,(4,3,3,
3,3,3,3,3,3,3,3,3,3,3,3,3,3,3,4),(-0.378621596831443,-0.353562246091994,
-0.33972679327765,-0.324795398102486,-0.29996799510237,-0.289118738473772,
-0.252370061457217,-0.234474320899414,-0.219335629080767,-0.200829495678084,
-0.174827314232915,-0.155846896352443,-0.144923681945981,-0.109696914410712,
-0.0896698834676189,-0.0773386968783234,-0.0372142012245099,-0.00401661180490457,
0.),.UNSPECIFIED.);
#2221=B_SPLINE_CURVE_WITH_KNOTS('',3,(#21190,#21191,#21192,#21193,#21194,
#21195,#21196,#21197,#21198,#21199,#21200,#21201,#21202,#21203,#21204,#21205,
#21206,#21207,#21208,#21209,#21210,#21211,#21212,#21213,#21214,#21215,#21216,
#21217,#21218,#21219,#21220,#21221,#21222,#21223,#21224,#21225,#21226,#21227,
#21228,#21229,#21230,#21231,#21232,#21233,#21234,#21235,#21236,#21237,#21238,
#21239,#21240,#21241,#21242,#21243,#21244),.UNSPECIFIED.,.F.,.F.,(4,3,3,
3,3,3,3,3,3,3,3,3,3,3,3,3,3,3,4),(-0.376940817211611,-0.351602437357937,
-0.332519414484987,-0.318228064219006,-0.288333486347302,-0.272718127906801,
-0.234505384447309,-0.21696214863526,-0.205493420723107,-0.180854828870948,
-0.153734168647042,-0.136642926650914,-0.126205451446247,-0.0954716908423004,
-0.0666266083256078,-0.0558556962658209,-0.0219613612575045,-0.00327040903046154,
0.),.UNSPECIFIED.);
#2222=B_SPLINE_CURVE_WITH_KNOTS('',3,(#21246,#21247,#21248,#21249,#21250,
#21251,#21252,#21253,#21254,#21255,#21256),.UNSPECIFIED.,.F.,.F.,(4,1,1,
1,1,1,1,1,4),(15.7079632679489,15.8518654961884,16.8494368691714,17.8470082421543,
18.8445796151372,19.8421509881202,20.8397223611031,21.837293734086,21.9911485751285),
 .UNSPECIFIED.);
#2223=B_SPLINE_CURVE_WITH_KNOTS('',3,(#21257,#21258,#21259,#21260,#21261,
#21262,#21263,#21264,#21265,#21266),.UNSPECIFIED.,.F.,.F.,(4,1,1,1,1,1,
1,4),(15.7079632679489,16.3932837587428,17.3908551317257,18.3884265047087,
19.3859978776916,20.3835692506745,21.3811406236575,21.9911485751285),
 .UNSPECIFIED.);
#2224=B_SPLINE_CURVE_WITH_KNOTS('',3,(#21611,#21612,#21613,#21614,#21615,
#21616,#21617,#21618,#21619,#21620,#21621,#21622,#21623,#21624,#21625,#21626,
#21627,#21628,#21629,#21630,#21631,#21632,#21633,#21634,#21635,#21636,#21637,
#21638,#21639,#21640,#21641,#21642,#21643,#21644,#21645,#21646,#21647,#21648,
#21649,#21650,#21651,#21652,#21653,#21654,#21655,#21656,#21657,#21658,#21659,
#21660,#21661,#21662),.UNSPECIFIED.,.F.,.F.,(4,3,3,3,3,3,3,3,3,3,3,3,3,
3,3,3,3,4),(0.,0.0336910719722371,0.0587346603191241,0.0734852357557152,
0.109792234187795,0.132864822139093,0.143632015204812,0.177205256270034,
0.195911998811098,0.207613973107216,0.244895181060382,0.269599327917347,
0.282507776228681,0.310158203547799,0.327758105582494,0.342580213444175,
0.372940760482282,0.376940817211633),.UNSPECIFIED.);
#2225=B_SPLINE_CURVE_WITH_KNOTS('',3,(#21663,#21664,#21665,#21666,#21667,
#21668,#21669,#21670,#21671,#21672,#21673,#21674,#21675,#21676,#21677,#21678,
#21679,#21680,#21681,#21682,#21683,#21684,#21685,#21686,#21687),
 .UNSPECIFIED.,.F.,.F.,(4,3,3,3,3,3,3,3,4),(-10.1295685708718,-9.97571372982935,
-8.97814235684641,-7.98057098386348,-6.98299961088054,-5.98542823789761,
-4.98785686491467,-3.99028549193174,-3.84638326369226),.UNSPECIFIED.);
#2226=B_SPLINE_CURVE_WITH_KNOTS('',3,(#22032,#22033,#22034,#22035,#22036,
#22037,#22038,#22039,#22040,#22041,#22042,#22043,#22044,#22045,#22046,#22047,
#22048,#22049,#22050,#22051,#22052,#22053),.UNSPECIFIED.,.F.,.F.,(4,3,3,
3,3,3,3,4),(7.59300756235157,7.98057098386348,8.97814235684641,9.97571372982935,
10.9732851028123,11.9708564757952,12.9684278487782,13.8761928695311),
 .UNSPECIFIED.);
#2227=B_SPLINE_CURVE_WITH_KNOTS('',3,(#22054,#22055,#22056,#22057,#22058,
#22059,#22060,#22061,#22062,#22063,#22064,#22065,#22066,#22067,#22068,#22069,
#22070,#22071,#22072,#22073,#22074,#22075,#22076,#22077,#22078,#22079,#22080,
#22081,#22082,#22083,#22084,#22085,#22086,#22087,#22088,#22089,#22090,#22091,
#22092,#22093,#22094,#22095,#22096,#22097,#22098,#22099,#22100,#22101,#22102,
#22103,#22104,#22105),.UNSPECIFIED.,.F.,.F.,(4,3,3,3,3,3,3,3,3,3,3,3,3,
3,3,3,3,4),(0.,0.0396791274481056,0.0597937021224953,0.0771976680457239,
0.0898303082602208,0.12849248988162,0.15352646947755,0.165101472375799,
0.197163594226428,0.224452133325792,0.23416053148377,0.269455200537544,
0.287578557392714,0.305421521052156,0.333081636597174,0.347224904045167,
0.375339207698866,0.378621596831432),.UNSPECIFIED.);
#2830=LINE('',#14566,#3462);
#2831=LINE('',#14601,#3463);
#2832=LINE('',#14628,#3464);
#2833=LINE('',#14679,#3465);
#2834=LINE('',#14727,#3466);
#2835=LINE('',#14775,#3467);
#2836=LINE('',#14826,#3468);
#2837=LINE('',#14874,#3469);
#2838=LINE('',#14922,#3470);
#2839=LINE('',#14973,#3471);
#2840=LINE('',#15024,#3472);
#2841=LINE('',#15072,#3473);
#2842=LINE('',#15123,#3474);
#2843=LINE('',#15162,#3475);
#2844=LINE('',#15184,#3476);
#2845=LINE('',#15208,#3477);
#2846=LINE('',#15233,#3478);
#2847=LINE('',#15258,#3479);
#2848=LINE('',#15282,#3480);
#2849=LINE('',#15307,#3481);
#2850=LINE('',#15331,#3482);
#2851=LINE('',#15356,#3483);
#2852=LINE('',#15380,#3484);
#2853=LINE('',#15405,#3485);
#2854=LINE('',#15430,#3486);
#2855=LINE('',#15454,#3487);
#2856=LINE('',#15471,#3488);
#2857=LINE('',#15506,#3489);
#2858=LINE('',#15533,#3490);
#2859=LINE('',#15584,#3491);
#2860=LINE('',#15632,#3492);
#2861=LINE('',#15680,#3493);
#2862=LINE('',#15731,#3494);
#2863=LINE('',#15779,#3495);
#2864=LINE('',#15827,#3496);
#2865=LINE('',#15878,#3497);
#2866=LINE('',#15929,#3498);
#2867=LINE('',#15977,#3499);
#2868=LINE('',#16028,#3500);
#2869=LINE('',#16067,#3501);
#2870=LINE('',#16089,#3502);
#2871=LINE('',#16113,#3503);
#2872=LINE('',#16138,#3504);
#2873=LINE('',#16163,#3505);
#2874=LINE('',#16187,#3506);
#2875=LINE('',#16212,#3507);
#2876=LINE('',#16236,#3508);
#2877=LINE('',#16261,#3509);
#2878=LINE('',#16285,#3510);
#2879=LINE('',#16310,#3511);
#2880=LINE('',#16335,#3512);
#2881=LINE('',#16359,#3513);
#2882=LINE('',#16376,#3514);
#2883=LINE('',#16411,#3515);
#2884=LINE('',#16438,#3516);
#2885=LINE('',#16489,#3517);
#2886=LINE('',#16537,#3518);
#2887=LINE('',#16585,#3519);
#2888=LINE('',#16636,#3520);
#2889=LINE('',#16684,#3521);
#2890=LINE('',#16732,#3522);
#2891=LINE('',#16783,#3523);
#2892=LINE('',#16834,#3524);
#2893=LINE('',#16882,#3525);
#2894=LINE('',#16933,#3526);
#2895=LINE('',#16972,#3527);
#2896=LINE('',#16994,#3528);
#2897=LINE('',#17018,#3529);
#2898=LINE('',#17043,#3530);
#2899=LINE('',#17068,#3531);
#2900=LINE('',#17092,#3532);
#2901=LINE('',#17117,#3533);
#2902=LINE('',#17141,#3534);
#2903=LINE('',#17166,#3535);
#2904=LINE('',#17190,#3536);
#2905=LINE('',#17215,#3537);
#2906=LINE('',#17240,#3538);
#2907=LINE('',#17264,#3539);
#2908=LINE('',#17281,#3540);
#2909=LINE('',#17316,#3541);
#2910=LINE('',#17343,#3542);
#2911=LINE('',#17394,#3543);
#2912=LINE('',#17442,#3544);
#2913=LINE('',#17490,#3545);
#2914=LINE('',#17541,#3546);
#2915=LINE('',#17589,#3547);
#2916=LINE('',#17637,#3548);
#2917=LINE('',#17688,#3549);
#2918=LINE('',#17739,#3550);
#2919=LINE('',#17787,#3551);
#2920=LINE('',#17838,#3552);
#2921=LINE('',#17877,#3553);
#2922=LINE('',#17899,#3554);
#2923=LINE('',#17923,#3555);
#2924=LINE('',#17948,#3556);
#2925=LINE('',#17973,#3557);
#2926=LINE('',#17997,#3558);
#2927=LINE('',#18022,#3559);
#2928=LINE('',#18046,#3560);
#2929=LINE('',#18071,#3561);
#2930=LINE('',#18095,#3562);
#2931=LINE('',#18120,#3563);
#2932=LINE('',#18145,#3564);
#2933=LINE('',#18169,#3565);
#2934=LINE('',#18187,#3566);
#2935=LINE('',#18197,#3567);
#2936=LINE('',#18200,#3568);
#2937=LINE('',#18210,#3569);
#2938=LINE('',#18213,#3570);
#2939=LINE('',#22115,#3571);
#2940=LINE('',#22121,#3572);
#2941=LINE('',#22126,#3573);
#2942=LINE('',#22128,#3574);
#2943=LINE('',#22130,#3575);
#2944=LINE('',#22131,#3576);
#2945=LINE('',#22134,#3577);
#2946=LINE('',#22136,#3578);
#2947=LINE('',#22137,#3579);
#2948=LINE('',#22140,#3580);
#2949=LINE('',#22142,#3581);
#2950=LINE('',#22143,#3582);
#2951=LINE('',#22145,#3583);
#2952=LINE('',#22149,#3584);
#2953=LINE('',#22151,#3585);
#2954=LINE('',#22153,#3586);
#2955=LINE('',#22154,#3587);
#2956=LINE('',#22158,#3588);
#2957=LINE('',#22160,#3589);
#2958=LINE('',#22162,#3590);
#2959=LINE('',#22163,#3591);
#2960=LINE('',#22165,#3592);
#2961=LINE('',#22166,#3593);
#2962=LINE('',#22168,#3594);
#2963=LINE('',#22173,#3595);
#2964=LINE('',#22179,#3596);
#2965=LINE('',#22187,#3597);
#2966=LINE('',#22191,#3598);
#2967=LINE('',#22195,#3599);
#2968=LINE('',#22198,#3600);
#2969=LINE('',#22201,#3601);
#2970=LINE('',#22204,#3602);
#2971=LINE('',#22207,#3603);
#2972=LINE('',#22208,#3604);
#2973=LINE('',#22211,#3605);
#2974=LINE('',#22215,#3606);
#2975=LINE('',#22216,#3607);
#2976=LINE('',#22219,#3608);
#2977=LINE('',#22222,#3609);
#2978=LINE('',#22226,#3610);
#2979=LINE('',#22227,#3611);
#2980=LINE('',#22231,#3612);
#2981=LINE('',#22235,#3613);
#2982=LINE('',#22237,#3614);
#2983=LINE('',#22239,#3615);
#2984=LINE('',#22240,#3616);
#2985=LINE('',#22242,#3617);
#2986=LINE('',#22244,#3618);
#2987=LINE('',#22246,#3619);
#2988=LINE('',#22247,#3620);
#2989=LINE('',#22250,#3621);
#2990=LINE('',#22252,#3622);
#2991=LINE('',#22253,#3623);
#2992=LINE('',#22255,#3624);
#2993=LINE('',#22256,#3625);
#2994=LINE('',#22257,#3626);
#3462=VECTOR('',#12273,0.2);
#3463=VECTOR('',#12276,0.2);
#3464=VECTOR('',#12281,0.2);
#3465=VECTOR('',#12284,0.2);
#3466=VECTOR('',#12287,0.2);
#3467=VECTOR('',#12290,0.2);
#3468=VECTOR('',#12293,0.2);
#3469=VECTOR('',#12296,0.2);
#3470=VECTOR('',#12299,0.2);
#3471=VECTOR('',#12302,0.2);
#3472=VECTOR('',#12305,0.2);
#3473=VECTOR('',#12308,0.2);
#3474=VECTOR('',#12311,0.2);
#3475=VECTOR('',#12316,0.205475000000001);
#3476=VECTOR('',#12321,0.205475000000001);
#3477=VECTOR('',#12324,0.205475000000001);
#3478=VECTOR('',#12327,0.205475000000001);
#3479=VECTOR('',#12330,0.205475000000001);
#3480=VECTOR('',#12333,0.205475000000001);
#3481=VECTOR('',#12336,0.205475000000001);
#3482=VECTOR('',#12339,0.205475000000001);
#3483=VECTOR('',#12342,0.205475000000001);
#3484=VECTOR('',#12345,0.205475000000001);
#3485=VECTOR('',#12348,0.205475000000001);
#3486=VECTOR('',#12351,0.205475000000001);
#3487=VECTOR('',#12354,0.205475000000001);
#3488=VECTOR('',#12359,0.2);
#3489=VECTOR('',#12362,0.2);
#3490=VECTOR('',#12367,0.2);
#3491=VECTOR('',#12370,0.2);
#3492=VECTOR('',#12373,0.2);
#3493=VECTOR('',#12376,0.2);
#3494=VECTOR('',#12379,0.2);
#3495=VECTOR('',#12382,0.2);
#3496=VECTOR('',#12385,0.2);
#3497=VECTOR('',#12388,0.2);
#3498=VECTOR('',#12391,0.2);
#3499=VECTOR('',#12394,0.2);
#3500=VECTOR('',#12397,0.2);
#3501=VECTOR('',#12402,0.205475000000001);
#3502=VECTOR('',#12407,0.205475000000001);
#3503=VECTOR('',#12410,0.205475000000001);
#3504=VECTOR('',#12413,0.205475000000001);
#3505=VECTOR('',#12416,0.205475000000001);
#3506=VECTOR('',#12419,0.205475000000001);
#3507=VECTOR('',#12422,0.205475000000001);
#3508=VECTOR('',#12425,0.205475000000001);
#3509=VECTOR('',#12428,0.205475000000001);
#3510=VECTOR('',#12431,0.205475000000001);
#3511=VECTOR('',#12434,0.205475000000001);
#3512=VECTOR('',#12437,0.205475000000001);
#3513=VECTOR('',#12440,0.205475000000001);
#3514=VECTOR('',#12445,0.2);
#3515=VECTOR('',#12448,0.2);
#3516=VECTOR('',#12453,0.2);
#3517=VECTOR('',#12456,0.2);
#3518=VECTOR('',#12459,0.2);
#3519=VECTOR('',#12462,0.2);
#3520=VECTOR('',#12465,0.2);
#3521=VECTOR('',#12468,0.2);
#3522=VECTOR('',#12471,0.2);
#3523=VECTOR('',#12474,0.2);
#3524=VECTOR('',#12477,0.2);
#3525=VECTOR('',#12480,0.2);
#3526=VECTOR('',#12483,0.2);
#3527=VECTOR('',#12488,0.205475);
#3528=VECTOR('',#12493,0.205475);
#3529=VECTOR('',#12496,0.205475);
#3530=VECTOR('',#12499,0.205475);
#3531=VECTOR('',#12502,0.205475);
#3532=VECTOR('',#12505,0.205475);
#3533=VECTOR('',#12508,0.205475);
#3534=VECTOR('',#12511,0.205475);
#3535=VECTOR('',#12514,0.205475);
#3536=VECTOR('',#12517,0.205475);
#3537=VECTOR('',#12520,0.205475);
#3538=VECTOR('',#12523,0.205475);
#3539=VECTOR('',#12526,0.205475);
#3540=VECTOR('',#12531,0.2);
#3541=VECTOR('',#12534,0.2);
#3542=VECTOR('',#12539,0.2);
#3543=VECTOR('',#12542,0.2);
#3544=VECTOR('',#12545,0.2);
#3545=VECTOR('',#12548,0.2);
#3546=VECTOR('',#12551,0.2);
#3547=VECTOR('',#12554,0.2);
#3548=VECTOR('',#12557,0.2);
#3549=VECTOR('',#12560,0.2);
#3550=VECTOR('',#12563,0.2);
#3551=VECTOR('',#12566,0.2);
#3552=VECTOR('',#12569,0.2);
#3553=VECTOR('',#12574,0.205475);
#3554=VECTOR('',#12579,0.205475);
#3555=VECTOR('',#12582,0.205475);
#3556=VECTOR('',#12585,0.205475);
#3557=VECTOR('',#12588,0.205475);
#3558=VECTOR('',#12591,0.205475);
#3559=VECTOR('',#12594,0.205475);
#3560=VECTOR('',#12597,0.205475);
#3561=VECTOR('',#12600,0.205475);
#3562=VECTOR('',#12603,0.205475);
#3563=VECTOR('',#12606,0.205475);
#3564=VECTOR('',#12609,0.205475);
#3565=VECTOR('',#12612,0.205475);
#3566=VECTOR('',#12619,0.6);
#3567=VECTOR('',#12632,0.4);
#3568=VECTOR('',#12635,0.25);
#3569=VECTOR('',#12648,0.4);
#3570=VECTOR('',#12651,0.25);
#3571=VECTOR('',#12690,0.3);
#3572=VECTOR('',#12697,0.3);
#3573=VECTOR('',#12702,1.);
#3574=VECTOR('',#12703,1.);
#3575=VECTOR('',#12704,1.);
#3576=VECTOR('',#12705,1.);
#3577=VECTOR('',#12708,1.);
#3578=VECTOR('',#12709,1.);
#3579=VECTOR('',#12710,1.);
#3580=VECTOR('',#12713,1.);
#3581=VECTOR('',#12714,1.);
#3582=VECTOR('',#12715,1.);
#3583=VECTOR('',#12718,1.);
#3584=VECTOR('',#12721,1.);
#3585=VECTOR('',#12722,1.);
#3586=VECTOR('',#12723,1.);
#3587=VECTOR('',#12724,1.);
#3588=VECTOR('',#12727,1.);
#3589=VECTOR('',#12728,1.);
#3590=VECTOR('',#12729,1.);
#3591=VECTOR('',#12730,1.);
#3592=VECTOR('',#12733,1.);
#3593=VECTOR('',#12734,1.);
#3594=VECTOR('',#12737,1.);
#3595=VECTOR('',#12742,0.65);
#3596=VECTOR('',#12749,0.8);
#3597=VECTOR('',#12758,1.);
#3598=VECTOR('',#12761,1.);
#3599=VECTOR('',#12764,1.);
#3600=VECTOR('',#12767,1.);
#3601=VECTOR('',#12770,1.);
#3602=VECTOR('',#12773,1.);
#3603=VECTOR('',#12776,1.);
#3604=VECTOR('',#12777,1.);
#3605=VECTOR('',#12780,1.);
#3606=VECTOR('',#12785,1.);
#3607=VECTOR('',#12786,1.);
#3608=VECTOR('',#12789,1.);
#3609=VECTOR('',#12792,1.);
#3610=VECTOR('',#12797,1.);
#3611=VECTOR('',#12798,1.);
#3612=VECTOR('',#12805,1.);
#3613=VECTOR('',#12808,1.);
#3614=VECTOR('',#12809,1.);
#3615=VECTOR('',#12810,1.);
#3616=VECTOR('',#12811,1.);
#3617=VECTOR('',#12814,1.);
#3618=VECTOR('',#12815,1.);
#3619=VECTOR('',#12816,1.);
#3620=VECTOR('',#12817,1.);
#3621=VECTOR('',#12820,1.);
#3622=VECTOR('',#12821,1.);
#3623=VECTOR('',#12822,1.);
#3624=VECTOR('',#12825,1.);
#3625=VECTOR('',#12826,1.);
#3626=VECTOR('',#12827,1.);
#4094=VERTEX_POINT('',#14564);
#4095=VERTEX_POINT('',#14565);
#4096=VERTEX_POINT('',#14567);
#4097=VERTEX_POINT('',#14590);
#4098=VERTEX_POINT('',#14592);
#4099=VERTEX_POINT('',#14600);
#4100=VERTEX_POINT('',#14626);
#4101=VERTEX_POINT('',#14627);
#4102=VERTEX_POINT('',#14677);
#4103=VERTEX_POINT('',#14678);
#4104=VERTEX_POINT('',#14725);
#4105=VERTEX_POINT('',#14726);
#4106=VERTEX_POINT('',#14773);
#4107=VERTEX_POINT('',#14774);
#4108=VERTEX_POINT('',#14824);
#4109=VERTEX_POINT('',#14825);
#4110=VERTEX_POINT('',#14872);
#4111=VERTEX_POINT('',#14873);
#4112=VERTEX_POINT('',#14920);
#4113=VERTEX_POINT('',#14921);
#4114=VERTEX_POINT('',#14971);
#4115=VERTEX_POINT('',#14972);
#4116=VERTEX_POINT('',#15022);
#4117=VERTEX_POINT('',#15023);
#4118=VERTEX_POINT('',#15070);
#4119=VERTEX_POINT('',#15071);
#4120=VERTEX_POINT('',#15121);
#4121=VERTEX_POINT('',#15122);
#4122=VERTEX_POINT('',#15124);
#4123=VERTEX_POINT('',#15138);
#4124=VERTEX_POINT('',#15160);
#4125=VERTEX_POINT('',#15161);
#4126=VERTEX_POINT('',#15163);
#4127=VERTEX_POINT('',#15171);
#4128=VERTEX_POINT('',#15182);
#4129=VERTEX_POINT('',#15183);
#4130=VERTEX_POINT('',#15206);
#4131=VERTEX_POINT('',#15207);
#4132=VERTEX_POINT('',#15231);
#4133=VERTEX_POINT('',#15232);
#4134=VERTEX_POINT('',#15256);
#4135=VERTEX_POINT('',#15257);
#4136=VERTEX_POINT('',#15280);
#4137=VERTEX_POINT('',#15281);
#4138=VERTEX_POINT('',#15305);
#4139=VERTEX_POINT('',#15306);
#4140=VERTEX_POINT('',#15329);
#4141=VERTEX_POINT('',#15330);
#4142=VERTEX_POINT('',#15354);
#4143=VERTEX_POINT('',#15355);
#4144=VERTEX_POINT('',#15378);
#4145=VERTEX_POINT('',#15379);
#4146=VERTEX_POINT('',#15403);
#4147=VERTEX_POINT('',#15404);
#4148=VERTEX_POINT('',#15428);
#4149=VERTEX_POINT('',#15429);
#4150=VERTEX_POINT('',#15452);
#4151=VERTEX_POINT('',#15453);
#4152=VERTEX_POINT('',#15455);
#4153=VERTEX_POINT('',#15461);
#4154=VERTEX_POINT('',#15469);
#4155=VERTEX_POINT('',#15470);
#4156=VERTEX_POINT('',#15472);
#4157=VERTEX_POINT('',#15495);
#4158=VERTEX_POINT('',#15497);
#4159=VERTEX_POINT('',#15505);
#4160=VERTEX_POINT('',#15531);
#4161=VERTEX_POINT('',#15532);
#4162=VERTEX_POINT('',#15582);
#4163=VERTEX_POINT('',#15583);
#4164=VERTEX_POINT('',#15630);
#4165=VERTEX_POINT('',#15631);
#4166=VERTEX_POINT('',#15678);
#4167=VERTEX_POINT('',#15679);
#4168=VERTEX_POINT('',#15729);
#4169=VERTEX_POINT('',#15730);
#4170=VERTEX_POINT('',#15777);
#4171=VERTEX_POINT('',#15778);
#4172=VERTEX_POINT('',#15825);
#4173=VERTEX_POINT('',#15826);
#4174=VERTEX_POINT('',#15876);
#4175=VERTEX_POINT('',#15877);
#4176=VERTEX_POINT('',#15927);
#4177=VERTEX_POINT('',#15928);
#4178=VERTEX_POINT('',#15975);
#4179=VERTEX_POINT('',#15976);
#4180=VERTEX_POINT('',#16026);
#4181=VERTEX_POINT('',#16027);
#4182=VERTEX_POINT('',#16029);
#4183=VERTEX_POINT('',#16043);
#4184=VERTEX_POINT('',#16065);
#4185=VERTEX_POINT('',#16066);
#4186=VERTEX_POINT('',#16068);
#4187=VERTEX_POINT('',#16076);
#4188=VERTEX_POINT('',#16087);
#4189=VERTEX_POINT('',#16088);
#4190=VERTEX_POINT('',#16111);
#4191=VERTEX_POINT('',#16112);
#4192=VERTEX_POINT('',#16136);
#4193=VERTEX_POINT('',#16137);
#4194=VERTEX_POINT('',#16161);
#4195=VERTEX_POINT('',#16162);
#4196=VERTEX_POINT('',#16185);
#4197=VERTEX_POINT('',#16186);
#4198=VERTEX_POINT('',#16210);
#4199=VERTEX_POINT('',#16211);
#4200=VERTEX_POINT('',#16234);
#4201=VERTEX_POINT('',#16235);
#4202=VERTEX_POINT('',#16259);
#4203=VERTEX_POINT('',#16260);
#4204=VERTEX_POINT('',#16283);
#4205=VERTEX_POINT('',#16284);
#4206=VERTEX_POINT('',#16308);
#4207=VERTEX_POINT('',#16309);
#4208=VERTEX_POINT('',#16333);
#4209=VERTEX_POINT('',#16334);
#4210=VERTEX_POINT('',#16357);
#4211=VERTEX_POINT('',#16358);
#4212=VERTEX_POINT('',#16360);
#4213=VERTEX_POINT('',#16366);
#4214=VERTEX_POINT('',#16374);
#4215=VERTEX_POINT('',#16375);
#4216=VERTEX_POINT('',#16377);
#4217=VERTEX_POINT('',#16400);
#4218=VERTEX_POINT('',#16402);
#4219=VERTEX_POINT('',#16410);
#4220=VERTEX_POINT('',#16436);
#4221=VERTEX_POINT('',#16437);
#4222=VERTEX_POINT('',#16487);
#4223=VERTEX_POINT('',#16488);
#4224=VERTEX_POINT('',#16535);
#4225=VERTEX_POINT('',#16536);
#4226=VERTEX_POINT('',#16583);
#4227=VERTEX_POINT('',#16584);
#4228=VERTEX_POINT('',#16634);
#4229=VERTEX_POINT('',#16635);
#4230=VERTEX_POINT('',#16682);
#4231=VERTEX_POINT('',#16683);
#4232=VERTEX_POINT('',#16730);
#4233=VERTEX_POINT('',#16731);
#4234=VERTEX_POINT('',#16781);
#4235=VERTEX_POINT('',#16782);
#4236=VERTEX_POINT('',#16832);
#4237=VERTEX_POINT('',#16833);
#4238=VERTEX_POINT('',#16880);
#4239=VERTEX_POINT('',#16881);
#4240=VERTEX_POINT('',#16931);
#4241=VERTEX_POINT('',#16932);
#4242=VERTEX_POINT('',#16934);
#4243=VERTEX_POINT('',#16948);
#4244=VERTEX_POINT('',#16970);
#4245=VERTEX_POINT('',#16971);
#4246=VERTEX_POINT('',#16973);
#4247=VERTEX_POINT('',#16981);
#4248=VERTEX_POINT('',#16992);
#4249=VERTEX_POINT('',#16993);
#4250=VERTEX_POINT('',#17016);
#4251=VERTEX_POINT('',#17017);
#4252=VERTEX_POINT('',#17041);
#4253=VERTEX_POINT('',#17042);
#4254=VERTEX_POINT('',#17066);
#4255=VERTEX_POINT('',#17067);
#4256=VERTEX_POINT('',#17090);
#4257=VERTEX_POINT('',#17091);
#4258=VERTEX_POINT('',#17115);
#4259=VERTEX_POINT('',#17116);
#4260=VERTEX_POINT('',#17139);
#4261=VERTEX_POINT('',#17140);
#4262=VERTEX_POINT('',#17164);
#4263=VERTEX_POINT('',#17165);
#4264=VERTEX_POINT('',#17188);
#4265=VERTEX_POINT('',#17189);
#4266=VERTEX_POINT('',#17213);
#4267=VERTEX_POINT('',#17214);
#4268=VERTEX_POINT('',#17238);
#4269=VERTEX_POINT('',#17239);
#4270=VERTEX_POINT('',#17262);
#4271=VERTEX_POINT('',#17263);
#4272=VERTEX_POINT('',#17265);
#4273=VERTEX_POINT('',#17271);
#4274=VERTEX_POINT('',#17279);
#4275=VERTEX_POINT('',#17280);
#4276=VERTEX_POINT('',#17282);
#4277=VERTEX_POINT('',#17305);
#4278=VERTEX_POINT('',#17307);
#4279=VERTEX_POINT('',#17315);
#4280=VERTEX_POINT('',#17341);
#4281=VERTEX_POINT('',#17342);
#4282=VERTEX_POINT('',#17392);
#4283=VERTEX_POINT('',#17393);
#4284=VERTEX_POINT('',#17440);
#4285=VERTEX_POINT('',#17441);
#4286=VERTEX_POINT('',#17488);
#4287=VERTEX_POINT('',#17489);
#4288=VERTEX_POINT('',#17539);
#4289=VERTEX_POINT('',#17540);
#4290=VERTEX_POINT('',#17587);
#4291=VERTEX_POINT('',#17588);
#4292=VERTEX_POINT('',#17635);
#4293=VERTEX_POINT('',#17636);
#4294=VERTEX_POINT('',#17686);
#4295=VERTEX_POINT('',#17687);
#4296=VERTEX_POINT('',#17737);
#4297=VERTEX_POINT('',#17738);
#4298=VERTEX_POINT('',#17785);
#4299=VERTEX_POINT('',#17786);
#4300=VERTEX_POINT('',#17836);
#4301=VERTEX_POINT('',#17837);
#4302=VERTEX_POINT('',#17839);
#4303=VERTEX_POINT('',#17853);
#4304=VERTEX_POINT('',#17875);
#4305=VERTEX_POINT('',#17876);
#4306=VERTEX_POINT('',#17878);
#4307=VERTEX_POINT('',#17886);
#4308=VERTEX_POINT('',#17897);
#4309=VERTEX_POINT('',#17898);
#4310=VERTEX_POINT('',#17921);
#4311=VERTEX_POINT('',#17922);
#4312=VERTEX_POINT('',#17946);
#4313=VERTEX_POINT('',#17947);
#4314=VERTEX_POINT('',#17971);
#4315=VERTEX_POINT('',#17972);
#4316=VERTEX_POINT('',#17995);
#4317=VERTEX_POINT('',#17996);
#4318=VERTEX_POINT('',#18020);
#4319=VERTEX_POINT('',#18021);
#4320=VERTEX_POINT('',#18044);
#4321=VERTEX_POINT('',#18045);
#4322=VERTEX_POINT('',#18069);
#4323=VERTEX_POINT('',#18070);
#4324=VERTEX_POINT('',#18093);
#4325=VERTEX_POINT('',#18094);
#4326=VERTEX_POINT('',#18118);
#4327=VERTEX_POINT('',#18119);
#4328=VERTEX_POINT('',#18143);
#4329=VERTEX_POINT('',#18144);
#4330=VERTEX_POINT('',#18167);
#4331=VERTEX_POINT('',#18168);
#4332=VERTEX_POINT('',#18170);
#4333=VERTEX_POINT('',#18176);
#4334=VERTEX_POINT('',#18184);
#4335=VERTEX_POINT('',#18186);
#4336=VERTEX_POINT('',#18190);
#4337=VERTEX_POINT('',#18192);
#4338=VERTEX_POINT('',#18195);
#4339=VERTEX_POINT('',#18199);
#4340=VERTEX_POINT('',#18203);
#4341=VERTEX_POINT('',#18205);
#4342=VERTEX_POINT('',#18208);
#4343=VERTEX_POINT('',#18212);
#4344=VERTEX_POINT('',#22112);
#4345=VERTEX_POINT('',#22114);
#4346=VERTEX_POINT('',#22118);
#4347=VERTEX_POINT('',#22120);
#4348=VERTEX_POINT('',#22124);
#4349=VERTEX_POINT('',#22125);
#4350=VERTEX_POINT('',#22127);
#4351=VERTEX_POINT('',#22129);
#4352=VERTEX_POINT('',#22133);
#4353=VERTEX_POINT('',#22135);
#4354=VERTEX_POINT('',#22139);
#4355=VERTEX_POINT('',#22141);
#4356=VERTEX_POINT('',#22147);
#4357=VERTEX_POINT('',#22148);
#4358=VERTEX_POINT('',#22150);
#4359=VERTEX_POINT('',#22152);
#4360=VERTEX_POINT('',#22156);
#4361=VERTEX_POINT('',#22157);
#4362=VERTEX_POINT('',#22159);
#4363=VERTEX_POINT('',#22161);
#4364=VERTEX_POINT('',#22170);
#4365=VERTEX_POINT('',#22172);
#4366=VERTEX_POINT('',#22176);
#4367=VERTEX_POINT('',#22178);
#4368=VERTEX_POINT('',#22183);
#4369=VERTEX_POINT('',#22184);
#4370=VERTEX_POINT('',#22186);
#4371=VERTEX_POINT('',#22188);
#4372=VERTEX_POINT('',#22190);
#4373=VERTEX_POINT('',#22192);
#4374=VERTEX_POINT('',#22194);
#4375=VERTEX_POINT('',#22196);
#4376=VERTEX_POINT('',#22200);
#4377=VERTEX_POINT('',#22202);
#4378=VERTEX_POINT('',#22206);
#4379=VERTEX_POINT('',#22210);
#4380=VERTEX_POINT('',#22214);
#4381=VERTEX_POINT('',#22218);
#4382=VERTEX_POINT('',#22220);
#4383=VERTEX_POINT('',#22225);
#4384=VERTEX_POINT('',#22233);
#4385=VERTEX_POINT('',#22234);
#4386=VERTEX_POINT('',#22236);
#4387=VERTEX_POINT('',#22238);
#4388=VERTEX_POINT('',#22243);
#4389=VERTEX_POINT('',#22245);
#4390=VERTEX_POINT('',#22249);
#4391=VERTEX_POINT('',#22251);
#5200=EDGE_CURVE('',#4094,#4095,#2830,.T.);
#5201=EDGE_CURVE('',#4095,#4096,#1992,.T.);
#5202=EDGE_CURVE('',#4096,#4097,#1801,.T.);
#5203=EDGE_CURVE('',#4097,#4098,#1993,.T.);
#5204=EDGE_CURVE('',#4098,#4099,#2831,.T.);
#5205=EDGE_CURVE('',#4099,#4099,#1802,.F.);
#5206=EDGE_CURVE('',#4098,#4094,#1994,.T.);
#5207=EDGE_CURVE('',#4100,#4101,#2832,.T.);
#5208=EDGE_CURVE('',#4101,#4095,#1995,.T.);
#5209=EDGE_CURVE('',#4094,#4100,#1996,.T.);
#5210=EDGE_CURVE('',#4102,#4103,#2833,.T.);
#5211=EDGE_CURVE('',#4103,#4101,#1997,.T.);
#5212=EDGE_CURVE('',#4100,#4102,#1998,.T.);
#5213=EDGE_CURVE('',#4104,#4105,#2834,.T.);
#5214=EDGE_CURVE('',#4105,#4103,#1999,.T.);
#5215=EDGE_CURVE('',#4102,#4104,#2000,.T.);
#5216=EDGE_CURVE('',#4106,#4107,#2835,.T.);
#5217=EDGE_CURVE('',#4107,#4105,#2001,.T.);
#5218=EDGE_CURVE('',#4104,#4106,#2002,.T.);
#5219=EDGE_CURVE('',#4108,#4109,#2836,.T.);
#5220=EDGE_CURVE('',#4109,#4107,#2003,.T.);
#5221=EDGE_CURVE('',#4106,#4108,#2004,.T.);
#5222=EDGE_CURVE('',#4110,#4111,#2837,.T.);
#5223=EDGE_CURVE('',#4111,#4109,#2005,.T.);
#5224=EDGE_CURVE('',#4108,#4110,#2006,.T.);
#5225=EDGE_CURVE('',#4112,#4113,#2838,.T.);
#5226=EDGE_CURVE('',#4113,#4111,#2007,.T.);
#5227=EDGE_CURVE('',#4110,#4112,#2008,.T.);
#5228=EDGE_CURVE('',#4114,#4115,#2839,.T.);
#5229=EDGE_CURVE('',#4115,#4113,#2009,.T.);
#5230=EDGE_CURVE('',#4112,#4114,#2010,.T.);
#5231=EDGE_CURVE('',#4116,#4117,#2840,.T.);
#5232=EDGE_CURVE('',#4117,#4115,#2011,.T.);
#5233=EDGE_CURVE('',#4114,#4116,#2012,.T.);
#5234=EDGE_CURVE('',#4118,#4119,#2841,.T.);
#5235=EDGE_CURVE('',#4119,#4117,#2013,.T.);
#5236=EDGE_CURVE('',#4116,#4118,#2014,.T.);
#5237=EDGE_CURVE('',#4120,#4121,#2842,.T.);
#5238=EDGE_CURVE('',#4120,#4122,#2015,.T.);
#5239=EDGE_CURVE('',#4123,#4122,#1803,.T.);
#5240=EDGE_CURVE('',#4123,#4121,#2016,.T.);
#5241=EDGE_CURVE('',#4124,#4125,#2843,.T.);
#5242=EDGE_CURVE('',#4125,#4126,#2017,.T.);
#5243=EDGE_CURVE('',#4127,#4126,#1804,.T.);
#5244=EDGE_CURVE('',#4124,#4127,#2018,.T.);
#5245=EDGE_CURVE('',#4128,#4129,#2844,.T.);
#5246=EDGE_CURVE('',#4129,#4125,#2019,.T.);
#5247=EDGE_CURVE('',#4128,#4124,#2020,.T.);
#5248=EDGE_CURVE('',#4130,#4131,#2845,.T.);
#5249=EDGE_CURVE('',#4131,#4129,#2021,.T.);
#5250=EDGE_CURVE('',#4130,#4128,#2022,.T.);
#5251=EDGE_CURVE('',#4132,#4133,#2846,.T.);
#5252=EDGE_CURVE('',#4133,#4131,#2023,.T.);
#5253=EDGE_CURVE('',#4132,#4130,#2024,.T.);
#5254=EDGE_CURVE('',#4134,#4135,#2847,.T.);
#5255=EDGE_CURVE('',#4135,#4133,#2025,.T.);
#5256=EDGE_CURVE('',#4134,#4132,#2026,.T.);
#5257=EDGE_CURVE('',#4136,#4137,#2848,.T.);
#5258=EDGE_CURVE('',#4137,#4135,#2027,.T.);
#5259=EDGE_CURVE('',#4136,#4134,#2028,.T.);
#5260=EDGE_CURVE('',#4138,#4139,#2849,.T.);
#5261=EDGE_CURVE('',#4139,#4137,#2029,.T.);
#5262=EDGE_CURVE('',#4138,#4136,#2030,.T.);
#5263=EDGE_CURVE('',#4140,#4141,#2850,.T.);
#5264=EDGE_CURVE('',#4141,#4139,#2031,.T.);
#5265=EDGE_CURVE('',#4140,#4138,#2032,.T.);
#5266=EDGE_CURVE('',#4142,#4143,#2851,.T.);
#5267=EDGE_CURVE('',#4143,#4141,#2033,.T.);
#5268=EDGE_CURVE('',#4142,#4140,#2034,.T.);
#5269=EDGE_CURVE('',#4144,#4145,#2852,.T.);
#5270=EDGE_CURVE('',#4145,#4143,#2035,.T.);
#5271=EDGE_CURVE('',#4144,#4142,#2036,.T.);
#5272=EDGE_CURVE('',#4146,#4147,#2853,.T.);
#5273=EDGE_CURVE('',#4147,#4145,#2037,.T.);
#5274=EDGE_CURVE('',#4146,#4144,#2038,.T.);
#5275=EDGE_CURVE('',#4148,#4149,#2854,.T.);
#5276=EDGE_CURVE('',#4149,#4147,#2039,.T.);
#5277=EDGE_CURVE('',#4148,#4146,#2040,.T.);
#5278=EDGE_CURVE('',#4150,#4151,#2855,.T.);
#5279=EDGE_CURVE('',#4152,#4150,#2041,.T.);
#5280=EDGE_CURVE('',#4153,#4152,#1805,.T.);
#5281=EDGE_CURVE('',#4153,#4151,#2042,.T.);
#5282=EDGE_CURVE('',#4154,#4155,#2856,.T.);
#5283=EDGE_CURVE('',#4155,#4156,#2043,.T.);
#5284=EDGE_CURVE('',#4156,#4157,#1806,.T.);
#5285=EDGE_CURVE('',#4157,#4158,#2044,.T.);
#5286=EDGE_CURVE('',#4158,#4159,#2857,.T.);
#5287=EDGE_CURVE('',#4159,#4159,#1807,.F.);
#5288=EDGE_CURVE('',#4158,#4154,#2045,.T.);
#5289=EDGE_CURVE('',#4160,#4161,#2858,.T.);
#5290=EDGE_CURVE('',#4161,#4155,#2046,.T.);
#5291=EDGE_CURVE('',#4154,#4160,#2047,.T.);
#5292=EDGE_CURVE('',#4162,#4163,#2859,.T.);
#5293=EDGE_CURVE('',#4163,#4161,#2048,.T.);
#5294=EDGE_CURVE('',#4160,#4162,#2049,.T.);
#5295=EDGE_CURVE('',#4164,#4165,#2860,.T.);
#5296=EDGE_CURVE('',#4165,#4163,#2050,.T.);
#5297=EDGE_CURVE('',#4162,#4164,#2051,.T.);
#5298=EDGE_CURVE('',#4166,#4167,#2861,.T.);
#5299=EDGE_CURVE('',#4167,#4165,#2052,.T.);
#5300=EDGE_CURVE('',#4164,#4166,#2053,.T.);
#5301=EDGE_CURVE('',#4168,#4169,#2862,.T.);
#5302=EDGE_CURVE('',#4169,#4167,#2054,.T.);
#5303=EDGE_CURVE('',#4166,#4168,#2055,.T.);
#5304=EDGE_CURVE('',#4170,#4171,#2863,.T.);
#5305=EDGE_CURVE('',#4171,#4169,#2056,.T.);
#5306=EDGE_CURVE('',#4168,#4170,#2057,.T.);
#5307=EDGE_CURVE('',#4172,#4173,#2864,.T.);
#5308=EDGE_CURVE('',#4173,#4171,#2058,.T.);
#5309=EDGE_CURVE('',#4170,#4172,#2059,.T.);
#5310=EDGE_CURVE('',#4174,#4175,#2865,.T.);
#5311=EDGE_CURVE('',#4175,#4173,#2060,.T.);
#5312=EDGE_CURVE('',#4172,#4174,#2061,.T.);
#5313=EDGE_CURVE('',#4176,#4177,#2866,.T.);
#5314=EDGE_CURVE('',#4177,#4175,#2062,.T.);
#5315=EDGE_CURVE('',#4174,#4176,#2063,.T.);
#5316=EDGE_CURVE('',#4178,#4179,#2867,.T.);
#5317=EDGE_CURVE('',#4179,#4177,#2064,.T.);
#5318=EDGE_CURVE('',#4176,#4178,#2065,.T.);
#5319=EDGE_CURVE('',#4180,#4181,#2868,.T.);
#5320=EDGE_CURVE('',#4180,#4182,#2066,.T.);
#5321=EDGE_CURVE('',#4183,#4182,#1808,.T.);
#5322=EDGE_CURVE('',#4183,#4181,#2067,.T.);
#5323=EDGE_CURVE('',#4184,#4185,#2869,.T.);
#5324=EDGE_CURVE('',#4185,#4186,#2068,.T.);
#5325=EDGE_CURVE('',#4187,#4186,#1809,.T.);
#5326=EDGE_CURVE('',#4184,#4187,#2069,.T.);
#5327=EDGE_CURVE('',#4188,#4189,#2870,.T.);
#5328=EDGE_CURVE('',#4189,#4185,#2070,.T.);
#5329=EDGE_CURVE('',#4188,#4184,#2071,.T.);
#5330=EDGE_CURVE('',#4190,#4191,#2871,.T.);
#5331=EDGE_CURVE('',#4191,#4189,#2072,.T.);
#5332=EDGE_CURVE('',#4190,#4188,#2073,.T.);
#5333=EDGE_CURVE('',#4192,#4193,#2872,.T.);
#5334=EDGE_CURVE('',#4193,#4191,#2074,.T.);
#5335=EDGE_CURVE('',#4192,#4190,#2075,.T.);
#5336=EDGE_CURVE('',#4194,#4195,#2873,.T.);
#5337=EDGE_CURVE('',#4195,#4193,#2076,.T.);
#5338=EDGE_CURVE('',#4194,#4192,#2077,.T.);
#5339=EDGE_CURVE('',#4196,#4197,#2874,.T.);
#5340=EDGE_CURVE('',#4197,#4195,#2078,.T.);
#5341=EDGE_CURVE('',#4196,#4194,#2079,.T.);
#5342=EDGE_CURVE('',#4198,#4199,#2875,.T.);
#5343=EDGE_CURVE('',#4199,#4197,#2080,.T.);
#5344=EDGE_CURVE('',#4198,#4196,#2081,.T.);
#5345=EDGE_CURVE('',#4200,#4201,#2876,.T.);
#5346=EDGE_CURVE('',#4201,#4199,#2082,.T.);
#5347=EDGE_CURVE('',#4200,#4198,#2083,.T.);
#5348=EDGE_CURVE('',#4202,#4203,#2877,.T.);
#5349=EDGE_CURVE('',#4203,#4201,#2084,.T.);
#5350=EDGE_CURVE('',#4202,#4200,#2085,.T.);
#5351=EDGE_CURVE('',#4204,#4205,#2878,.T.);
#5352=EDGE_CURVE('',#4205,#4203,#2086,.T.);
#5353=EDGE_CURVE('',#4204,#4202,#2087,.T.);
#5354=EDGE_CURVE('',#4206,#4207,#2879,.T.);
#5355=EDGE_CURVE('',#4207,#4205,#2088,.T.);
#5356=EDGE_CURVE('',#4206,#4204,#2089,.T.);
#5357=EDGE_CURVE('',#4208,#4209,#2880,.T.);
#5358=EDGE_CURVE('',#4209,#4207,#2090,.T.);
#5359=EDGE_CURVE('',#4208,#4206,#2091,.T.);
#5360=EDGE_CURVE('',#4210,#4211,#2881,.T.);
#5361=EDGE_CURVE('',#4212,#4210,#2092,.T.);
#5362=EDGE_CURVE('',#4213,#4212,#1810,.T.);
#5363=EDGE_CURVE('',#4213,#4211,#2093,.T.);
#5364=EDGE_CURVE('',#4214,#4215,#2882,.T.);
#5365=EDGE_CURVE('',#4215,#4216,#2094,.T.);
#5366=EDGE_CURVE('',#4216,#4217,#1811,.T.);
#5367=EDGE_CURVE('',#4217,#4218,#2095,.T.);
#5368=EDGE_CURVE('',#4218,#4219,#2883,.T.);
#5369=EDGE_CURVE('',#4219,#4219,#1812,.F.);
#5370=EDGE_CURVE('',#4218,#4214,#2096,.T.);
#5371=EDGE_CURVE('',#4220,#4221,#2884,.T.);
#5372=EDGE_CURVE('',#4221,#4215,#2097,.T.);
#5373=EDGE_CURVE('',#4214,#4220,#2098,.T.);
#5374=EDGE_CURVE('',#4222,#4223,#2885,.T.);
#5375=EDGE_CURVE('',#4223,#4221,#2099,.T.);
#5376=EDGE_CURVE('',#4220,#4222,#2100,.T.);
#5377=EDGE_CURVE('',#4224,#4225,#2886,.T.);
#5378=EDGE_CURVE('',#4225,#4223,#2101,.T.);
#5379=EDGE_CURVE('',#4222,#4224,#2102,.T.);
#5380=EDGE_CURVE('',#4226,#4227,#2887,.T.);
#5381=EDGE_CURVE('',#4227,#4225,#2103,.T.);
#5382=EDGE_CURVE('',#4224,#4226,#2104,.T.);
#5383=EDGE_CURVE('',#4228,#4229,#2888,.T.);
#5384=EDGE_CURVE('',#4229,#4227,#2105,.T.);
#5385=EDGE_CURVE('',#4226,#4228,#2106,.T.);
#5386=EDGE_CURVE('',#4230,#4231,#2889,.T.);
#5387=EDGE_CURVE('',#4231,#4229,#2107,.T.);
#5388=EDGE_CURVE('',#4228,#4230,#2108,.T.);
#5389=EDGE_CURVE('',#4232,#4233,#2890,.T.);
#5390=EDGE_CURVE('',#4233,#4231,#2109,.T.);
#5391=EDGE_CURVE('',#4230,#4232,#2110,.T.);
#5392=EDGE_CURVE('',#4234,#4235,#2891,.T.);
#5393=EDGE_CURVE('',#4235,#4233,#2111,.T.);
#5394=EDGE_CURVE('',#4232,#4234,#2112,.T.);
#5395=EDGE_CURVE('',#4236,#4237,#2892,.T.);
#5396=EDGE_CURVE('',#4237,#4235,#2113,.T.);
#5397=EDGE_CURVE('',#4234,#4236,#2114,.T.);
#5398=EDGE_CURVE('',#4238,#4239,#2893,.T.);
#5399=EDGE_CURVE('',#4239,#4237,#2115,.T.);
#5400=EDGE_CURVE('',#4236,#4238,#2116,.T.);
#5401=EDGE_CURVE('',#4240,#4241,#2894,.T.);
#5402=EDGE_CURVE('',#4240,#4242,#2117,.T.);
#5403=EDGE_CURVE('',#4243,#4242,#1813,.T.);
#5404=EDGE_CURVE('',#4243,#4241,#2118,.T.);
#5405=EDGE_CURVE('',#4244,#4245,#2895,.T.);
#5406=EDGE_CURVE('',#4245,#4246,#2119,.T.);
#5407=EDGE_CURVE('',#4247,#4246,#1814,.T.);
#5408=EDGE_CURVE('',#4244,#4247,#2120,.T.);
#5409=EDGE_CURVE('',#4248,#4249,#2896,.T.);
#5410=EDGE_CURVE('',#4249,#4245,#2121,.T.);
#5411=EDGE_CURVE('',#4248,#4244,#2122,.T.);
#5412=EDGE_CURVE('',#4250,#4251,#2897,.T.);
#5413=EDGE_CURVE('',#4251,#4249,#2123,.T.);
#5414=EDGE_CURVE('',#4250,#4248,#2124,.T.);
#5415=EDGE_CURVE('',#4252,#4253,#2898,.T.);
#5416=EDGE_CURVE('',#4253,#4251,#2125,.T.);
#5417=EDGE_CURVE('',#4252,#4250,#2126,.T.);
#5418=EDGE_CURVE('',#4254,#4255,#2899,.T.);
#5419=EDGE_CURVE('',#4255,#4253,#2127,.T.);
#5420=EDGE_CURVE('',#4254,#4252,#2128,.T.);
#5421=EDGE_CURVE('',#4256,#4257,#2900,.T.);
#5422=EDGE_CURVE('',#4257,#4255,#2129,.T.);
#5423=EDGE_CURVE('',#4256,#4254,#2130,.T.);
#5424=EDGE_CURVE('',#4258,#4259,#2901,.T.);
#5425=EDGE_CURVE('',#4259,#4257,#2131,.T.);
#5426=EDGE_CURVE('',#4258,#4256,#2132,.T.);
#5427=EDGE_CURVE('',#4260,#4261,#2902,.T.);
#5428=EDGE_CURVE('',#4261,#4259,#2133,.T.);
#5429=EDGE_CURVE('',#4260,#4258,#2134,.T.);
#5430=EDGE_CURVE('',#4262,#4263,#2903,.T.);
#5431=EDGE_CURVE('',#4263,#4261,#2135,.T.);
#5432=EDGE_CURVE('',#4262,#4260,#2136,.T.);
#5433=EDGE_CURVE('',#4264,#4265,#2904,.T.);
#5434=EDGE_CURVE('',#4265,#4263,#2137,.T.);
#5435=EDGE_CURVE('',#4264,#4262,#2138,.T.);
#5436=EDGE_CURVE('',#4266,#4267,#2905,.T.);
#5437=EDGE_CURVE('',#4267,#4265,#2139,.T.);
#5438=EDGE_CURVE('',#4266,#4264,#2140,.T.);
#5439=EDGE_CURVE('',#4268,#4269,#2906,.T.);
#5440=EDGE_CURVE('',#4269,#4267,#2141,.T.);
#5441=EDGE_CURVE('',#4268,#4266,#2142,.T.);
#5442=EDGE_CURVE('',#4270,#4271,#2907,.T.);
#5443=EDGE_CURVE('',#4272,#4270,#2143,.T.);
#5444=EDGE_CURVE('',#4273,#4272,#1815,.T.);
#5445=EDGE_CURVE('',#4273,#4271,#2144,.T.);
#5446=EDGE_CURVE('',#4274,#4275,#2908,.T.);
#5447=EDGE_CURVE('',#4275,#4276,#2145,.T.);
#5448=EDGE_CURVE('',#4276,#4277,#1816,.T.);
#5449=EDGE_CURVE('',#4277,#4278,#2146,.T.);
#5450=EDGE_CURVE('',#4278,#4279,#2909,.T.);
#5451=EDGE_CURVE('',#4279,#4279,#1817,.F.);
#5452=EDGE_CURVE('',#4278,#4274,#2147,.T.);
#5453=EDGE_CURVE('',#4280,#4281,#2910,.T.);
#5454=EDGE_CURVE('',#4281,#4275,#2148,.T.);
#5455=EDGE_CURVE('',#4274,#4280,#2149,.T.);
#5456=EDGE_CURVE('',#4282,#4283,#2911,.T.);
#5457=EDGE_CURVE('',#4283,#4281,#2150,.T.);
#5458=EDGE_CURVE('',#4280,#4282,#2151,.T.);
#5459=EDGE_CURVE('',#4284,#4285,#2912,.T.);
#5460=EDGE_CURVE('',#4285,#4283,#2152,.T.);
#5461=EDGE_CURVE('',#4282,#4284,#2153,.T.);
#5462=EDGE_CURVE('',#4286,#4287,#2913,.T.);
#5463=EDGE_CURVE('',#4287,#4285,#2154,.T.);
#5464=EDGE_CURVE('',#4284,#4286,#2155,.T.);
#5465=EDGE_CURVE('',#4288,#4289,#2914,.T.);
#5466=EDGE_CURVE('',#4289,#4287,#2156,.T.);
#5467=EDGE_CURVE('',#4286,#4288,#2157,.T.);
#5468=EDGE_CURVE('',#4290,#4291,#2915,.T.);
#5469=EDGE_CURVE('',#4291,#4289,#2158,.T.);
#5470=EDGE_CURVE('',#4288,#4290,#2159,.T.);
#5471=EDGE_CURVE('',#4292,#4293,#2916,.T.);
#5472=EDGE_CURVE('',#4293,#4291,#2160,.T.);
#5473=EDGE_CURVE('',#4290,#4292,#2161,.T.);
#5474=EDGE_CURVE('',#4294,#4295,#2917,.T.);
#5475=EDGE_CURVE('',#4295,#4293,#2162,.T.);
#5476=EDGE_CURVE('',#4292,#4294,#2163,.T.);
#5477=EDGE_CURVE('',#4296,#4297,#2918,.T.);
#5478=EDGE_CURVE('',#4297,#4295,#2164,.T.);
#5479=EDGE_CURVE('',#4294,#4296,#2165,.T.);
#5480=EDGE_CURVE('',#4298,#4299,#2919,.T.);
#5481=EDGE_CURVE('',#4299,#4297,#2166,.T.);
#5482=EDGE_CURVE('',#4296,#4298,#2167,.T.);
#5483=EDGE_CURVE('',#4300,#4301,#2920,.T.);
#5484=EDGE_CURVE('',#4300,#4302,#2168,.T.);
#5485=EDGE_CURVE('',#4303,#4302,#1818,.T.);
#5486=EDGE_CURVE('',#4303,#4301,#2169,.T.);
#5487=EDGE_CURVE('',#4304,#4305,#2921,.T.);
#5488=EDGE_CURVE('',#4305,#4306,#2170,.T.);
#5489=EDGE_CURVE('',#4307,#4306,#1819,.T.);
#5490=EDGE_CURVE('',#4304,#4307,#2171,.T.);
#5491=EDGE_CURVE('',#4308,#4309,#2922,.T.);
#5492=EDGE_CURVE('',#4309,#4305,#2172,.T.);
#5493=EDGE_CURVE('',#4308,#4304,#2173,.T.);
#5494=EDGE_CURVE('',#4310,#4311,#2923,.T.);
#5495=EDGE_CURVE('',#4311,#4309,#2174,.T.);
#5496=EDGE_CURVE('',#4310,#4308,#2175,.T.);
#5497=EDGE_CURVE('',#4312,#4313,#2924,.T.);
#5498=EDGE_CURVE('',#4313,#4311,#2176,.T.);
#5499=EDGE_CURVE('',#4312,#4310,#2177,.T.);
#5500=EDGE_CURVE('',#4314,#4315,#2925,.T.);
#5501=EDGE_CURVE('',#4315,#4313,#2178,.T.);
#5502=EDGE_CURVE('',#4314,#4312,#2179,.T.);
#5503=EDGE_CURVE('',#4316,#4317,#2926,.T.);
#5504=EDGE_CURVE('',#4317,#4315,#2180,.T.);
#5505=EDGE_CURVE('',#4316,#4314,#2181,.T.);
#5506=EDGE_CURVE('',#4318,#4319,#2927,.T.);
#5507=EDGE_CURVE('',#4319,#4317,#2182,.T.);
#5508=EDGE_CURVE('',#4318,#4316,#2183,.T.);
#5509=EDGE_CURVE('',#4320,#4321,#2928,.T.);
#5510=EDGE_CURVE('',#4321,#4319,#2184,.T.);
#5511=EDGE_CURVE('',#4320,#4318,#2185,.T.);
#5512=EDGE_CURVE('',#4322,#4323,#2929,.T.);
#5513=EDGE_CURVE('',#4323,#4321,#2186,.T.);
#5514=EDGE_CURVE('',#4322,#4320,#2187,.T.);
#5515=EDGE_CURVE('',#4324,#4325,#2930,.T.);
#5516=EDGE_CURVE('',#4325,#4323,#2188,.T.);
#5517=EDGE_CURVE('',#4324,#4322,#2189,.T.);
#5518=EDGE_CURVE('',#4326,#4327,#2931,.T.);
#5519=EDGE_CURVE('',#4327,#4325,#2190,.T.);
#5520=EDGE_CURVE('',#4326,#4324,#2191,.T.);
#5521=EDGE_CURVE('',#4328,#4329,#2932,.T.);
#5522=EDGE_CURVE('',#4329,#4327,#2192,.T.);
#5523=EDGE_CURVE('',#4328,#4326,#2193,.T.);
#5524=EDGE_CURVE('',#4330,#4331,#2933,.T.);
#5525=EDGE_CURVE('',#4332,#4330,#2194,.T.);
#5526=EDGE_CURVE('',#4333,#4332,#1820,.T.);
#5527=EDGE_CURVE('',#4333,#4331,#2195,.T.);
#5528=EDGE_CURVE('',#4334,#4334,#1821,.T.);
#5529=EDGE_CURVE('',#4334,#4335,#2934,.T.);
#5530=EDGE_CURVE('',#4335,#4335,#1822,.T.);
#5531=EDGE_CURVE('',#4336,#4336,#1823,.T.);
#5532=EDGE_CURVE('',#4337,#4337,#1824,.T.);
#5533=EDGE_CURVE('',#4338,#4338,#1825,.T.);
#5534=EDGE_CURVE('',#4338,#4336,#2935,.T.);
#5535=EDGE_CURVE('',#4337,#4339,#2936,.T.);
#5536=EDGE_CURVE('',#4339,#4339,#1826,.T.);
#5537=EDGE_CURVE('',#4340,#4340,#1827,.T.);
#5538=EDGE_CURVE('',#4341,#4341,#1828,.T.);
#5539=EDGE_CURVE('',#4342,#4342,#1829,.T.);
#5540=EDGE_CURVE('',#4342,#4340,#2937,.T.);
#5541=EDGE_CURVE('',#4341,#4343,#2938,.T.);
#5542=EDGE_CURVE('',#4343,#4343,#1830,.T.);
#5543=EDGE_CURVE('',#4276,#4307,#2196,.T.);
#5544=EDGE_CURVE('',#4306,#4277,#2197,.T.);
#5545=EDGE_CURVE('',#4331,#4329,#2198,.T.);
#5546=EDGE_CURVE('',#4330,#4328,#2199,.T.);
#5547=EDGE_CURVE('',#4302,#4333,#2200,.T.);
#5548=EDGE_CURVE('',#4298,#4300,#2201,.T.);
#5549=EDGE_CURVE('',#4301,#4299,#2202,.T.);
#5550=EDGE_CURVE('',#4332,#4303,#2203,.T.);
#5551=EDGE_CURVE('',#4216,#4247,#2204,.T.);
#5552=EDGE_CURVE('',#4246,#4217,#2205,.T.);
#5553=EDGE_CURVE('',#4271,#4269,#2206,.T.);
#5554=EDGE_CURVE('',#4270,#4268,#2207,.T.);
#5555=EDGE_CURVE('',#4242,#4273,#2208,.T.);
#5556=EDGE_CURVE('',#4238,#4240,#2209,.T.);
#5557=EDGE_CURVE('',#4241,#4239,#2210,.T.);
#5558=EDGE_CURVE('',#4272,#4243,#2211,.T.);
#5559=EDGE_CURVE('',#4156,#4187,#2212,.T.);
#5560=EDGE_CURVE('',#4186,#4157,#2213,.T.);
#5561=EDGE_CURVE('',#4211,#4209,#2214,.T.);
#5562=EDGE_CURVE('',#4210,#4208,#2215,.T.);
#5563=EDGE_CURVE('',#4182,#4213,#2216,.T.);
#5564=EDGE_CURVE('',#4178,#4180,#2217,.T.);
#5565=EDGE_CURVE('',#4181,#4179,#2218,.T.);
#5566=EDGE_CURVE('',#4212,#4183,#2219,.T.);
#5567=EDGE_CURVE('',#4096,#4127,#2220,.T.);
#5568=EDGE_CURVE('',#4126,#4097,#2221,.T.);
#5569=EDGE_CURVE('',#4151,#4149,#2222,.T.);
#5570=EDGE_CURVE('',#4150,#4148,#2223,.T.);
#5571=EDGE_CURVE('',#4122,#4153,#2224,.T.);
#5572=EDGE_CURVE('',#4118,#4120,#2225,.T.);
#5573=EDGE_CURVE('',#4121,#4119,#2226,.T.);
#5574=EDGE_CURVE('',#4152,#4123,#2227,.T.);
#5575=EDGE_CURVE('',#4344,#4344,#1831,.T.);
#5576=EDGE_CURVE('',#4344,#4345,#2939,.T.);
#5577=EDGE_CURVE('',#4345,#4345,#1832,.T.);
#5578=EDGE_CURVE('',#4346,#4346,#1833,.T.);
#5579=EDGE_CURVE('',#4346,#4347,#2940,.T.);
#5580=EDGE_CURVE('',#4347,#4347,#1834,.T.);
#5581=EDGE_CURVE('',#4348,#4349,#2941,.T.);
#5582=EDGE_CURVE('',#4350,#4349,#2942,.T.);
#5583=EDGE_CURVE('',#4351,#4350,#2943,.T.);
#5584=EDGE_CURVE('',#4348,#4351,#2944,.T.);
#5585=EDGE_CURVE('',#4352,#4348,#2945,.T.);
#5586=EDGE_CURVE('',#4353,#4351,#2946,.T.);
#5587=EDGE_CURVE('',#4352,#4353,#2947,.T.);
#5588=EDGE_CURVE('',#4354,#4352,#2948,.T.);
#5589=EDGE_CURVE('',#4355,#4353,#2949,.T.);
#5590=EDGE_CURVE('',#4354,#4355,#2950,.T.);
#5591=EDGE_CURVE('',#4355,#4350,#2951,.T.);
#5592=EDGE_CURVE('',#4356,#4357,#2952,.T.);
#5593=EDGE_CURVE('',#4357,#4358,#2953,.T.);
#5594=EDGE_CURVE('',#4359,#4358,#2954,.T.);
#5595=EDGE_CURVE('',#4356,#4359,#2955,.T.);
#5596=EDGE_CURVE('',#4360,#4361,#2956,.T.);
#5597=EDGE_CURVE('',#4362,#4361,#2957,.T.);
#5598=EDGE_CURVE('',#4363,#4362,#2958,.T.);
#5599=EDGE_CURVE('',#4360,#4363,#2959,.T.);
#5600=EDGE_CURVE('',#4357,#4360,#2960,.T.);
#5601=EDGE_CURVE('',#4358,#4363,#2961,.T.);
#5602=EDGE_CURVE('',#4359,#4362,#2962,.T.);
#5603=EDGE_CURVE('',#4364,#4364,#1835,.T.);
#5604=EDGE_CURVE('',#4364,#4365,#2963,.T.);
#5605=EDGE_CURVE('',#4365,#4365,#1836,.T.);
#5606=EDGE_CURVE('',#4366,#4366,#1837,.T.);
#5607=EDGE_CURVE('',#4366,#4367,#2964,.T.);
#5608=EDGE_CURVE('',#4367,#4367,#1838,.T.);
#5609=EDGE_CURVE('',#4368,#4369,#1839,.T.);
#5610=EDGE_CURVE('',#4370,#4369,#2965,.T.);
#5611=EDGE_CURVE('',#4370,#4371,#1840,.T.);
#5612=EDGE_CURVE('',#4372,#4371,#2966,.T.);
#5613=EDGE_CURVE('',#4372,#4373,#1841,.T.);
#5614=EDGE_CURVE('',#4374,#4373,#2967,.T.);
#5615=EDGE_CURVE('',#4374,#4375,#1842,.T.);
#5616=EDGE_CURVE('',#4368,#4375,#2968,.T.);
#5617=EDGE_CURVE('',#4368,#4376,#2969,.T.);
#5618=EDGE_CURVE('',#4376,#4377,#1843,.T.);
#5619=EDGE_CURVE('',#4377,#4369,#2970,.T.);
#5620=EDGE_CURVE('',#4378,#4375,#2971,.T.);
#5621=EDGE_CURVE('',#4376,#4378,#2972,.T.);
#5622=EDGE_CURVE('',#4374,#4379,#2973,.T.);
#5623=EDGE_CURVE('',#4379,#4378,#1844,.T.);
#5624=EDGE_CURVE('',#4380,#4373,#2974,.T.);
#5625=EDGE_CURVE('',#4379,#4380,#2975,.T.);
#5626=EDGE_CURVE('',#4370,#4381,#2976,.T.);
#5627=EDGE_CURVE('',#4381,#4382,#1845,.T.);
#5628=EDGE_CURVE('',#4382,#4371,#2977,.T.);
#5629=EDGE_CURVE('',#4383,#4382,#2978,.T.);
#5630=EDGE_CURVE('',#4372,#4383,#2979,.T.);
#5631=EDGE_CURVE('',#4383,#4380,#1846,.T.);
#5632=EDGE_CURVE('',#4381,#4377,#2980,.T.);
#5633=EDGE_CURVE('',#4384,#4385,#2981,.T.);
#5634=EDGE_CURVE('',#4385,#4386,#2982,.T.);
#5635=EDGE_CURVE('',#4387,#4386,#2983,.T.);
#5636=EDGE_CURVE('',#4384,#4387,#2984,.T.);
#5637=EDGE_CURVE('',#4349,#4384,#2985,.T.);
#5638=EDGE_CURVE('',#4388,#4387,#2986,.T.);
#5639=EDGE_CURVE('',#4389,#4388,#2987,.T.);
#5640=EDGE_CURVE('',#4389,#4354,#2988,.T.);
#5641=EDGE_CURVE('',#4390,#4389,#2989,.T.);
#5642=EDGE_CURVE('',#4391,#4388,#2990,.T.);
#5643=EDGE_CURVE('',#4390,#4391,#2991,.T.);
#5644=EDGE_CURVE('',#4361,#4390,#2992,.T.);
#5645=EDGE_CURVE('',#4386,#4391,#2993,.T.);
#5646=EDGE_CURVE('',#4385,#4356,#2994,.T.);
#6861=ORIENTED_EDGE('',*,*,#5200,.T.);
#6862=ORIENTED_EDGE('',*,*,#5201,.T.);
#6863=ORIENTED_EDGE('',*,*,#5202,.T.);
#6864=ORIENTED_EDGE('',*,*,#5203,.T.);
#6865=ORIENTED_EDGE('',*,*,#5204,.T.);
#6866=ORIENTED_EDGE('',*,*,#5205,.T.);
#6867=ORIENTED_EDGE('',*,*,#5204,.F.);
#6868=ORIENTED_EDGE('',*,*,#5206,.T.);
#6869=ORIENTED_EDGE('',*,*,#5207,.T.);
#6870=ORIENTED_EDGE('',*,*,#5208,.T.);
#6871=ORIENTED_EDGE('',*,*,#5200,.F.);
#6872=ORIENTED_EDGE('',*,*,#5209,.T.);
#6873=ORIENTED_EDGE('',*,*,#5210,.T.);
#6874=ORIENTED_EDGE('',*,*,#5211,.T.);
#6875=ORIENTED_EDGE('',*,*,#5207,.F.);
#6876=ORIENTED_EDGE('',*,*,#5212,.T.);
#6877=ORIENTED_EDGE('',*,*,#5213,.T.);
#6878=ORIENTED_EDGE('',*,*,#5214,.T.);
#6879=ORIENTED_EDGE('',*,*,#5210,.F.);
#6880=ORIENTED_EDGE('',*,*,#5215,.T.);
#6881=ORIENTED_EDGE('',*,*,#5216,.T.);
#6882=ORIENTED_EDGE('',*,*,#5217,.T.);
#6883=ORIENTED_EDGE('',*,*,#5213,.F.);
#6884=ORIENTED_EDGE('',*,*,#5218,.T.);
#6885=ORIENTED_EDGE('',*,*,#5219,.T.);
#6886=ORIENTED_EDGE('',*,*,#5220,.T.);
#6887=ORIENTED_EDGE('',*,*,#5216,.F.);
#6888=ORIENTED_EDGE('',*,*,#5221,.T.);
#6889=ORIENTED_EDGE('',*,*,#5222,.T.);
#6890=ORIENTED_EDGE('',*,*,#5223,.T.);
#6891=ORIENTED_EDGE('',*,*,#5219,.F.);
#6892=ORIENTED_EDGE('',*,*,#5224,.T.);
#6893=ORIENTED_EDGE('',*,*,#5225,.T.);
#6894=ORIENTED_EDGE('',*,*,#5226,.T.);
#6895=ORIENTED_EDGE('',*,*,#5222,.F.);
#6896=ORIENTED_EDGE('',*,*,#5227,.T.);
#6897=ORIENTED_EDGE('',*,*,#5228,.T.);
#6898=ORIENTED_EDGE('',*,*,#5229,.T.);
#6899=ORIENTED_EDGE('',*,*,#5225,.F.);
#6900=ORIENTED_EDGE('',*,*,#5230,.T.);
#6901=ORIENTED_EDGE('',*,*,#5231,.T.);
#6902=ORIENTED_EDGE('',*,*,#5232,.T.);
#6903=ORIENTED_EDGE('',*,*,#5228,.F.);
#6904=ORIENTED_EDGE('',*,*,#5233,.T.);
#6905=ORIENTED_EDGE('',*,*,#5234,.T.);
#6906=ORIENTED_EDGE('',*,*,#5235,.T.);
#6907=ORIENTED_EDGE('',*,*,#5231,.F.);
#6908=ORIENTED_EDGE('',*,*,#5236,.T.);
#6909=ORIENTED_EDGE('',*,*,#5237,.F.);
#6910=ORIENTED_EDGE('',*,*,#5238,.T.);
#6911=ORIENTED_EDGE('',*,*,#5239,.F.);
#6912=ORIENTED_EDGE('',*,*,#5240,.T.);
#6913=ORIENTED_EDGE('',*,*,#5241,.T.);
#6914=ORIENTED_EDGE('',*,*,#5242,.T.);
#6915=ORIENTED_EDGE('',*,*,#5243,.F.);
#6916=ORIENTED_EDGE('',*,*,#5244,.F.);
#6917=ORIENTED_EDGE('',*,*,#5245,.T.);
#6918=ORIENTED_EDGE('',*,*,#5246,.T.);
#6919=ORIENTED_EDGE('',*,*,#5241,.F.);
#6920=ORIENTED_EDGE('',*,*,#5247,.F.);
#6921=ORIENTED_EDGE('',*,*,#5248,.T.);
#6922=ORIENTED_EDGE('',*,*,#5249,.T.);
#6923=ORIENTED_EDGE('',*,*,#5245,.F.);
#6924=ORIENTED_EDGE('',*,*,#5250,.F.);
#6925=ORIENTED_EDGE('',*,*,#5251,.T.);
#6926=ORIENTED_EDGE('',*,*,#5252,.T.);
#6927=ORIENTED_EDGE('',*,*,#5248,.F.);
#6928=ORIENTED_EDGE('',*,*,#5253,.F.);
#6929=ORIENTED_EDGE('',*,*,#5254,.T.);
#6930=ORIENTED_EDGE('',*,*,#5255,.T.);
#6931=ORIENTED_EDGE('',*,*,#5251,.F.);
#6932=ORIENTED_EDGE('',*,*,#5256,.F.);
#6933=ORIENTED_EDGE('',*,*,#5257,.T.);
#6934=ORIENTED_EDGE('',*,*,#5258,.T.);
#6935=ORIENTED_EDGE('',*,*,#5254,.F.);
#6936=ORIENTED_EDGE('',*,*,#5259,.F.);
#6937=ORIENTED_EDGE('',*,*,#5260,.T.);
#6938=ORIENTED_EDGE('',*,*,#5261,.T.);
#6939=ORIENTED_EDGE('',*,*,#5257,.F.);
#6940=ORIENTED_EDGE('',*,*,#5262,.F.);
#6941=ORIENTED_EDGE('',*,*,#5263,.T.);
#6942=ORIENTED_EDGE('',*,*,#5264,.T.);
#6943=ORIENTED_EDGE('',*,*,#5260,.F.);
#6944=ORIENTED_EDGE('',*,*,#5265,.F.);
#6945=ORIENTED_EDGE('',*,*,#5266,.T.);
#6946=ORIENTED_EDGE('',*,*,#5267,.T.);
#6947=ORIENTED_EDGE('',*,*,#5263,.F.);
#6948=ORIENTED_EDGE('',*,*,#5268,.F.);
#6949=ORIENTED_EDGE('',*,*,#5269,.T.);
#6950=ORIENTED_EDGE('',*,*,#5270,.T.);
#6951=ORIENTED_EDGE('',*,*,#5266,.F.);
#6952=ORIENTED_EDGE('',*,*,#5271,.F.);
#6953=ORIENTED_EDGE('',*,*,#5272,.T.);
#6954=ORIENTED_EDGE('',*,*,#5273,.T.);
#6955=ORIENTED_EDGE('',*,*,#5269,.F.);
#6956=ORIENTED_EDGE('',*,*,#5274,.F.);
#6957=ORIENTED_EDGE('',*,*,#5275,.T.);
#6958=ORIENTED_EDGE('',*,*,#5276,.T.);
#6959=ORIENTED_EDGE('',*,*,#5272,.F.);
#6960=ORIENTED_EDGE('',*,*,#5277,.F.);
#6961=ORIENTED_EDGE('',*,*,#5278,.F.);
#6962=ORIENTED_EDGE('',*,*,#5279,.F.);
#6963=ORIENTED_EDGE('',*,*,#5280,.F.);
#6964=ORIENTED_EDGE('',*,*,#5281,.T.);
#6965=ORIENTED_EDGE('',*,*,#5282,.T.);
#6966=ORIENTED_EDGE('',*,*,#5283,.T.);
#6967=ORIENTED_EDGE('',*,*,#5284,.T.);
#6968=ORIENTED_EDGE('',*,*,#5285,.T.);
#6969=ORIENTED_EDGE('',*,*,#5286,.T.);
#6970=ORIENTED_EDGE('',*,*,#5287,.T.);
#6971=ORIENTED_EDGE('',*,*,#5286,.F.);
#6972=ORIENTED_EDGE('',*,*,#5288,.T.);
#6973=ORIENTED_EDGE('',*,*,#5289,.T.);
#6974=ORIENTED_EDGE('',*,*,#5290,.T.);
#6975=ORIENTED_EDGE('',*,*,#5282,.F.);
#6976=ORIENTED_EDGE('',*,*,#5291,.T.);
#6977=ORIENTED_EDGE('',*,*,#5292,.T.);
#6978=ORIENTED_EDGE('',*,*,#5293,.T.);
#6979=ORIENTED_EDGE('',*,*,#5289,.F.);
#6980=ORIENTED_EDGE('',*,*,#5294,.T.);
#6981=ORIENTED_EDGE('',*,*,#5295,.T.);
#6982=ORIENTED_EDGE('',*,*,#5296,.T.);
#6983=ORIENTED_EDGE('',*,*,#5292,.F.);
#6984=ORIENTED_EDGE('',*,*,#5297,.T.);
#6985=ORIENTED_EDGE('',*,*,#5298,.T.);
#6986=ORIENTED_EDGE('',*,*,#5299,.T.);
#6987=ORIENTED_EDGE('',*,*,#5295,.F.);
#6988=ORIENTED_EDGE('',*,*,#5300,.T.);
#6989=ORIENTED_EDGE('',*,*,#5301,.T.);
#6990=ORIENTED_EDGE('',*,*,#5302,.T.);
#6991=ORIENTED_EDGE('',*,*,#5298,.F.);
#6992=ORIENTED_EDGE('',*,*,#5303,.T.);
#6993=ORIENTED_EDGE('',*,*,#5304,.T.);
#6994=ORIENTED_EDGE('',*,*,#5305,.T.);
#6995=ORIENTED_EDGE('',*,*,#5301,.F.);
#6996=ORIENTED_EDGE('',*,*,#5306,.T.);
#6997=ORIENTED_EDGE('',*,*,#5307,.T.);
#6998=ORIENTED_EDGE('',*,*,#5308,.T.);
#6999=ORIENTED_EDGE('',*,*,#5304,.F.);
#7000=ORIENTED_EDGE('',*,*,#5309,.T.);
#7001=ORIENTED_EDGE('',*,*,#5310,.T.);
#7002=ORIENTED_EDGE('',*,*,#5311,.T.);
#7003=ORIENTED_EDGE('',*,*,#5307,.F.);
#7004=ORIENTED_EDGE('',*,*,#5312,.T.);
#7005=ORIENTED_EDGE('',*,*,#5313,.T.);
#7006=ORIENTED_EDGE('',*,*,#5314,.T.);
#7007=ORIENTED_EDGE('',*,*,#5310,.F.);
#7008=ORIENTED_EDGE('',*,*,#5315,.T.);
#7009=ORIENTED_EDGE('',*,*,#5316,.T.);
#7010=ORIENTED_EDGE('',*,*,#5317,.T.);
#7011=ORIENTED_EDGE('',*,*,#5313,.F.);
#7012=ORIENTED_EDGE('',*,*,#5318,.T.);
#7013=ORIENTED_EDGE('',*,*,#5319,.F.);
#7014=ORIENTED_EDGE('',*,*,#5320,.T.);
#7015=ORIENTED_EDGE('',*,*,#5321,.F.);
#7016=ORIENTED_EDGE('',*,*,#5322,.T.);
#7017=ORIENTED_EDGE('',*,*,#5323,.T.);
#7018=ORIENTED_EDGE('',*,*,#5324,.T.);
#7019=ORIENTED_EDGE('',*,*,#5325,.F.);
#7020=ORIENTED_EDGE('',*,*,#5326,.F.);
#7021=ORIENTED_EDGE('',*,*,#5327,.T.);
#7022=ORIENTED_EDGE('',*,*,#5328,.T.);
#7023=ORIENTED_EDGE('',*,*,#5323,.F.);
#7024=ORIENTED_EDGE('',*,*,#5329,.F.);
#7025=ORIENTED_EDGE('',*,*,#5330,.T.);
#7026=ORIENTED_EDGE('',*,*,#5331,.T.);
#7027=ORIENTED_EDGE('',*,*,#5327,.F.);
#7028=ORIENTED_EDGE('',*,*,#5332,.F.);
#7029=ORIENTED_EDGE('',*,*,#5333,.T.);
#7030=ORIENTED_EDGE('',*,*,#5334,.T.);
#7031=ORIENTED_EDGE('',*,*,#5330,.F.);
#7032=ORIENTED_EDGE('',*,*,#5335,.F.);
#7033=ORIENTED_EDGE('',*,*,#5336,.T.);
#7034=ORIENTED_EDGE('',*,*,#5337,.T.);
#7035=ORIENTED_EDGE('',*,*,#5333,.F.);
#7036=ORIENTED_EDGE('',*,*,#5338,.F.);
#7037=ORIENTED_EDGE('',*,*,#5339,.T.);
#7038=ORIENTED_EDGE('',*,*,#5340,.T.);
#7039=ORIENTED_EDGE('',*,*,#5336,.F.);
#7040=ORIENTED_EDGE('',*,*,#5341,.F.);
#7041=ORIENTED_EDGE('',*,*,#5342,.T.);
#7042=ORIENTED_EDGE('',*,*,#5343,.T.);
#7043=ORIENTED_EDGE('',*,*,#5339,.F.);
#7044=ORIENTED_EDGE('',*,*,#5344,.F.);
#7045=ORIENTED_EDGE('',*,*,#5345,.T.);
#7046=ORIENTED_EDGE('',*,*,#5346,.T.);
#7047=ORIENTED_EDGE('',*,*,#5342,.F.);
#7048=ORIENTED_EDGE('',*,*,#5347,.F.);
#7049=ORIENTED_EDGE('',*,*,#5348,.T.);
#7050=ORIENTED_EDGE('',*,*,#5349,.T.);
#7051=ORIENTED_EDGE('',*,*,#5345,.F.);
#7052=ORIENTED_EDGE('',*,*,#5350,.F.);
#7053=ORIENTED_EDGE('',*,*,#5351,.T.);
#7054=ORIENTED_EDGE('',*,*,#5352,.T.);
#7055=ORIENTED_EDGE('',*,*,#5348,.F.);
#7056=ORIENTED_EDGE('',*,*,#5353,.F.);
#7057=ORIENTED_EDGE('',*,*,#5354,.T.);
#7058=ORIENTED_EDGE('',*,*,#5355,.T.);
#7059=ORIENTED_EDGE('',*,*,#5351,.F.);
#7060=ORIENTED_EDGE('',*,*,#5356,.F.);
#7061=ORIENTED_EDGE('',*,*,#5357,.T.);
#7062=ORIENTED_EDGE('',*,*,#5358,.T.);
#7063=ORIENTED_EDGE('',*,*,#5354,.F.);
#7064=ORIENTED_EDGE('',*,*,#5359,.F.);
#7065=ORIENTED_EDGE('',*,*,#5360,.F.);
#7066=ORIENTED_EDGE('',*,*,#5361,.F.);
#7067=ORIENTED_EDGE('',*,*,#5362,.F.);
#7068=ORIENTED_EDGE('',*,*,#5363,.T.);
#7069=ORIENTED_EDGE('',*,*,#5364,.T.);
#7070=ORIENTED_EDGE('',*,*,#5365,.T.);
#7071=ORIENTED_EDGE('',*,*,#5366,.T.);
#7072=ORIENTED_EDGE('',*,*,#5367,.T.);
#7073=ORIENTED_EDGE('',*,*,#5368,.T.);
#7074=ORIENTED_EDGE('',*,*,#5369,.T.);
#7075=ORIENTED_EDGE('',*,*,#5368,.F.);
#7076=ORIENTED_EDGE('',*,*,#5370,.T.);
#7077=ORIENTED_EDGE('',*,*,#5371,.T.);
#7078=ORIENTED_EDGE('',*,*,#5372,.T.);
#7079=ORIENTED_EDGE('',*,*,#5364,.F.);
#7080=ORIENTED_EDGE('',*,*,#5373,.T.);
#7081=ORIENTED_EDGE('',*,*,#5374,.T.);
#7082=ORIENTED_EDGE('',*,*,#5375,.T.);
#7083=ORIENTED_EDGE('',*,*,#5371,.F.);
#7084=ORIENTED_EDGE('',*,*,#5376,.T.);
#7085=ORIENTED_EDGE('',*,*,#5377,.T.);
#7086=ORIENTED_EDGE('',*,*,#5378,.T.);
#7087=ORIENTED_EDGE('',*,*,#5374,.F.);
#7088=ORIENTED_EDGE('',*,*,#5379,.T.);
#7089=ORIENTED_EDGE('',*,*,#5380,.T.);
#7090=ORIENTED_EDGE('',*,*,#5381,.T.);
#7091=ORIENTED_EDGE('',*,*,#5377,.F.);
#7092=ORIENTED_EDGE('',*,*,#5382,.T.);
#7093=ORIENTED_EDGE('',*,*,#5383,.T.);
#7094=ORIENTED_EDGE('',*,*,#5384,.T.);
#7095=ORIENTED_EDGE('',*,*,#5380,.F.);
#7096=ORIENTED_EDGE('',*,*,#5385,.T.);
#7097=ORIENTED_EDGE('',*,*,#5386,.T.);
#7098=ORIENTED_EDGE('',*,*,#5387,.T.);
#7099=ORIENTED_EDGE('',*,*,#5383,.F.);
#7100=ORIENTED_EDGE('',*,*,#5388,.T.);
#7101=ORIENTED_EDGE('',*,*,#5389,.T.);
#7102=ORIENTED_EDGE('',*,*,#5390,.T.);
#7103=ORIENTED_EDGE('',*,*,#5386,.F.);
#7104=ORIENTED_EDGE('',*,*,#5391,.T.);
#7105=ORIENTED_EDGE('',*,*,#5392,.T.);
#7106=ORIENTED_EDGE('',*,*,#5393,.T.);
#7107=ORIENTED_EDGE('',*,*,#5389,.F.);
#7108=ORIENTED_EDGE('',*,*,#5394,.T.);
#7109=ORIENTED_EDGE('',*,*,#5395,.T.);
#7110=ORIENTED_EDGE('',*,*,#5396,.T.);
#7111=ORIENTED_EDGE('',*,*,#5392,.F.);
#7112=ORIENTED_EDGE('',*,*,#5397,.T.);
#7113=ORIENTED_EDGE('',*,*,#5398,.T.);
#7114=ORIENTED_EDGE('',*,*,#5399,.T.);
#7115=ORIENTED_EDGE('',*,*,#5395,.F.);
#7116=ORIENTED_EDGE('',*,*,#5400,.T.);
#7117=ORIENTED_EDGE('',*,*,#5401,.F.);
#7118=ORIENTED_EDGE('',*,*,#5402,.T.);
#7119=ORIENTED_EDGE('',*,*,#5403,.F.);
#7120=ORIENTED_EDGE('',*,*,#5404,.T.);
#7121=ORIENTED_EDGE('',*,*,#5405,.T.);
#7122=ORIENTED_EDGE('',*,*,#5406,.T.);
#7123=ORIENTED_EDGE('',*,*,#5407,.F.);
#7124=ORIENTED_EDGE('',*,*,#5408,.F.);
#7125=ORIENTED_EDGE('',*,*,#5409,.T.);
#7126=ORIENTED_EDGE('',*,*,#5410,.T.);
#7127=ORIENTED_EDGE('',*,*,#5405,.F.);
#7128=ORIENTED_EDGE('',*,*,#5411,.F.);
#7129=ORIENTED_EDGE('',*,*,#5412,.T.);
#7130=ORIENTED_EDGE('',*,*,#5413,.T.);
#7131=ORIENTED_EDGE('',*,*,#5409,.F.);
#7132=ORIENTED_EDGE('',*,*,#5414,.F.);
#7133=ORIENTED_EDGE('',*,*,#5415,.T.);
#7134=ORIENTED_EDGE('',*,*,#5416,.T.);
#7135=ORIENTED_EDGE('',*,*,#5412,.F.);
#7136=ORIENTED_EDGE('',*,*,#5417,.F.);
#7137=ORIENTED_EDGE('',*,*,#5418,.T.);
#7138=ORIENTED_EDGE('',*,*,#5419,.T.);
#7139=ORIENTED_EDGE('',*,*,#5415,.F.);
#7140=ORIENTED_EDGE('',*,*,#5420,.F.);
#7141=ORIENTED_EDGE('',*,*,#5421,.T.);
#7142=ORIENTED_EDGE('',*,*,#5422,.T.);
#7143=ORIENTED_EDGE('',*,*,#5418,.F.);
#7144=ORIENTED_EDGE('',*,*,#5423,.F.);
#7145=ORIENTED_EDGE('',*,*,#5424,.T.);
#7146=ORIENTED_EDGE('',*,*,#5425,.T.);
#7147=ORIENTED_EDGE('',*,*,#5421,.F.);
#7148=ORIENTED_EDGE('',*,*,#5426,.F.);
#7149=ORIENTED_EDGE('',*,*,#5427,.T.);
#7150=ORIENTED_EDGE('',*,*,#5428,.T.);
#7151=ORIENTED_EDGE('',*,*,#5424,.F.);
#7152=ORIENTED_EDGE('',*,*,#5429,.F.);
#7153=ORIENTED_EDGE('',*,*,#5430,.T.);
#7154=ORIENTED_EDGE('',*,*,#5431,.T.);
#7155=ORIENTED_EDGE('',*,*,#5427,.F.);
#7156=ORIENTED_EDGE('',*,*,#5432,.F.);
#7157=ORIENTED_EDGE('',*,*,#5433,.T.);
#7158=ORIENTED_EDGE('',*,*,#5434,.T.);
#7159=ORIENTED_EDGE('',*,*,#5430,.F.);
#7160=ORIENTED_EDGE('',*,*,#5435,.F.);
#7161=ORIENTED_EDGE('',*,*,#5436,.T.);
#7162=ORIENTED_EDGE('',*,*,#5437,.T.);
#7163=ORIENTED_EDGE('',*,*,#5433,.F.);
#7164=ORIENTED_EDGE('',*,*,#5438,.F.);
#7165=ORIENTED_EDGE('',*,*,#5439,.T.);
#7166=ORIENTED_EDGE('',*,*,#5440,.T.);
#7167=ORIENTED_EDGE('',*,*,#5436,.F.);
#7168=ORIENTED_EDGE('',*,*,#5441,.F.);
#7169=ORIENTED_EDGE('',*,*,#5442,.F.);
#7170=ORIENTED_EDGE('',*,*,#5443,.F.);
#7171=ORIENTED_EDGE('',*,*,#5444,.F.);
#7172=ORIENTED_EDGE('',*,*,#5445,.T.);
#7173=ORIENTED_EDGE('',*,*,#5446,.T.);
#7174=ORIENTED_EDGE('',*,*,#5447,.T.);
#7175=ORIENTED_EDGE('',*,*,#5448,.T.);
#7176=ORIENTED_EDGE('',*,*,#5449,.T.);
#7177=ORIENTED_EDGE('',*,*,#5450,.T.);
#7178=ORIENTED_EDGE('',*,*,#5451,.T.);
#7179=ORIENTED_EDGE('',*,*,#5450,.F.);
#7180=ORIENTED_EDGE('',*,*,#5452,.T.);
#7181=ORIENTED_EDGE('',*,*,#5453,.T.);
#7182=ORIENTED_EDGE('',*,*,#5454,.T.);
#7183=ORIENTED_EDGE('',*,*,#5446,.F.);
#7184=ORIENTED_EDGE('',*,*,#5455,.T.);
#7185=ORIENTED_EDGE('',*,*,#5456,.T.);
#7186=ORIENTED_EDGE('',*,*,#5457,.T.);
#7187=ORIENTED_EDGE('',*,*,#5453,.F.);
#7188=ORIENTED_EDGE('',*,*,#5458,.T.);
#7189=ORIENTED_EDGE('',*,*,#5459,.T.);
#7190=ORIENTED_EDGE('',*,*,#5460,.T.);
#7191=ORIENTED_EDGE('',*,*,#5456,.F.);
#7192=ORIENTED_EDGE('',*,*,#5461,.T.);
#7193=ORIENTED_EDGE('',*,*,#5462,.T.);
#7194=ORIENTED_EDGE('',*,*,#5463,.T.);
#7195=ORIENTED_EDGE('',*,*,#5459,.F.);
#7196=ORIENTED_EDGE('',*,*,#5464,.T.);
#7197=ORIENTED_EDGE('',*,*,#5465,.T.);
#7198=ORIENTED_EDGE('',*,*,#5466,.T.);
#7199=ORIENTED_EDGE('',*,*,#5462,.F.);
#7200=ORIENTED_EDGE('',*,*,#5467,.T.);
#7201=ORIENTED_EDGE('',*,*,#5468,.T.);
#7202=ORIENTED_EDGE('',*,*,#5469,.T.);
#7203=ORIENTED_EDGE('',*,*,#5465,.F.);
#7204=ORIENTED_EDGE('',*,*,#5470,.T.);
#7205=ORIENTED_EDGE('',*,*,#5471,.T.);
#7206=ORIENTED_EDGE('',*,*,#5472,.T.);
#7207=ORIENTED_EDGE('',*,*,#5468,.F.);
#7208=ORIENTED_EDGE('',*,*,#5473,.T.);
#7209=ORIENTED_EDGE('',*,*,#5474,.T.);
#7210=ORIENTED_EDGE('',*,*,#5475,.T.);
#7211=ORIENTED_EDGE('',*,*,#5471,.F.);
#7212=ORIENTED_EDGE('',*,*,#5476,.T.);
#7213=ORIENTED_EDGE('',*,*,#5477,.T.);
#7214=ORIENTED_EDGE('',*,*,#5478,.T.);
#7215=ORIENTED_EDGE('',*,*,#5474,.F.);
#7216=ORIENTED_EDGE('',*,*,#5479,.T.);
#7217=ORIENTED_EDGE('',*,*,#5480,.T.);
#7218=ORIENTED_EDGE('',*,*,#5481,.T.);
#7219=ORIENTED_EDGE('',*,*,#5477,.F.);
#7220=ORIENTED_EDGE('',*,*,#5482,.T.);
#7221=ORIENTED_EDGE('',*,*,#5483,.F.);
#7222=ORIENTED_EDGE('',*,*,#5484,.T.);
#7223=ORIENTED_EDGE('',*,*,#5485,.F.);
#7224=ORIENTED_EDGE('',*,*,#5486,.T.);
#7225=ORIENTED_EDGE('',*,*,#5487,.T.);
#7226=ORIENTED_EDGE('',*,*,#5488,.T.);
#7227=ORIENTED_EDGE('',*,*,#5489,.F.);
#7228=ORIENTED_EDGE('',*,*,#5490,.F.);
#7229=ORIENTED_EDGE('',*,*,#5491,.T.);
#7230=ORIENTED_EDGE('',*,*,#5492,.T.);
#7231=ORIENTED_EDGE('',*,*,#5487,.F.);
#7232=ORIENTED_EDGE('',*,*,#5493,.F.);
#7233=ORIENTED_EDGE('',*,*,#5494,.T.);
#7234=ORIENTED_EDGE('',*,*,#5495,.T.);
#7235=ORIENTED_EDGE('',*,*,#5491,.F.);
#7236=ORIENTED_EDGE('',*,*,#5496,.F.);
#7237=ORIENTED_EDGE('',*,*,#5497,.T.);
#7238=ORIENTED_EDGE('',*,*,#5498,.T.);
#7239=ORIENTED_EDGE('',*,*,#5494,.F.);
#7240=ORIENTED_EDGE('',*,*,#5499,.F.);
#7241=ORIENTED_EDGE('',*,*,#5500,.T.);
#7242=ORIENTED_EDGE('',*,*,#5501,.T.);
#7243=ORIENTED_EDGE('',*,*,#5497,.F.);
#7244=ORIENTED_EDGE('',*,*,#5502,.F.);
#7245=ORIENTED_EDGE('',*,*,#5503,.T.);
#7246=ORIENTED_EDGE('',*,*,#5504,.T.);
#7247=ORIENTED_EDGE('',*,*,#5500,.F.);
#7248=ORIENTED_EDGE('',*,*,#5505,.F.);
#7249=ORIENTED_EDGE('',*,*,#5506,.T.);
#7250=ORIENTED_EDGE('',*,*,#5507,.T.);
#7251=ORIENTED_EDGE('',*,*,#5503,.F.);
#7252=ORIENTED_EDGE('',*,*,#5508,.F.);
#7253=ORIENTED_EDGE('',*,*,#5509,.T.);
#7254=ORIENTED_EDGE('',*,*,#5510,.T.);
#7255=ORIENTED_EDGE('',*,*,#5506,.F.);
#7256=ORIENTED_EDGE('',*,*,#5511,.F.);
#7257=ORIENTED_EDGE('',*,*,#5512,.T.);
#7258=ORIENTED_EDGE('',*,*,#5513,.T.);
#7259=ORIENTED_EDGE('',*,*,#5509,.F.);
#7260=ORIENTED_EDGE('',*,*,#5514,.F.);
#7261=ORIENTED_EDGE('',*,*,#5515,.T.);
#7262=ORIENTED_EDGE('',*,*,#5516,.T.);
#7263=ORIENTED_EDGE('',*,*,#5512,.F.);
#7264=ORIENTED_EDGE('',*,*,#5517,.F.);
#7265=ORIENTED_EDGE('',*,*,#5518,.T.);
#7266=ORIENTED_EDGE('',*,*,#5519,.T.);
#7267=ORIENTED_EDGE('',*,*,#5515,.F.);
#7268=ORIENTED_EDGE('',*,*,#5520,.F.);
#7269=ORIENTED_EDGE('',*,*,#5521,.T.);
#7270=ORIENTED_EDGE('',*,*,#5522,.T.);
#7271=ORIENTED_EDGE('',*,*,#5518,.F.);
#7272=ORIENTED_EDGE('',*,*,#5523,.F.);
#7273=ORIENTED_EDGE('',*,*,#5524,.F.);
#7274=ORIENTED_EDGE('',*,*,#5525,.F.);
#7275=ORIENTED_EDGE('',*,*,#5526,.F.);
#7276=ORIENTED_EDGE('',*,*,#5527,.T.);
#7277=ORIENTED_EDGE('',*,*,#5528,.F.);
#7278=ORIENTED_EDGE('',*,*,#5529,.T.);
#7279=ORIENTED_EDGE('',*,*,#5530,.F.);
#7280=ORIENTED_EDGE('',*,*,#5529,.F.);
#7281=ORIENTED_EDGE('',*,*,#5531,.F.);
#7282=ORIENTED_EDGE('',*,*,#5532,.T.);
#7283=ORIENTED_EDGE('',*,*,#5533,.F.);
#7284=ORIENTED_EDGE('',*,*,#5534,.T.);
#7285=ORIENTED_EDGE('',*,*,#5531,.T.);
#7286=ORIENTED_EDGE('',*,*,#5534,.F.);
#7287=ORIENTED_EDGE('',*,*,#5532,.F.);
#7288=ORIENTED_EDGE('',*,*,#5535,.T.);
#7289=ORIENTED_EDGE('',*,*,#5536,.F.);
#7290=ORIENTED_EDGE('',*,*,#5535,.F.);
#7291=ORIENTED_EDGE('',*,*,#5537,.F.);
#7292=ORIENTED_EDGE('',*,*,#5538,.T.);
#7293=ORIENTED_EDGE('',*,*,#5539,.F.);
#7294=ORIENTED_EDGE('',*,*,#5540,.T.);
#7295=ORIENTED_EDGE('',*,*,#5537,.T.);
#7296=ORIENTED_EDGE('',*,*,#5540,.F.);
#7297=ORIENTED_EDGE('',*,*,#5538,.F.);
#7298=ORIENTED_EDGE('',*,*,#5541,.T.);
#7299=ORIENTED_EDGE('',*,*,#5542,.F.);
#7300=ORIENTED_EDGE('',*,*,#5541,.F.);
#7301=ORIENTED_EDGE('',*,*,#5448,.F.);
#7302=ORIENTED_EDGE('',*,*,#5543,.T.);
#7303=ORIENTED_EDGE('',*,*,#5489,.T.);
#7304=ORIENTED_EDGE('',*,*,#5544,.T.);
#7305=ORIENTED_EDGE('',*,*,#5524,.T.);
#7306=ORIENTED_EDGE('',*,*,#5545,.T.);
#7307=ORIENTED_EDGE('',*,*,#5521,.F.);
#7308=ORIENTED_EDGE('',*,*,#5546,.F.);
#7309=ORIENTED_EDGE('',*,*,#5544,.F.);
#7310=ORIENTED_EDGE('',*,*,#5488,.F.);
#7311=ORIENTED_EDGE('',*,*,#5492,.F.);
#7312=ORIENTED_EDGE('',*,*,#5495,.F.);
#7313=ORIENTED_EDGE('',*,*,#5498,.F.);
#7314=ORIENTED_EDGE('',*,*,#5501,.F.);
#7315=ORIENTED_EDGE('',*,*,#5504,.F.);
#7316=ORIENTED_EDGE('',*,*,#5507,.F.);
#7317=ORIENTED_EDGE('',*,*,#5510,.F.);
#7318=ORIENTED_EDGE('',*,*,#5513,.F.);
#7319=ORIENTED_EDGE('',*,*,#5516,.F.);
#7320=ORIENTED_EDGE('',*,*,#5519,.F.);
#7321=ORIENTED_EDGE('',*,*,#5522,.F.);
#7322=ORIENTED_EDGE('',*,*,#5545,.F.);
#7323=ORIENTED_EDGE('',*,*,#5527,.F.);
#7324=ORIENTED_EDGE('',*,*,#5547,.F.);
#7325=ORIENTED_EDGE('',*,*,#5484,.F.);
#7326=ORIENTED_EDGE('',*,*,#5548,.F.);
#7327=ORIENTED_EDGE('',*,*,#5482,.F.);
#7328=ORIENTED_EDGE('',*,*,#5479,.F.);
#7329=ORIENTED_EDGE('',*,*,#5476,.F.);
#7330=ORIENTED_EDGE('',*,*,#5473,.F.);
#7331=ORIENTED_EDGE('',*,*,#5470,.F.);
#7332=ORIENTED_EDGE('',*,*,#5467,.F.);
#7333=ORIENTED_EDGE('',*,*,#5464,.F.);
#7334=ORIENTED_EDGE('',*,*,#5461,.F.);
#7335=ORIENTED_EDGE('',*,*,#5458,.F.);
#7336=ORIENTED_EDGE('',*,*,#5455,.F.);
#7337=ORIENTED_EDGE('',*,*,#5452,.F.);
#7338=ORIENTED_EDGE('',*,*,#5449,.F.);
#7339=ORIENTED_EDGE('',*,*,#5543,.F.);
#7340=ORIENTED_EDGE('',*,*,#5447,.F.);
#7341=ORIENTED_EDGE('',*,*,#5454,.F.);
#7342=ORIENTED_EDGE('',*,*,#5457,.F.);
#7343=ORIENTED_EDGE('',*,*,#5460,.F.);
#7344=ORIENTED_EDGE('',*,*,#5463,.F.);
#7345=ORIENTED_EDGE('',*,*,#5466,.F.);
#7346=ORIENTED_EDGE('',*,*,#5469,.F.);
#7347=ORIENTED_EDGE('',*,*,#5472,.F.);
#7348=ORIENTED_EDGE('',*,*,#5475,.F.);
#7349=ORIENTED_EDGE('',*,*,#5478,.F.);
#7350=ORIENTED_EDGE('',*,*,#5481,.F.);
#7351=ORIENTED_EDGE('',*,*,#5549,.F.);
#7352=ORIENTED_EDGE('',*,*,#5486,.F.);
#7353=ORIENTED_EDGE('',*,*,#5550,.F.);
#7354=ORIENTED_EDGE('',*,*,#5525,.T.);
#7355=ORIENTED_EDGE('',*,*,#5546,.T.);
#7356=ORIENTED_EDGE('',*,*,#5523,.T.);
#7357=ORIENTED_EDGE('',*,*,#5520,.T.);
#7358=ORIENTED_EDGE('',*,*,#5517,.T.);
#7359=ORIENTED_EDGE('',*,*,#5514,.T.);
#7360=ORIENTED_EDGE('',*,*,#5511,.T.);
#7361=ORIENTED_EDGE('',*,*,#5508,.T.);
#7362=ORIENTED_EDGE('',*,*,#5505,.T.);
#7363=ORIENTED_EDGE('',*,*,#5502,.T.);
#7364=ORIENTED_EDGE('',*,*,#5499,.T.);
#7365=ORIENTED_EDGE('',*,*,#5496,.T.);
#7366=ORIENTED_EDGE('',*,*,#5493,.T.);
#7367=ORIENTED_EDGE('',*,*,#5490,.T.);
#7368=ORIENTED_EDGE('',*,*,#5483,.T.);
#7369=ORIENTED_EDGE('',*,*,#5549,.T.);
#7370=ORIENTED_EDGE('',*,*,#5480,.F.);
#7371=ORIENTED_EDGE('',*,*,#5548,.T.);
#7372=ORIENTED_EDGE('',*,*,#5366,.F.);
#7373=ORIENTED_EDGE('',*,*,#5551,.T.);
#7374=ORIENTED_EDGE('',*,*,#5407,.T.);
#7375=ORIENTED_EDGE('',*,*,#5552,.T.);
#7376=ORIENTED_EDGE('',*,*,#5442,.T.);
#7377=ORIENTED_EDGE('',*,*,#5553,.T.);
#7378=ORIENTED_EDGE('',*,*,#5439,.F.);
#7379=ORIENTED_EDGE('',*,*,#5554,.F.);
#7380=ORIENTED_EDGE('',*,*,#5552,.F.);
#7381=ORIENTED_EDGE('',*,*,#5406,.F.);
#7382=ORIENTED_EDGE('',*,*,#5410,.F.);
#7383=ORIENTED_EDGE('',*,*,#5413,.F.);
#7384=ORIENTED_EDGE('',*,*,#5416,.F.);
#7385=ORIENTED_EDGE('',*,*,#5419,.F.);
#7386=ORIENTED_EDGE('',*,*,#5422,.F.);
#7387=ORIENTED_EDGE('',*,*,#5425,.F.);
#7388=ORIENTED_EDGE('',*,*,#5428,.F.);
#7389=ORIENTED_EDGE('',*,*,#5431,.F.);
#7390=ORIENTED_EDGE('',*,*,#5434,.F.);
#7391=ORIENTED_EDGE('',*,*,#5437,.F.);
#7392=ORIENTED_EDGE('',*,*,#5440,.F.);
#7393=ORIENTED_EDGE('',*,*,#5553,.F.);
#7394=ORIENTED_EDGE('',*,*,#5445,.F.);
#7395=ORIENTED_EDGE('',*,*,#5555,.F.);
#7396=ORIENTED_EDGE('',*,*,#5402,.F.);
#7397=ORIENTED_EDGE('',*,*,#5556,.F.);
#7398=ORIENTED_EDGE('',*,*,#5400,.F.);
#7399=ORIENTED_EDGE('',*,*,#5397,.F.);
#7400=ORIENTED_EDGE('',*,*,#5394,.F.);
#7401=ORIENTED_EDGE('',*,*,#5391,.F.);
#7402=ORIENTED_EDGE('',*,*,#5388,.F.);
#7403=ORIENTED_EDGE('',*,*,#5385,.F.);
#7404=ORIENTED_EDGE('',*,*,#5382,.F.);
#7405=ORIENTED_EDGE('',*,*,#5379,.F.);
#7406=ORIENTED_EDGE('',*,*,#5376,.F.);
#7407=ORIENTED_EDGE('',*,*,#5373,.F.);
#7408=ORIENTED_EDGE('',*,*,#5370,.F.);
#7409=ORIENTED_EDGE('',*,*,#5367,.F.);
#7410=ORIENTED_EDGE('',*,*,#5551,.F.);
#7411=ORIENTED_EDGE('',*,*,#5365,.F.);
#7412=ORIENTED_EDGE('',*,*,#5372,.F.);
#7413=ORIENTED_EDGE('',*,*,#5375,.F.);
#7414=ORIENTED_EDGE('',*,*,#5378,.F.);
#7415=ORIENTED_EDGE('',*,*,#5381,.F.);
#7416=ORIENTED_EDGE('',*,*,#5384,.F.);
#7417=ORIENTED_EDGE('',*,*,#5387,.F.);
#7418=ORIENTED_EDGE('',*,*,#5390,.F.);
#7419=ORIENTED_EDGE('',*,*,#5393,.F.);
#7420=ORIENTED_EDGE('',*,*,#5396,.F.);
#7421=ORIENTED_EDGE('',*,*,#5399,.F.);
#7422=ORIENTED_EDGE('',*,*,#5557,.F.);
#7423=ORIENTED_EDGE('',*,*,#5404,.F.);
#7424=ORIENTED_EDGE('',*,*,#5558,.F.);
#7425=ORIENTED_EDGE('',*,*,#5443,.T.);
#7426=ORIENTED_EDGE('',*,*,#5554,.T.);
#7427=ORIENTED_EDGE('',*,*,#5441,.T.);
#7428=ORIENTED_EDGE('',*,*,#5438,.T.);
#7429=ORIENTED_EDGE('',*,*,#5435,.T.);
#7430=ORIENTED_EDGE('',*,*,#5432,.T.);
#7431=ORIENTED_EDGE('',*,*,#5429,.T.);
#7432=ORIENTED_EDGE('',*,*,#5426,.T.);
#7433=ORIENTED_EDGE('',*,*,#5423,.T.);
#7434=ORIENTED_EDGE('',*,*,#5420,.T.);
#7435=ORIENTED_EDGE('',*,*,#5417,.T.);
#7436=ORIENTED_EDGE('',*,*,#5414,.T.);
#7437=ORIENTED_EDGE('',*,*,#5411,.T.);
#7438=ORIENTED_EDGE('',*,*,#5408,.T.);
#7439=ORIENTED_EDGE('',*,*,#5401,.T.);
#7440=ORIENTED_EDGE('',*,*,#5557,.T.);
#7441=ORIENTED_EDGE('',*,*,#5398,.F.);
#7442=ORIENTED_EDGE('',*,*,#5556,.T.);
#7443=ORIENTED_EDGE('',*,*,#5284,.F.);
#7444=ORIENTED_EDGE('',*,*,#5559,.T.);
#7445=ORIENTED_EDGE('',*,*,#5325,.T.);
#7446=ORIENTED_EDGE('',*,*,#5560,.T.);
#7447=ORIENTED_EDGE('',*,*,#5360,.T.);
#7448=ORIENTED_EDGE('',*,*,#5561,.T.);
#7449=ORIENTED_EDGE('',*,*,#5357,.F.);
#7450=ORIENTED_EDGE('',*,*,#5562,.F.);
#7451=ORIENTED_EDGE('',*,*,#5560,.F.);
#7452=ORIENTED_EDGE('',*,*,#5324,.F.);
#7453=ORIENTED_EDGE('',*,*,#5328,.F.);
#7454=ORIENTED_EDGE('',*,*,#5331,.F.);
#7455=ORIENTED_EDGE('',*,*,#5334,.F.);
#7456=ORIENTED_EDGE('',*,*,#5337,.F.);
#7457=ORIENTED_EDGE('',*,*,#5340,.F.);
#7458=ORIENTED_EDGE('',*,*,#5343,.F.);
#7459=ORIENTED_EDGE('',*,*,#5346,.F.);
#7460=ORIENTED_EDGE('',*,*,#5349,.F.);
#7461=ORIENTED_EDGE('',*,*,#5352,.F.);
#7462=ORIENTED_EDGE('',*,*,#5355,.F.);
#7463=ORIENTED_EDGE('',*,*,#5358,.F.);
#7464=ORIENTED_EDGE('',*,*,#5561,.F.);
#7465=ORIENTED_EDGE('',*,*,#5363,.F.);
#7466=ORIENTED_EDGE('',*,*,#5563,.F.);
#7467=ORIENTED_EDGE('',*,*,#5320,.F.);
#7468=ORIENTED_EDGE('',*,*,#5564,.F.);
#7469=ORIENTED_EDGE('',*,*,#5318,.F.);
#7470=ORIENTED_EDGE('',*,*,#5315,.F.);
#7471=ORIENTED_EDGE('',*,*,#5312,.F.);
#7472=ORIENTED_EDGE('',*,*,#5309,.F.);
#7473=ORIENTED_EDGE('',*,*,#5306,.F.);
#7474=ORIENTED_EDGE('',*,*,#5303,.F.);
#7475=ORIENTED_EDGE('',*,*,#5300,.F.);
#7476=ORIENTED_EDGE('',*,*,#5297,.F.);
#7477=ORIENTED_EDGE('',*,*,#5294,.F.);
#7478=ORIENTED_EDGE('',*,*,#5291,.F.);
#7479=ORIENTED_EDGE('',*,*,#5288,.F.);
#7480=ORIENTED_EDGE('',*,*,#5285,.F.);
#7481=ORIENTED_EDGE('',*,*,#5559,.F.);
#7482=ORIENTED_EDGE('',*,*,#5283,.F.);
#7483=ORIENTED_EDGE('',*,*,#5290,.F.);
#7484=ORIENTED_EDGE('',*,*,#5293,.F.);
#7485=ORIENTED_EDGE('',*,*,#5296,.F.);
#7486=ORIENTED_EDGE('',*,*,#5299,.F.);
#7487=ORIENTED_EDGE('',*,*,#5302,.F.);
#7488=ORIENTED_EDGE('',*,*,#5305,.F.);
#7489=ORIENTED_EDGE('',*,*,#5308,.F.);
#7490=ORIENTED_EDGE('',*,*,#5311,.F.);
#7491=ORIENTED_EDGE('',*,*,#5314,.F.);
#7492=ORIENTED_EDGE('',*,*,#5317,.F.);
#7493=ORIENTED_EDGE('',*,*,#5565,.F.);
#7494=ORIENTED_EDGE('',*,*,#5322,.F.);
#7495=ORIENTED_EDGE('',*,*,#5566,.F.);
#7496=ORIENTED_EDGE('',*,*,#5361,.T.);
#7497=ORIENTED_EDGE('',*,*,#5562,.T.);
#7498=ORIENTED_EDGE('',*,*,#5359,.T.);
#7499=ORIENTED_EDGE('',*,*,#5356,.T.);
#7500=ORIENTED_EDGE('',*,*,#5353,.T.);
#7501=ORIENTED_EDGE('',*,*,#5350,.T.);
#7502=ORIENTED_EDGE('',*,*,#5347,.T.);
#7503=ORIENTED_EDGE('',*,*,#5344,.T.);
#7504=ORIENTED_EDGE('',*,*,#5341,.T.);
#7505=ORIENTED_EDGE('',*,*,#5338,.T.);
#7506=ORIENTED_EDGE('',*,*,#5335,.T.);
#7507=ORIENTED_EDGE('',*,*,#5332,.T.);
#7508=ORIENTED_EDGE('',*,*,#5329,.T.);
#7509=ORIENTED_EDGE('',*,*,#5326,.T.);
#7510=ORIENTED_EDGE('',*,*,#5319,.T.);
#7511=ORIENTED_EDGE('',*,*,#5565,.T.);
#7512=ORIENTED_EDGE('',*,*,#5316,.F.);
#7513=ORIENTED_EDGE('',*,*,#5564,.T.);
#7514=ORIENTED_EDGE('',*,*,#5202,.F.);
#7515=ORIENTED_EDGE('',*,*,#5567,.T.);
#7516=ORIENTED_EDGE('',*,*,#5243,.T.);
#7517=ORIENTED_EDGE('',*,*,#5568,.T.);
#7518=ORIENTED_EDGE('',*,*,#5278,.T.);
#7519=ORIENTED_EDGE('',*,*,#5569,.T.);
#7520=ORIENTED_EDGE('',*,*,#5275,.F.);
#7521=ORIENTED_EDGE('',*,*,#5570,.F.);
#7522=ORIENTED_EDGE('',*,*,#5568,.F.);
#7523=ORIENTED_EDGE('',*,*,#5242,.F.);
#7524=ORIENTED_EDGE('',*,*,#5246,.F.);
#7525=ORIENTED_EDGE('',*,*,#5249,.F.);
#7526=ORIENTED_EDGE('',*,*,#5252,.F.);
#7527=ORIENTED_EDGE('',*,*,#5255,.F.);
#7528=ORIENTED_EDGE('',*,*,#5258,.F.);
#7529=ORIENTED_EDGE('',*,*,#5261,.F.);
#7530=ORIENTED_EDGE('',*,*,#5264,.F.);
#7531=ORIENTED_EDGE('',*,*,#5267,.F.);
#7532=ORIENTED_EDGE('',*,*,#5270,.F.);
#7533=ORIENTED_EDGE('',*,*,#5273,.F.);
#7534=ORIENTED_EDGE('',*,*,#5276,.F.);
#7535=ORIENTED_EDGE('',*,*,#5569,.F.);
#7536=ORIENTED_EDGE('',*,*,#5281,.F.);
#7537=ORIENTED_EDGE('',*,*,#5571,.F.);
#7538=ORIENTED_EDGE('',*,*,#5238,.F.);
#7539=ORIENTED_EDGE('',*,*,#5572,.F.);
#7540=ORIENTED_EDGE('',*,*,#5236,.F.);
#7541=ORIENTED_EDGE('',*,*,#5233,.F.);
#7542=ORIENTED_EDGE('',*,*,#5230,.F.);
#7543=ORIENTED_EDGE('',*,*,#5227,.F.);
#7544=ORIENTED_EDGE('',*,*,#5224,.F.);
#7545=ORIENTED_EDGE('',*,*,#5221,.F.);
#7546=ORIENTED_EDGE('',*,*,#5218,.F.);
#7547=ORIENTED_EDGE('',*,*,#5215,.F.);
#7548=ORIENTED_EDGE('',*,*,#5212,.F.);
#7549=ORIENTED_EDGE('',*,*,#5209,.F.);
#7550=ORIENTED_EDGE('',*,*,#5206,.F.);
#7551=ORIENTED_EDGE('',*,*,#5203,.F.);
#7552=ORIENTED_EDGE('',*,*,#5567,.F.);
#7553=ORIENTED_EDGE('',*,*,#5201,.F.);
#7554=ORIENTED_EDGE('',*,*,#5208,.F.);
#7555=ORIENTED_EDGE('',*,*,#5211,.F.);
#7556=ORIENTED_EDGE('',*,*,#5214,.F.);
#7557=ORIENTED_EDGE('',*,*,#5217,.F.);
#7558=ORIENTED_EDGE('',*,*,#5220,.F.);
#7559=ORIENTED_EDGE('',*,*,#5223,.F.);
#7560=ORIENTED_EDGE('',*,*,#5226,.F.);
#7561=ORIENTED_EDGE('',*,*,#5229,.F.);
#7562=ORIENTED_EDGE('',*,*,#5232,.F.);
#7563=ORIENTED_EDGE('',*,*,#5235,.F.);
#7564=ORIENTED_EDGE('',*,*,#5573,.F.);
#7565=ORIENTED_EDGE('',*,*,#5240,.F.);
#7566=ORIENTED_EDGE('',*,*,#5574,.F.);
#7567=ORIENTED_EDGE('',*,*,#5279,.T.);
#7568=ORIENTED_EDGE('',*,*,#5570,.T.);
#7569=ORIENTED_EDGE('',*,*,#5277,.T.);
#7570=ORIENTED_EDGE('',*,*,#5274,.T.);
#7571=ORIENTED_EDGE('',*,*,#5271,.T.);
#7572=ORIENTED_EDGE('',*,*,#5268,.T.);
#7573=ORIENTED_EDGE('',*,*,#5265,.T.);
#7574=ORIENTED_EDGE('',*,*,#5262,.T.);
#7575=ORIENTED_EDGE('',*,*,#5259,.T.);
#7576=ORIENTED_EDGE('',*,*,#5256,.T.);
#7577=ORIENTED_EDGE('',*,*,#5253,.T.);
#7578=ORIENTED_EDGE('',*,*,#5250,.T.);
#7579=ORIENTED_EDGE('',*,*,#5247,.T.);
#7580=ORIENTED_EDGE('',*,*,#5244,.T.);
#7581=ORIENTED_EDGE('',*,*,#5237,.T.);
#7582=ORIENTED_EDGE('',*,*,#5573,.T.);
#7583=ORIENTED_EDGE('',*,*,#5234,.F.);
#7584=ORIENTED_EDGE('',*,*,#5572,.T.);
#7585=ORIENTED_EDGE('',*,*,#5287,.F.);
#7586=ORIENTED_EDGE('',*,*,#5205,.F.);
#7587=ORIENTED_EDGE('',*,*,#5451,.F.);
#7588=ORIENTED_EDGE('',*,*,#5369,.F.);
#7589=ORIENTED_EDGE('',*,*,#5575,.F.);
#7590=ORIENTED_EDGE('',*,*,#5576,.T.);
#7591=ORIENTED_EDGE('',*,*,#5577,.F.);
#7592=ORIENTED_EDGE('',*,*,#5576,.F.);
#7593=ORIENTED_EDGE('',*,*,#5578,.F.);
#7594=ORIENTED_EDGE('',*,*,#5579,.T.);
#7595=ORIENTED_EDGE('',*,*,#5580,.F.);
#7596=ORIENTED_EDGE('',*,*,#5579,.F.);
#7597=ORIENTED_EDGE('',*,*,#5581,.T.);
#7598=ORIENTED_EDGE('',*,*,#5582,.F.);
#7599=ORIENTED_EDGE('',*,*,#5583,.F.);
#7600=ORIENTED_EDGE('',*,*,#5584,.F.);
#7601=ORIENTED_EDGE('',*,*,#5585,.T.);
#7602=ORIENTED_EDGE('',*,*,#5584,.T.);
#7603=ORIENTED_EDGE('',*,*,#5586,.F.);
#7604=ORIENTED_EDGE('',*,*,#5587,.F.);
#7605=ORIENTED_EDGE('',*,*,#5588,.T.);
#7606=ORIENTED_EDGE('',*,*,#5587,.T.);
#7607=ORIENTED_EDGE('',*,*,#5589,.F.);
#7608=ORIENTED_EDGE('',*,*,#5590,.F.);
#7609=ORIENTED_EDGE('',*,*,#5591,.F.);
#7610=ORIENTED_EDGE('',*,*,#5589,.T.);
#7611=ORIENTED_EDGE('',*,*,#5586,.T.);
#7612=ORIENTED_EDGE('',*,*,#5583,.T.);
#7613=ORIENTED_EDGE('',*,*,#5578,.T.);
#7614=ORIENTED_EDGE('',*,*,#5592,.T.);
#7615=ORIENTED_EDGE('',*,*,#5593,.T.);
#7616=ORIENTED_EDGE('',*,*,#5594,.F.);
#7617=ORIENTED_EDGE('',*,*,#5595,.F.);
#7618=ORIENTED_EDGE('',*,*,#5596,.T.);
#7619=ORIENTED_EDGE('',*,*,#5597,.F.);
#7620=ORIENTED_EDGE('',*,*,#5598,.F.);
#7621=ORIENTED_EDGE('',*,*,#5599,.F.);
#7622=ORIENTED_EDGE('',*,*,#5600,.T.);
#7623=ORIENTED_EDGE('',*,*,#5599,.T.);
#7624=ORIENTED_EDGE('',*,*,#5601,.F.);
#7625=ORIENTED_EDGE('',*,*,#5593,.F.);
#7626=ORIENTED_EDGE('',*,*,#5601,.T.);
#7627=ORIENTED_EDGE('',*,*,#5598,.T.);
#7628=ORIENTED_EDGE('',*,*,#5602,.F.);
#7629=ORIENTED_EDGE('',*,*,#5594,.T.);
#7630=ORIENTED_EDGE('',*,*,#5575,.T.);
#7631=ORIENTED_EDGE('',*,*,#5603,.F.);
#7632=ORIENTED_EDGE('',*,*,#5604,.T.);
#7633=ORIENTED_EDGE('',*,*,#5605,.F.);
#7634=ORIENTED_EDGE('',*,*,#5604,.F.);
#7635=ORIENTED_EDGE('',*,*,#5606,.F.);
#7636=ORIENTED_EDGE('',*,*,#5607,.T.);
#7637=ORIENTED_EDGE('',*,*,#5608,.F.);
#7638=ORIENTED_EDGE('',*,*,#5607,.F.);
#7639=ORIENTED_EDGE('',*,*,#5606,.T.);
#7640=ORIENTED_EDGE('',*,*,#5603,.T.);
#7641=ORIENTED_EDGE('',*,*,#5609,.T.);
#7642=ORIENTED_EDGE('',*,*,#5610,.F.);
#7643=ORIENTED_EDGE('',*,*,#5611,.T.);
#7644=ORIENTED_EDGE('',*,*,#5612,.F.);
#7645=ORIENTED_EDGE('',*,*,#5613,.T.);
#7646=ORIENTED_EDGE('',*,*,#5614,.F.);
#7647=ORIENTED_EDGE('',*,*,#5615,.T.);
#7648=ORIENTED_EDGE('',*,*,#5616,.F.);
#7649=ORIENTED_EDGE('',*,*,#5536,.T.);
#7650=ORIENTED_EDGE('',*,*,#5542,.T.);
#7651=ORIENTED_EDGE('',*,*,#5608,.T.);
#7652=ORIENTED_EDGE('',*,*,#5609,.F.);
#7653=ORIENTED_EDGE('',*,*,#5617,.T.);
#7654=ORIENTED_EDGE('',*,*,#5618,.T.);
#7655=ORIENTED_EDGE('',*,*,#5619,.T.);
#7656=ORIENTED_EDGE('',*,*,#5617,.F.);
#7657=ORIENTED_EDGE('',*,*,#5616,.T.);
#7658=ORIENTED_EDGE('',*,*,#5620,.F.);
#7659=ORIENTED_EDGE('',*,*,#5621,.F.);
#7660=ORIENTED_EDGE('',*,*,#5615,.F.);
#7661=ORIENTED_EDGE('',*,*,#5622,.T.);
#7662=ORIENTED_EDGE('',*,*,#5623,.T.);
#7663=ORIENTED_EDGE('',*,*,#5620,.T.);
#7664=ORIENTED_EDGE('',*,*,#5622,.F.);
#7665=ORIENTED_EDGE('',*,*,#5614,.T.);
#7666=ORIENTED_EDGE('',*,*,#5624,.F.);
#7667=ORIENTED_EDGE('',*,*,#5625,.F.);
#7668=ORIENTED_EDGE('',*,*,#5611,.F.);
#7669=ORIENTED_EDGE('',*,*,#5626,.T.);
#7670=ORIENTED_EDGE('',*,*,#5627,.T.);
#7671=ORIENTED_EDGE('',*,*,#5628,.T.);
#7672=ORIENTED_EDGE('',*,*,#5605,.T.);
#7673=ORIENTED_EDGE('',*,*,#5628,.F.);
#7674=ORIENTED_EDGE('',*,*,#5629,.F.);
#7675=ORIENTED_EDGE('',*,*,#5630,.F.);
#7676=ORIENTED_EDGE('',*,*,#5612,.T.);
#7677=ORIENTED_EDGE('',*,*,#5530,.T.);
#7678=ORIENTED_EDGE('',*,*,#5613,.F.);
#7679=ORIENTED_EDGE('',*,*,#5630,.T.);
#7680=ORIENTED_EDGE('',*,*,#5631,.T.);
#7681=ORIENTED_EDGE('',*,*,#5624,.T.);
#7682=ORIENTED_EDGE('',*,*,#5619,.F.);
#7683=ORIENTED_EDGE('',*,*,#5632,.F.);
#7684=ORIENTED_EDGE('',*,*,#5626,.F.);
#7685=ORIENTED_EDGE('',*,*,#5610,.T.);
#7686=ORIENTED_EDGE('',*,*,#5633,.T.);
#7687=ORIENTED_EDGE('',*,*,#5634,.T.);
#7688=ORIENTED_EDGE('',*,*,#5635,.F.);
#7689=ORIENTED_EDGE('',*,*,#5636,.F.);
#7690=ORIENTED_EDGE('',*,*,#5582,.T.);
#7691=ORIENTED_EDGE('',*,*,#5637,.T.);
#7692=ORIENTED_EDGE('',*,*,#5636,.T.);
#7693=ORIENTED_EDGE('',*,*,#5638,.F.);
#7694=ORIENTED_EDGE('',*,*,#5639,.F.);
#7695=ORIENTED_EDGE('',*,*,#5640,.T.);
#7696=ORIENTED_EDGE('',*,*,#5590,.T.);
#7697=ORIENTED_EDGE('',*,*,#5591,.T.);
#7698=ORIENTED_EDGE('',*,*,#5641,.T.);
#7699=ORIENTED_EDGE('',*,*,#5639,.T.);
#7700=ORIENTED_EDGE('',*,*,#5642,.F.);
#7701=ORIENTED_EDGE('',*,*,#5643,.F.);
#7702=ORIENTED_EDGE('',*,*,#5528,.T.);
#7703=ORIENTED_EDGE('',*,*,#5597,.T.);
#7704=ORIENTED_EDGE('',*,*,#5644,.T.);
#7705=ORIENTED_EDGE('',*,*,#5643,.T.);
#7706=ORIENTED_EDGE('',*,*,#5645,.F.);
#7707=ORIENTED_EDGE('',*,*,#5634,.F.);
#7708=ORIENTED_EDGE('',*,*,#5646,.T.);
#7709=ORIENTED_EDGE('',*,*,#5595,.T.);
#7710=ORIENTED_EDGE('',*,*,#5602,.T.);
#7711=ORIENTED_EDGE('',*,*,#5645,.T.);
#7712=ORIENTED_EDGE('',*,*,#5642,.T.);
#7713=ORIENTED_EDGE('',*,*,#5638,.T.);
#7714=ORIENTED_EDGE('',*,*,#5635,.T.);
#7715=ORIENTED_EDGE('',*,*,#5550,.T.);
#7716=ORIENTED_EDGE('',*,*,#5485,.T.);
#7717=ORIENTED_EDGE('',*,*,#5547,.T.);
#7718=ORIENTED_EDGE('',*,*,#5526,.T.);
#7719=ORIENTED_EDGE('',*,*,#5558,.T.);
#7720=ORIENTED_EDGE('',*,*,#5403,.T.);
#7721=ORIENTED_EDGE('',*,*,#5555,.T.);
#7722=ORIENTED_EDGE('',*,*,#5444,.T.);
#7723=ORIENTED_EDGE('',*,*,#5566,.T.);
#7724=ORIENTED_EDGE('',*,*,#5321,.T.);
#7725=ORIENTED_EDGE('',*,*,#5563,.T.);
#7726=ORIENTED_EDGE('',*,*,#5362,.T.);
#7727=ORIENTED_EDGE('',*,*,#5574,.T.);
#7728=ORIENTED_EDGE('',*,*,#5239,.T.);
#7729=ORIENTED_EDGE('',*,*,#5571,.T.);
#7730=ORIENTED_EDGE('',*,*,#5280,.T.);
#7731=ORIENTED_EDGE('',*,*,#5629,.T.);
#7732=ORIENTED_EDGE('',*,*,#5627,.F.);
#7733=ORIENTED_EDGE('',*,*,#5632,.T.);
#7734=ORIENTED_EDGE('',*,*,#5618,.F.);
#7735=ORIENTED_EDGE('',*,*,#5621,.T.);
#7736=ORIENTED_EDGE('',*,*,#5623,.F.);
#7737=ORIENTED_EDGE('',*,*,#5625,.T.);
#7738=ORIENTED_EDGE('',*,*,#5631,.F.);
#7739=ORIENTED_EDGE('',*,*,#5646,.F.);
#7740=ORIENTED_EDGE('',*,*,#5633,.F.);
#7741=ORIENTED_EDGE('',*,*,#5637,.F.);
#7742=ORIENTED_EDGE('',*,*,#5581,.F.);
#7743=ORIENTED_EDGE('',*,*,#5585,.F.);
#7744=ORIENTED_EDGE('',*,*,#5588,.F.);
#7745=ORIENTED_EDGE('',*,*,#5640,.F.);
#7746=ORIENTED_EDGE('',*,*,#5641,.F.);
#7747=ORIENTED_EDGE('',*,*,#5644,.F.);
#7748=ORIENTED_EDGE('',*,*,#5596,.F.);
#7749=ORIENTED_EDGE('',*,*,#5600,.F.);
#7750=ORIENTED_EDGE('',*,*,#5592,.F.);
#7751=ORIENTED_EDGE('',*,*,#5533,.T.);
#7752=ORIENTED_EDGE('',*,*,#5539,.T.);
#7753=ORIENTED_EDGE('',*,*,#5577,.T.);
#7754=ORIENTED_EDGE('',*,*,#5580,.T.);
#10183=CYLINDRICAL_SURFACE('',#11438,0.1666);
#10184=CYLINDRICAL_SURFACE('',#11441,0.1666);
#10185=CYLINDRICAL_SURFACE('',#11442,0.1666);
#10186=CYLINDRICAL_SURFACE('',#11443,0.1666);
#10187=CYLINDRICAL_SURFACE('',#11444,0.1666);
#10188=CYLINDRICAL_SURFACE('',#11445,0.1666);
#10189=CYLINDRICAL_SURFACE('',#11446,0.1666);
#10190=CYLINDRICAL_SURFACE('',#11447,0.1666);
#10191=CYLINDRICAL_SURFACE('',#11448,0.1666);
#10192=CYLINDRICAL_SURFACE('',#11449,0.1666);
#10193=CYLINDRICAL_SURFACE('',#11450,0.1666);
#10194=CYLINDRICAL_SURFACE('',#11451,0.1666);
#10195=CYLINDRICAL_SURFACE('',#11453,0.205475000000001);
#10196=CYLINDRICAL_SURFACE('',#11455,0.205475000000001);
#10197=CYLINDRICAL_SURFACE('',#11456,0.205475000000001);
#10198=CYLINDRICAL_SURFACE('',#11457,0.205475000000001);
#10199=CYLINDRICAL_SURFACE('',#11458,0.205475000000001);
#10200=CYLINDRICAL_SURFACE('',#11459,0.205475000000001);
#10201=CYLINDRICAL_SURFACE('',#11460,0.205475000000001);
#10202=CYLINDRICAL_SURFACE('',#11461,0.205475000000001);
#10203=CYLINDRICAL_SURFACE('',#11462,0.205475000000001);
#10204=CYLINDRICAL_SURFACE('',#11463,0.205475000000001);
#10205=CYLINDRICAL_SURFACE('',#11464,0.205475000000001);
#10206=CYLINDRICAL_SURFACE('',#11465,0.205475000000001);
#10207=CYLINDRICAL_SURFACE('',#11466,0.205475000000001);
#10208=CYLINDRICAL_SURFACE('',#11468,0.1666);
#10209=CYLINDRICAL_SURFACE('',#11471,0.1666);
#10210=CYLINDRICAL_SURFACE('',#11472,0.1666);
#10211=CYLINDRICAL_SURFACE('',#11473,0.1666);
#10212=CYLINDRICAL_SURFACE('',#11474,0.1666);
#10213=CYLINDRICAL_SURFACE('',#11475,0.1666);
#10214=CYLINDRICAL_SURFACE('',#11476,0.1666);
#10215=CYLINDRICAL_SURFACE('',#11477,0.1666);
#10216=CYLINDRICAL_SURFACE('',#11478,0.1666);
#10217=CYLINDRICAL_SURFACE('',#11479,0.1666);
#10218=CYLINDRICAL_SURFACE('',#11480,0.1666);
#10219=CYLINDRICAL_SURFACE('',#11481,0.1666);
#10220=CYLINDRICAL_SURFACE('',#11483,0.205475000000001);
#10221=CYLINDRICAL_SURFACE('',#11485,0.205475000000001);
#10222=CYLINDRICAL_SURFACE('',#11486,0.205475000000001);
#10223=CYLINDRICAL_SURFACE('',#11487,0.205475000000001);
#10224=CYLINDRICAL_SURFACE('',#11488,0.205475000000001);
#10225=CYLINDRICAL_SURFACE('',#11489,0.205475000000001);
#10226=CYLINDRICAL_SURFACE('',#11490,0.205475000000001);
#10227=CYLINDRICAL_SURFACE('',#11491,0.205475000000001);
#10228=CYLINDRICAL_SURFACE('',#11492,0.205475000000001);
#10229=CYLINDRICAL_SURFACE('',#11493,0.205475000000001);
#10230=CYLINDRICAL_SURFACE('',#11494,0.205475000000001);
#10231=CYLINDRICAL_SURFACE('',#11495,0.205475000000001);
#10232=CYLINDRICAL_SURFACE('',#11496,0.205475000000001);
#10233=CYLINDRICAL_SURFACE('',#11498,0.1666);
#10234=CYLINDRICAL_SURFACE('',#11501,0.1666);
#10235=CYLINDRICAL_SURFACE('',#11502,0.1666);
#10236=CYLINDRICAL_SURFACE('',#11503,0.1666);
#10237=CYLINDRICAL_SURFACE('',#11504,0.1666);
#10238=CYLINDRICAL_SURFACE('',#11505,0.1666);
#10239=CYLINDRICAL_SURFACE('',#11506,0.1666);
#10240=CYLINDRICAL_SURFACE('',#11507,0.1666);
#10241=CYLINDRICAL_SURFACE('',#11508,0.1666);
#10242=CYLINDRICAL_SURFACE('',#11509,0.1666);
#10243=CYLINDRICAL_SURFACE('',#11510,0.1666);
#10244=CYLINDRICAL_SURFACE('',#11511,0.1666);
#10245=CYLINDRICAL_SURFACE('',#11513,0.205475);
#10246=CYLINDRICAL_SURFACE('',#11515,0.205475);
#10247=CYLINDRICAL_SURFACE('',#11516,0.205475);
#10248=CYLINDRICAL_SURFACE('',#11517,0.205475);
#10249=CYLINDRICAL_SURFACE('',#11518,0.205475);
#10250=CYLINDRICAL_SURFACE('',#11519,0.205475);
#10251=CYLINDRICAL_SURFACE('',#11520,0.205475);
#10252=CYLINDRICAL_SURFACE('',#11521,0.205475);
#10253=CYLINDRICAL_SURFACE('',#11522,0.205475);
#10254=CYLINDRICAL_SURFACE('',#11523,0.205475);
#10255=CYLINDRICAL_SURFACE('',#11524,0.205475);
#10256=CYLINDRICAL_SURFACE('',#11525,0.205475);
#10257=CYLINDRICAL_SURFACE('',#11526,0.205475);
#10258=CYLINDRICAL_SURFACE('',#11528,0.1666);
#10259=CYLINDRICAL_SURFACE('',#11531,0.1666);
#10260=CYLINDRICAL_SURFACE('',#11532,0.1666);
#10261=CYLINDRICAL_SURFACE('',#11533,0.1666);
#10262=CYLINDRICAL_SURFACE('',#11534,0.1666);
#10263=CYLINDRICAL_SURFACE('',#11535,0.1666);
#10264=CYLINDRICAL_SURFACE('',#11536,0.1666);
#10265=CYLINDRICAL_SURFACE('',#11537,0.1666);
#10266=CYLINDRICAL_SURFACE('',#11538,0.1666);
#10267=CYLINDRICAL_SURFACE('',#11539,0.1666);
#10268=CYLINDRICAL_SURFACE('',#11540,0.1666);
#10269=CYLINDRICAL_SURFACE('',#11541,0.1666);
#10270=CYLINDRICAL_SURFACE('',#11543,0.205475);
#10271=CYLINDRICAL_SURFACE('',#11545,0.205475);
#10272=CYLINDRICAL_SURFACE('',#11546,0.205475);
#10273=CYLINDRICAL_SURFACE('',#11547,0.205475);
#10274=CYLINDRICAL_SURFACE('',#11548,0.205475);
#10275=CYLINDRICAL_SURFACE('',#11549,0.205475);
#10276=CYLINDRICAL_SURFACE('',#11550,0.205475);
#10277=CYLINDRICAL_SURFACE('',#11551,0.205475);
#10278=CYLINDRICAL_SURFACE('',#11552,0.205475);
#10279=CYLINDRICAL_SURFACE('',#11553,0.205475);
#10280=CYLINDRICAL_SURFACE('',#11554,0.205475);
#10281=CYLINDRICAL_SURFACE('',#11555,0.205475);
#10282=CYLINDRICAL_SURFACE('',#11556,0.205475);
#10283=CYLINDRICAL_SURFACE('',#11558,0.6);
#10284=CYLINDRICAL_SURFACE('',#11564,0.4);
#10285=CYLINDRICAL_SURFACE('',#11566,0.25);
#10286=CYLINDRICAL_SURFACE('',#11571,0.4);
#10287=CYLINDRICAL_SURFACE('',#11573,0.25);
#10288=CYLINDRICAL_SURFACE('',#11576,0.205475);
#10289=CYLINDRICAL_SURFACE('',#11577,0.1666);
#10290=CYLINDRICAL_SURFACE('',#11579,0.205475);
#10291=CYLINDRICAL_SURFACE('',#11580,0.1666);
#10292=CYLINDRICAL_SURFACE('',#11582,0.205475000000001);
#10293=CYLINDRICAL_SURFACE('',#11583,0.1666);
#10294=CYLINDRICAL_SURFACE('',#11585,0.205475000000001);
#10295=CYLINDRICAL_SURFACE('',#11586,0.1666);
#10296=CYLINDRICAL_SURFACE('',#11591,0.3);
#10297=CYLINDRICAL_SURFACE('',#11594,0.3);
#10298=CYLINDRICAL_SURFACE('',#11605,0.65);
#10299=CYLINDRICAL_SURFACE('',#11608,0.8);
#10300=CYLINDRICAL_SURFACE('',#11617,0.2);
#10301=CYLINDRICAL_SURFACE('',#11620,0.2);
#10302=CYLINDRICAL_SURFACE('',#11623,0.2);
#10303=CYLINDRICAL_SURFACE('',#11627,0.2);
#10609=ADVANCED_FACE('',(#484),#10183,.F.);
#10610=ADVANCED_FACE('',(#485),#10184,.F.);
#10611=ADVANCED_FACE('',(#486),#10185,.F.);
#10612=ADVANCED_FACE('',(#487),#10186,.F.);
#10613=ADVANCED_FACE('',(#488),#10187,.F.);
#10614=ADVANCED_FACE('',(#489),#10188,.F.);
#10615=ADVANCED_FACE('',(#490),#10189,.F.);
#10616=ADVANCED_FACE('',(#491),#10190,.F.);
#10617=ADVANCED_FACE('',(#492),#10191,.F.);
#10618=ADVANCED_FACE('',(#493),#10192,.F.);
#10619=ADVANCED_FACE('',(#494),#10193,.F.);
#10620=ADVANCED_FACE('',(#495),#10194,.F.);
#10621=ADVANCED_FACE('',(#496),#10195,.F.);
#10622=ADVANCED_FACE('',(#497),#10196,.F.);
#10623=ADVANCED_FACE('',(#498),#10197,.F.);
#10624=ADVANCED_FACE('',(#499),#10198,.F.);
#10625=ADVANCED_FACE('',(#500),#10199,.F.);
#10626=ADVANCED_FACE('',(#501),#10200,.F.);
#10627=ADVANCED_FACE('',(#502),#10201,.F.);
#10628=ADVANCED_FACE('',(#503),#10202,.F.);
#10629=ADVANCED_FACE('',(#504),#10203,.F.);
#10630=ADVANCED_FACE('',(#505),#10204,.F.);
#10631=ADVANCED_FACE('',(#506),#10205,.F.);
#10632=ADVANCED_FACE('',(#507),#10206,.F.);
#10633=ADVANCED_FACE('',(#508),#10207,.F.);
#10634=ADVANCED_FACE('',(#509),#10208,.F.);
#10635=ADVANCED_FACE('',(#510),#10209,.F.);
#10636=ADVANCED_FACE('',(#511),#10210,.F.);
#10637=ADVANCED_FACE('',(#512),#10211,.F.);
#10638=ADVANCED_FACE('',(#513),#10212,.F.);
#10639=ADVANCED_FACE('',(#514),#10213,.F.);
#10640=ADVANCED_FACE('',(#515),#10214,.F.);
#10641=ADVANCED_FACE('',(#516),#10215,.F.);
#10642=ADVANCED_FACE('',(#517),#10216,.F.);
#10643=ADVANCED_FACE('',(#518),#10217,.F.);
#10644=ADVANCED_FACE('',(#519),#10218,.F.);
#10645=ADVANCED_FACE('',(#520),#10219,.F.);
#10646=ADVANCED_FACE('',(#521),#10220,.F.);
#10647=ADVANCED_FACE('',(#522),#10221,.F.);
#10648=ADVANCED_FACE('',(#523),#10222,.F.);
#10649=ADVANCED_FACE('',(#524),#10223,.F.);
#10650=ADVANCED_FACE('',(#525),#10224,.F.);
#10651=ADVANCED_FACE('',(#526),#10225,.F.);
#10652=ADVANCED_FACE('',(#527),#10226,.F.);
#10653=ADVANCED_FACE('',(#528),#10227,.F.);
#10654=ADVANCED_FACE('',(#529),#10228,.F.);
#10655=ADVANCED_FACE('',(#530),#10229,.F.);
#10656=ADVANCED_FACE('',(#531),#10230,.F.);
#10657=ADVANCED_FACE('',(#532),#10231,.F.);
#10658=ADVANCED_FACE('',(#533),#10232,.F.);
#10659=ADVANCED_FACE('',(#534),#10233,.F.);
#10660=ADVANCED_FACE('',(#535),#10234,.F.);
#10661=ADVANCED_FACE('',(#536),#10235,.F.);
#10662=ADVANCED_FACE('',(#537),#10236,.F.);
#10663=ADVANCED_FACE('',(#538),#10237,.F.);
#10664=ADVANCED_FACE('',(#539),#10238,.F.);
#10665=ADVANCED_FACE('',(#540),#10239,.F.);
#10666=ADVANCED_FACE('',(#541),#10240,.F.);
#10667=ADVANCED_FACE('',(#542),#10241,.F.);
#10668=ADVANCED_FACE('',(#543),#10242,.F.);
#10669=ADVANCED_FACE('',(#544),#10243,.F.);
#10670=ADVANCED_FACE('',(#545),#10244,.F.);
#10671=ADVANCED_FACE('',(#546),#10245,.F.);
#10672=ADVANCED_FACE('',(#547),#10246,.F.);
#10673=ADVANCED_FACE('',(#548),#10247,.F.);
#10674=ADVANCED_FACE('',(#549),#10248,.F.);
#10675=ADVANCED_FACE('',(#550),#10249,.F.);
#10676=ADVANCED_FACE('',(#551),#10250,.F.);
#10677=ADVANCED_FACE('',(#552),#10251,.F.);
#10678=ADVANCED_FACE('',(#553),#10252,.F.);
#10679=ADVANCED_FACE('',(#554),#10253,.F.);
#10680=ADVANCED_FACE('',(#555),#10254,.F.);
#10681=ADVANCED_FACE('',(#556),#10255,.F.);
#10682=ADVANCED_FACE('',(#557),#10256,.F.);
#10683=ADVANCED_FACE('',(#558),#10257,.F.);
#10684=ADVANCED_FACE('',(#559),#10258,.F.);
#10685=ADVANCED_FACE('',(#560),#10259,.F.);
#10686=ADVANCED_FACE('',(#561),#10260,.F.);
#10687=ADVANCED_FACE('',(#562),#10261,.F.);
#10688=ADVANCED_FACE('',(#563),#10262,.F.);
#10689=ADVANCED_FACE('',(#564),#10263,.F.);
#10690=ADVANCED_FACE('',(#565),#10264,.F.);
#10691=ADVANCED_FACE('',(#566),#10265,.F.);
#10692=ADVANCED_FACE('',(#567),#10266,.F.);
#10693=ADVANCED_FACE('',(#568),#10267,.F.);
#10694=ADVANCED_FACE('',(#569),#10268,.F.);
#10695=ADVANCED_FACE('',(#570),#10269,.F.);
#10696=ADVANCED_FACE('',(#571),#10270,.F.);
#10697=ADVANCED_FACE('',(#572),#10271,.F.);
#10698=ADVANCED_FACE('',(#573),#10272,.F.);
#10699=ADVANCED_FACE('',(#574),#10273,.F.);
#10700=ADVANCED_FACE('',(#575),#10274,.F.);
#10701=ADVANCED_FACE('',(#576),#10275,.F.);
#10702=ADVANCED_FACE('',(#577),#10276,.F.);
#10703=ADVANCED_FACE('',(#578),#10277,.F.);
#10704=ADVANCED_FACE('',(#579),#10278,.F.);
#10705=ADVANCED_FACE('',(#580),#10279,.F.);
#10706=ADVANCED_FACE('',(#581),#10280,.F.);
#10707=ADVANCED_FACE('',(#582),#10281,.F.);
#10708=ADVANCED_FACE('',(#583),#10282,.F.);
#10709=ADVANCED_FACE('',(#584),#10283,.F.);
#10710=ADVANCED_FACE('',(#585,#258),#331,.F.);
#10711=ADVANCED_FACE('',(#586),#10284,.F.);
#10712=ADVANCED_FACE('',(#587),#10285,.F.);
#10713=ADVANCED_FACE('',(#588,#259),#332,.F.);
#10714=ADVANCED_FACE('',(#589),#10286,.F.);
#10715=ADVANCED_FACE('',(#590),#10287,.F.);
#10716=ADVANCED_FACE('',(#591),#333,.T.);
#10717=ADVANCED_FACE('',(#592),#10288,.F.);
#10718=ADVANCED_FACE('',(#593),#224,.F.);
#10719=ADVANCED_FACE('',(#594),#225,.F.);
#10720=ADVANCED_FACE('',(#595),#10289,.F.);
#10721=ADVANCED_FACE('',(#596),#334,.T.);
#10722=ADVANCED_FACE('',(#597),#10290,.F.);
#10723=ADVANCED_FACE('',(#598),#226,.F.);
#10724=ADVANCED_FACE('',(#599),#227,.F.);
#10725=ADVANCED_FACE('',(#600),#10291,.F.);
#10726=ADVANCED_FACE('',(#601),#335,.T.);
#10727=ADVANCED_FACE('',(#602),#10292,.F.);
#10728=ADVANCED_FACE('',(#603),#228,.F.);
#10729=ADVANCED_FACE('',(#604),#229,.F.);
#10730=ADVANCED_FACE('',(#605),#10293,.F.);
#10731=ADVANCED_FACE('',(#606),#336,.T.);
#10732=ADVANCED_FACE('',(#607),#10294,.F.);
#10733=ADVANCED_FACE('',(#608),#230,.F.);
#10734=ADVANCED_FACE('',(#609),#231,.F.);
#10735=ADVANCED_FACE('',(#610),#10295,.F.);
#10736=ADVANCED_FACE('',(#611),#337,.F.);
#10737=ADVANCED_FACE('',(#612),#338,.F.);
#10738=ADVANCED_FACE('',(#613),#339,.F.);
#10739=ADVANCED_FACE('',(#614),#340,.F.);
#10740=ADVANCED_FACE('',(#615),#10296,.F.);
#10741=ADVANCED_FACE('',(#616),#10297,.F.);
#10742=ADVANCED_FACE('',(#617),#341,.T.);
#10743=ADVANCED_FACE('',(#618),#342,.T.);
#10744=ADVANCED_FACE('',(#619),#343,.T.);
#10745=ADVANCED_FACE('',(#620,#260),#344,.T.);
#10746=ADVANCED_FACE('',(#621),#345,.T.);
#10747=ADVANCED_FACE('',(#622),#346,.T.);
#10748=ADVANCED_FACE('',(#623),#347,.T.);
#10749=ADVANCED_FACE('',(#624,#261),#348,.T.);
#10750=ADVANCED_FACE('',(#625),#10298,.F.);
#10751=ADVANCED_FACE('',(#626),#10299,.T.);
#10752=ADVANCED_FACE('',(#627,#262),#349,.T.);
#10753=ADVANCED_FACE('',(#628,#263,#264,#265),#350,.F.);
#10754=ADVANCED_FACE('',(#629),#10300,.F.);
#10755=ADVANCED_FACE('',(#630),#351,.F.);
#10756=ADVANCED_FACE('',(#631),#10301,.F.);
#10757=ADVANCED_FACE('',(#632),#352,.F.);
#10758=ADVANCED_FACE('',(#633),#10302,.F.);
#10759=ADVANCED_FACE('',(#634),#353,.F.);
#10760=ADVANCED_FACE('',(#635,#266),#354,.F.);
#10761=ADVANCED_FACE('',(#636),#10303,.F.);
#10762=ADVANCED_FACE('',(#637),#355,.F.);
#10763=ADVANCED_FACE('',(#638),#356,.T.);
#10764=ADVANCED_FACE('',(#639),#357,.T.);
#10765=ADVANCED_FACE('',(#640,#267),#358,.T.);
#10766=ADVANCED_FACE('',(#641),#359,.T.);
#10767=ADVANCED_FACE('',(#642,#268,#269,#270,#271,#272),#360,.T.);
#10768=ADVANCED_FACE('',(#643,#273,#274,#275,#276),#361,.F.);
#11231=CLOSED_SHELL('',(#10609,#10610,#10611,#10612,#10613,#10614,#10615,
#10616,#10617,#10618,#10619,#10620,#10621,#10622,#10623,#10624,#10625,#10626,
#10627,#10628,#10629,#10630,#10631,#10632,#10633,#10634,#10635,#10636,#10637,
#10638,#10639,#10640,#10641,#10642,#10643,#10644,#10645,#10646,#10647,#10648,
#10649,#10650,#10651,#10652,#10653,#10654,#10655,#10656,#10657,#10658,#10659,
#10660,#10661,#10662,#10663,#10664,#10665,#10666,#10667,#10668,#10669,#10670,
#10671,#10672,#10673,#10674,#10675,#10676,#10677,#10678,#10679,#10680,#10681,
#10682,#10683,#10684,#10685,#10686,#10687,#10688,#10689,#10690,#10691,#10692,
#10693,#10694,#10695,#10696,#10697,#10698,#10699,#10700,#10701,#10702,#10703,
#10704,#10705,#10706,#10707,#10708,#10709,#10710,#10711,#10712,#10713,#10714,
#10715,#10716,#10717,#10718,#10719,#10720,#10721,#10722,#10723,#10724,#10725,
#10726,#10727,#10728,#10729,#10730,#10731,#10732,#10733,#10734,#10735,#10736,
#10737,#10738,#10739,#10740,#10741,#10742,#10743,#10744,#10745,#10746,#10747,
#10748,#10749,#10750,#10751,#10752,#10753,#10754,#10755,#10756,#10757,#10758,
#10759,#10760,#10761,#10762,#10763,#10764,#10765,#10766,#10767,#10768));
#11437=AXIS2_PLACEMENT_3D('',#14562,#12269,#12270);
#11438=AXIS2_PLACEMENT_3D('',#14563,#12271,#12272);
#11439=AXIS2_PLACEMENT_3D('',#14591,#12274,#12275);
#11440=AXIS2_PLACEMENT_3D('',#14602,#12277,#12278);
#11441=AXIS2_PLACEMENT_3D('',#14625,#12279,#12280);
#11442=AXIS2_PLACEMENT_3D('',#14676,#12282,#12283);
#11443=AXIS2_PLACEMENT_3D('',#14724,#12285,#12286);
#11444=AXIS2_PLACEMENT_3D('',#14772,#12288,#12289);
#11445=AXIS2_PLACEMENT_3D('',#14823,#12291,#12292);
#11446=AXIS2_PLACEMENT_3D('',#14871,#12294,#12295);
#11447=AXIS2_PLACEMENT_3D('',#14919,#12297,#12298);
#11448=AXIS2_PLACEMENT_3D('',#14970,#12300,#12301);
#11449=AXIS2_PLACEMENT_3D('',#15021,#12303,#12304);
#11450=AXIS2_PLACEMENT_3D('',#15069,#12306,#12307);
#11451=AXIS2_PLACEMENT_3D('',#15120,#12309,#12310);
#11452=AXIS2_PLACEMENT_3D('',#15139,#12312,#12313);
#11453=AXIS2_PLACEMENT_3D('',#15159,#12314,#12315);
#11454=AXIS2_PLACEMENT_3D('',#15172,#12317,#12318);
#11455=AXIS2_PLACEMENT_3D('',#15181,#12319,#12320);
#11456=AXIS2_PLACEMENT_3D('',#15205,#12322,#12323);
#11457=AXIS2_PLACEMENT_3D('',#15230,#12325,#12326);
#11458=AXIS2_PLACEMENT_3D('',#15255,#12328,#12329);
#11459=AXIS2_PLACEMENT_3D('',#15279,#12331,#12332);
#11460=AXIS2_PLACEMENT_3D('',#15304,#12334,#12335);
#11461=AXIS2_PLACEMENT_3D('',#15328,#12337,#12338);
#11462=AXIS2_PLACEMENT_3D('',#15353,#12340,#12341);
#11463=AXIS2_PLACEMENT_3D('',#15377,#12343,#12344);
#11464=AXIS2_PLACEMENT_3D('',#15402,#12346,#12347);
#11465=AXIS2_PLACEMENT_3D('',#15427,#12349,#12350);
#11466=AXIS2_PLACEMENT_3D('',#15451,#12352,#12353);
#11467=AXIS2_PLACEMENT_3D('',#15462,#12355,#12356);
#11468=AXIS2_PLACEMENT_3D('',#15468,#12357,#12358);
#11469=AXIS2_PLACEMENT_3D('',#15496,#12360,#12361);
#11470=AXIS2_PLACEMENT_3D('',#15507,#12363,#12364);
#11471=AXIS2_PLACEMENT_3D('',#15530,#12365,#12366);
#11472=AXIS2_PLACEMENT_3D('',#15581,#12368,#12369);
#11473=AXIS2_PLACEMENT_3D('',#15629,#12371,#12372);
#11474=AXIS2_PLACEMENT_3D('',#15677,#12374,#12375);
#11475=AXIS2_PLACEMENT_3D('',#15728,#12377,#12378);
#11476=AXIS2_PLACEMENT_3D('',#15776,#12380,#12381);
#11477=AXIS2_PLACEMENT_3D('',#15824,#12383,#12384);
#11478=AXIS2_PLACEMENT_3D('',#15875,#12386,#12387);
#11479=AXIS2_PLACEMENT_3D('',#15926,#12389,#12390);
#11480=AXIS2_PLACEMENT_3D('',#15974,#12392,#12393);
#11481=AXIS2_PLACEMENT_3D('',#16025,#12395,#12396);
#11482=AXIS2_PLACEMENT_3D('',#16044,#12398,#12399);
#11483=AXIS2_PLACEMENT_3D('',#16064,#12400,#12401);
#11484=AXIS2_PLACEMENT_3D('',#16077,#12403,#12404);
#11485=AXIS2_PLACEMENT_3D('',#16086,#12405,#12406);
#11486=AXIS2_PLACEMENT_3D('',#16110,#12408,#12409);
#11487=AXIS2_PLACEMENT_3D('',#16135,#12411,#12412);
#11488=AXIS2_PLACEMENT_3D('',#16160,#12414,#12415);
#11489=AXIS2_PLACEMENT_3D('',#16184,#12417,#12418);
#11490=AXIS2_PLACEMENT_3D('',#16209,#12420,#12421);
#11491=AXIS2_PLACEMENT_3D('',#16233,#12423,#12424);
#11492=AXIS2_PLACEMENT_3D('',#16258,#12426,#12427);
#11493=AXIS2_PLACEMENT_3D('',#16282,#12429,#12430);
#11494=AXIS2_PLACEMENT_3D('',#16307,#12432,#12433);
#11495=AXIS2_PLACEMENT_3D('',#16332,#12435,#12436);
#11496=AXIS2_PLACEMENT_3D('',#16356,#12438,#12439);
#11497=AXIS2_PLACEMENT_3D('',#16367,#12441,#12442);
#11498=AXIS2_PLACEMENT_3D('',#16373,#12443,#12444);
#11499=AXIS2_PLACEMENT_3D('',#16401,#12446,#12447);
#11500=AXIS2_PLACEMENT_3D('',#16412,#12449,#12450);
#11501=AXIS2_PLACEMENT_3D('',#16435,#12451,#12452);
#11502=AXIS2_PLACEMENT_3D('',#16486,#12454,#12455);
#11503=AXIS2_PLACEMENT_3D('',#16534,#12457,#12458);
#11504=AXIS2_PLACEMENT_3D('',#16582,#12460,#12461);
#11505=AXIS2_PLACEMENT_3D('',#16633,#12463,#12464);
#11506=AXIS2_PLACEMENT_3D('',#16681,#12466,#12467);
#11507=AXIS2_PLACEMENT_3D('',#16729,#12469,#12470);
#11508=AXIS2_PLACEMENT_3D('',#16780,#12472,#12473);
#11509=AXIS2_PLACEMENT_3D('',#16831,#12475,#12476);
#11510=AXIS2_PLACEMENT_3D('',#16879,#12478,#12479);
#11511=AXIS2_PLACEMENT_3D('',#16930,#12481,#12482);
#11512=AXIS2_PLACEMENT_3D('',#16949,#12484,#12485);
#11513=AXIS2_PLACEMENT_3D('',#16969,#12486,#12487);
#11514=AXIS2_PLACEMENT_3D('',#16982,#12489,#12490);
#11515=AXIS2_PLACEMENT_3D('',#16991,#12491,#12492);
#11516=AXIS2_PLACEMENT_3D('',#17015,#12494,#12495);
#11517=AXIS2_PLACEMENT_3D('',#17040,#12497,#12498);
#11518=AXIS2_PLACEMENT_3D('',#17065,#12500,#12501);
#11519=AXIS2_PLACEMENT_3D('',#17089,#12503,#12504);
#11520=AXIS2_PLACEMENT_3D('',#17114,#12506,#12507);
#11521=AXIS2_PLACEMENT_3D('',#17138,#12509,#12510);
#11522=AXIS2_PLACEMENT_3D('',#17163,#12512,#12513);
#11523=AXIS2_PLACEMENT_3D('',#17187,#12515,#12516);
#11524=AXIS2_PLACEMENT_3D('',#17212,#12518,#12519);
#11525=AXIS2_PLACEMENT_3D('',#17237,#12521,#12522);
#11526=AXIS2_PLACEMENT_3D('',#17261,#12524,#12525);
#11527=AXIS2_PLACEMENT_3D('',#17272,#12527,#12528);
#11528=AXIS2_PLACEMENT_3D('',#17278,#12529,#12530);
#11529=AXIS2_PLACEMENT_3D('',#17306,#12532,#12533);
#11530=AXIS2_PLACEMENT_3D('',#17317,#12535,#12536);
#11531=AXIS2_PLACEMENT_3D('',#17340,#12537,#12538);
#11532=AXIS2_PLACEMENT_3D('',#17391,#12540,#12541);
#11533=AXIS2_PLACEMENT_3D('',#17439,#12543,#12544);
#11534=AXIS2_PLACEMENT_3D('',#17487,#12546,#12547);
#11535=AXIS2_PLACEMENT_3D('',#17538,#12549,#12550);
#11536=AXIS2_PLACEMENT_3D('',#17586,#12552,#12553);
#11537=AXIS2_PLACEMENT_3D('',#17634,#12555,#12556);
#11538=AXIS2_PLACEMENT_3D('',#17685,#12558,#12559);
#11539=AXIS2_PLACEMENT_3D('',#17736,#12561,#12562);
#11540=AXIS2_PLACEMENT_3D('',#17784,#12564,#12565);
#11541=AXIS2_PLACEMENT_3D('',#17835,#12567,#12568);
#11542=AXIS2_PLACEMENT_3D('',#17854,#12570,#12571);
#11543=AXIS2_PLACEMENT_3D('',#17874,#12572,#12573);
#11544=AXIS2_PLACEMENT_3D('',#17887,#12575,#12576);
#11545=AXIS2_PLACEMENT_3D('',#17896,#12577,#12578);
#11546=AXIS2_PLACEMENT_3D('',#17920,#12580,#12581);
#11547=AXIS2_PLACEMENT_3D('',#17945,#12583,#12584);
#11548=AXIS2_PLACEMENT_3D('',#17970,#12586,#12587);
#11549=AXIS2_PLACEMENT_3D('',#17994,#12589,#12590);
#11550=AXIS2_PLACEMENT_3D('',#18019,#12592,#12593);
#11551=AXIS2_PLACEMENT_3D('',#18043,#12595,#12596);
#11552=AXIS2_PLACEMENT_3D('',#18068,#12598,#12599);
#11553=AXIS2_PLACEMENT_3D('',#18092,#12601,#12602);
#11554=AXIS2_PLACEMENT_3D('',#18117,#12604,#12605);
#11555=AXIS2_PLACEMENT_3D('',#18142,#12607,#12608);
#11556=AXIS2_PLACEMENT_3D('',#18166,#12610,#12611);
#11557=AXIS2_PLACEMENT_3D('',#18177,#12613,#12614);
#11558=AXIS2_PLACEMENT_3D('',#18183,#12615,#12616);
#11559=AXIS2_PLACEMENT_3D('',#18185,#12617,#12618);
#11560=AXIS2_PLACEMENT_3D('',#18188,#12620,#12621);
#11561=AXIS2_PLACEMENT_3D('',#18189,#12622,#12623);
#11562=AXIS2_PLACEMENT_3D('',#18191,#12624,#12625);
#11563=AXIS2_PLACEMENT_3D('',#18193,#12626,#12627);
#11564=AXIS2_PLACEMENT_3D('',#18194,#12628,#12629);
#11565=AXIS2_PLACEMENT_3D('',#18196,#12630,#12631);
#11566=AXIS2_PLACEMENT_3D('',#18198,#12633,#12634);
#11567=AXIS2_PLACEMENT_3D('',#18201,#12636,#12637);
#11568=AXIS2_PLACEMENT_3D('',#18202,#12638,#12639);
#11569=AXIS2_PLACEMENT_3D('',#18204,#12640,#12641);
#11570=AXIS2_PLACEMENT_3D('',#18206,#12642,#12643);
#11571=AXIS2_PLACEMENT_3D('',#18207,#12644,#12645);
#11572=AXIS2_PLACEMENT_3D('',#18209,#12646,#12647);
#11573=AXIS2_PLACEMENT_3D('',#18211,#12649,#12650);
#11574=AXIS2_PLACEMENT_3D('',#18214,#12652,#12653);
#11575=AXIS2_PLACEMENT_3D('',#18215,#12654,#12655);
#11576=AXIS2_PLACEMENT_3D('',#18326,#12656,#12657);
#11577=AXIS2_PLACEMENT_3D('',#19187,#12658,#12659);
#11578=AXIS2_PLACEMENT_3D('',#19188,#12660,#12661);
#11579=AXIS2_PLACEMENT_3D('',#19299,#12662,#12663);
#11580=AXIS2_PLACEMENT_3D('',#20160,#12664,#12665);
#11581=AXIS2_PLACEMENT_3D('',#20161,#12666,#12667);
#11582=AXIS2_PLACEMENT_3D('',#20272,#12668,#12669);
#11583=AXIS2_PLACEMENT_3D('',#21133,#12670,#12671);
#11584=AXIS2_PLACEMENT_3D('',#21134,#12672,#12673);
#11585=AXIS2_PLACEMENT_3D('',#21245,#12674,#12675);
#11586=AXIS2_PLACEMENT_3D('',#22106,#12676,#12677);
#11587=AXIS2_PLACEMENT_3D('',#22107,#12678,#12679);
#11588=AXIS2_PLACEMENT_3D('',#22108,#12680,#12681);
#11589=AXIS2_PLACEMENT_3D('',#22109,#12682,#12683);
#11590=AXIS2_PLACEMENT_3D('',#22110,#12684,#12685);
#11591=AXIS2_PLACEMENT_3D('',#22111,#12686,#12687);
#11592=AXIS2_PLACEMENT_3D('',#22113,#12688,#12689);
#11593=AXIS2_PLACEMENT_3D('',#22116,#12691,#12692);
#11594=AXIS2_PLACEMENT_3D('',#22117,#12693,#12694);
#11595=AXIS2_PLACEMENT_3D('',#22119,#12695,#12696);
#11596=AXIS2_PLACEMENT_3D('',#22122,#12698,#12699);
#11597=AXIS2_PLACEMENT_3D('',#22123,#12700,#12701);
#11598=AXIS2_PLACEMENT_3D('',#22132,#12706,#12707);
#11599=AXIS2_PLACEMENT_3D('',#22138,#12711,#12712);
#11600=AXIS2_PLACEMENT_3D('',#22144,#12716,#12717);
#11601=AXIS2_PLACEMENT_3D('',#22146,#12719,#12720);
#11602=AXIS2_PLACEMENT_3D('',#22155,#12725,#12726);
#11603=AXIS2_PLACEMENT_3D('',#22164,#12731,#12732);
#11604=AXIS2_PLACEMENT_3D('',#22167,#12735,#12736);
#11605=AXIS2_PLACEMENT_3D('',#22169,#12738,#12739);
#11606=AXIS2_PLACEMENT_3D('',#22171,#12740,#12741);
#11607=AXIS2_PLACEMENT_3D('',#22174,#12743,#12744);
#11608=AXIS2_PLACEMENT_3D('',#22175,#12745,#12746);
#11609=AXIS2_PLACEMENT_3D('',#22177,#12747,#12748);
#11610=AXIS2_PLACEMENT_3D('',#22180,#12750,#12751);
#11611=AXIS2_PLACEMENT_3D('',#22181,#12752,#12753);
#11612=AXIS2_PLACEMENT_3D('',#22182,#12754,#12755);
#11613=AXIS2_PLACEMENT_3D('',#22185,#12756,#12757);
#11614=AXIS2_PLACEMENT_3D('',#22189,#12759,#12760);
#11615=AXIS2_PLACEMENT_3D('',#22193,#12762,#12763);
#11616=AXIS2_PLACEMENT_3D('',#22197,#12765,#12766);
#11617=AXIS2_PLACEMENT_3D('',#22199,#12768,#12769);
#11618=AXIS2_PLACEMENT_3D('',#22203,#12771,#12772);
#11619=AXIS2_PLACEMENT_3D('',#22205,#12774,#12775);
#11620=AXIS2_PLACEMENT_3D('',#22209,#12778,#12779);
#11621=AXIS2_PLACEMENT_3D('',#22212,#12781,#12782);
#11622=AXIS2_PLACEMENT_3D('',#22213,#12783,#12784);
#11623=AXIS2_PLACEMENT_3D('',#22217,#12787,#12788);
#11624=AXIS2_PLACEMENT_3D('',#22221,#12790,#12791);
#11625=AXIS2_PLACEMENT_3D('',#22223,#12793,#12794);
#11626=AXIS2_PLACEMENT_3D('',#22224,#12795,#12796);
#11627=AXIS2_PLACEMENT_3D('',#22228,#12799,#12800);
#11628=AXIS2_PLACEMENT_3D('',#22229,#12801,#12802);
#11629=AXIS2_PLACEMENT_3D('',#22230,#12803,#12804);
#11630=AXIS2_PLACEMENT_3D('',#22232,#12806,#12807);
#11631=AXIS2_PLACEMENT_3D('',#22241,#12812,#12813);
#11632=AXIS2_PLACEMENT_3D('',#22248,#12818,#12819);
#11633=AXIS2_PLACEMENT_3D('',#22254,#12823,#12824);
#11634=AXIS2_PLACEMENT_3D('',#22258,#12828,#12829);
#11635=AXIS2_PLACEMENT_3D('',#22259,#12830,#12831);
#12269=DIRECTION('axis',(0.,0.,1.));
#12270=DIRECTION('refdir',(1.,0.,0.));
#12271=DIRECTION('center_axis',(0.,0.,-1.));
#12272=DIRECTION('ref_axis',(1.,0.,0.));
#12273=DIRECTION('',(0.,0.,-1.));
#12274=DIRECTION('center_axis',(0.,0.,1.));
#12275=DIRECTION('ref_axis',(1.,0.,0.));
#12276=DIRECTION('',(0.,0.,-1.));
#12277=DIRECTION('center_axis',(0.,0.,1.));
#12278=DIRECTION('ref_axis',(1.,0.,0.));
#12279=DIRECTION('center_axis',(0.,0.,-1.));
#12280=DIRECTION('ref_axis',(1.,0.,0.));
#12281=DIRECTION('',(0.,0.,-1.));
#12282=DIRECTION('center_axis',(0.,0.,-1.));
#12283=DIRECTION('ref_axis',(1.,0.,0.));
#12284=DIRECTION('',(0.,0.,-1.));
#12285=DIRECTION('center_axis',(0.,0.,-1.));
#12286=DIRECTION('ref_axis',(1.,0.,0.));
#12287=DIRECTION('',(0.,0.,-1.));
#12288=DIRECTION('center_axis',(0.,0.,-1.));
#12289=DIRECTION('ref_axis',(1.,0.,0.));
#12290=DIRECTION('',(0.,0.,-1.));
#12291=DIRECTION('center_axis',(0.,0.,-1.));
#12292=DIRECTION('ref_axis',(1.,0.,0.));
#12293=DIRECTION('',(0.,0.,-1.));
#12294=DIRECTION('center_axis',(0.,0.,-1.));
#12295=DIRECTION('ref_axis',(1.,0.,0.));
#12296=DIRECTION('',(0.,0.,-1.));
#12297=DIRECTION('center_axis',(0.,0.,-1.));
#12298=DIRECTION('ref_axis',(1.,0.,0.));
#12299=DIRECTION('',(0.,0.,-1.));
#12300=DIRECTION('center_axis',(0.,0.,-1.));
#12301=DIRECTION('ref_axis',(1.,0.,0.));
#12302=DIRECTION('',(0.,0.,-1.));
#12303=DIRECTION('center_axis',(0.,0.,-1.));
#12304=DIRECTION('ref_axis',(1.,0.,0.));
#12305=DIRECTION('',(0.,0.,-1.));
#12306=DIRECTION('center_axis',(0.,0.,-1.));
#12307=DIRECTION('ref_axis',(1.,0.,0.));
#12308=DIRECTION('',(0.,0.,-1.));
#12309=DIRECTION('center_axis',(0.,0.,-1.));
#12310=DIRECTION('ref_axis',(0.938438617144983,-0.345446033196231,0.));
#12311=DIRECTION('',(0.,0.,-1.));
#12312=DIRECTION('center_axis',(0.,0.,-1.));
#12313=DIRECTION('ref_axis',(1.,0.,0.));
#12314=DIRECTION('center_axis',(0.,0.,-1.));
#12315=DIRECTION('ref_axis',(0.450153067737633,0.892951407192126,0.));
#12316=DIRECTION('',(1.22464679914735E-16,-6.89669277429462E-30,-1.));
#12317=DIRECTION('center_axis',(0.,0.,1.));
#12318=DIRECTION('ref_axis',(1.,-5.61933055413145E-14,0.));
#12319=DIRECTION('center_axis',(0.,0.,-1.));
#12320=DIRECTION('ref_axis',(1.,-5.61933055413145E-14,0.));
#12321=DIRECTION('',(1.22464679914735E-16,-6.89669277429462E-30,-1.));
#12322=DIRECTION('center_axis',(0.,0.,-1.));
#12323=DIRECTION('ref_axis',(1.,-5.61933055413145E-14,0.));
#12324=DIRECTION('',(1.22464679914735E-16,-6.89669277429462E-30,-1.));
#12325=DIRECTION('center_axis',(0.,0.,-1.));
#12326=DIRECTION('ref_axis',(1.,-5.61933055413145E-14,0.));
#12327=DIRECTION('',(1.22464679914735E-16,-6.89669277429462E-30,-1.));
#12328=DIRECTION('center_axis',(0.,0.,-1.));
#12329=DIRECTION('ref_axis',(1.,-5.61933055413145E-14,0.));
#12330=DIRECTION('',(1.22464679914735E-16,-6.89669277429462E-30,-1.));
#12331=DIRECTION('center_axis',(0.,0.,-1.));
#12332=DIRECTION('ref_axis',(1.,-5.61933055413145E-14,0.));
#12333=DIRECTION('',(1.22464679914735E-16,-6.89669277429462E-30,-1.));
#12334=DIRECTION('center_axis',(0.,0.,-1.));
#12335=DIRECTION('ref_axis',(1.,-5.61933055413145E-14,0.));
#12336=DIRECTION('',(1.22464679914735E-16,-6.89669277429462E-30,-1.));
#12337=DIRECTION('center_axis',(0.,0.,-1.));
#12338=DIRECTION('ref_axis',(1.,-5.61933055413145E-14,0.));
#12339=DIRECTION('',(1.22464679914735E-16,-6.89669277429462E-30,-1.));
#12340=DIRECTION('center_axis',(0.,0.,-1.));
#12341=DIRECTION('ref_axis',(1.,-5.61933055413145E-14,0.));
#12342=DIRECTION('',(1.22464679914735E-16,-6.89669277429462E-30,-1.));
#12343=DIRECTION('center_axis',(0.,0.,-1.));
#12344=DIRECTION('ref_axis',(1.,-5.61933055413145E-14,0.));
#12345=DIRECTION('',(1.22464679914735E-16,-6.89669277429462E-30,-1.));
#12346=DIRECTION('center_axis',(0.,0.,-1.));
#12347=DIRECTION('ref_axis',(1.,-5.61933055413145E-14,0.));
#12348=DIRECTION('',(1.22464679914735E-16,-6.89669277429462E-30,-1.));
#12349=DIRECTION('center_axis',(0.,0.,-1.));
#12350=DIRECTION('ref_axis',(1.,-5.61933055413145E-14,0.));
#12351=DIRECTION('',(1.22464679914735E-16,-6.89669277429462E-30,-1.));
#12352=DIRECTION('center_axis',(0.,0.,-1.));
#12353=DIRECTION('ref_axis',(-0.609341520949359,-0.79290788295181,0.));
#12354=DIRECTION('',(1.22464679914735E-16,-6.89669277429462E-30,-1.));
#12355=DIRECTION('center_axis',(0.,0.,-1.));
#12356=DIRECTION('ref_axis',(1.,-5.61933055413145E-14,0.));
#12357=DIRECTION('center_axis',(0.,0.,-1.));
#12358=DIRECTION('ref_axis',(1.,0.,0.));
#12359=DIRECTION('',(0.,0.,-1.));
#12360=DIRECTION('center_axis',(0.,0.,1.));
#12361=DIRECTION('ref_axis',(1.,0.,0.));
#12362=DIRECTION('',(0.,0.,-1.));
#12363=DIRECTION('center_axis',(0.,0.,1.));
#12364=DIRECTION('ref_axis',(1.,0.,0.));
#12365=DIRECTION('center_axis',(0.,0.,-1.));
#12366=DIRECTION('ref_axis',(1.,0.,0.));
#12367=DIRECTION('',(0.,0.,-1.));
#12368=DIRECTION('center_axis',(0.,0.,-1.));
#12369=DIRECTION('ref_axis',(1.,0.,0.));
#12370=DIRECTION('',(0.,0.,-1.));
#12371=DIRECTION('center_axis',(0.,0.,-1.));
#12372=DIRECTION('ref_axis',(1.,0.,0.));
#12373=DIRECTION('',(0.,0.,-1.));
#12374=DIRECTION('center_axis',(0.,0.,-1.));
#12375=DIRECTION('ref_axis',(1.,0.,0.));
#12376=DIRECTION('',(0.,0.,-1.));
#12377=DIRECTION('center_axis',(0.,0.,-1.));
#12378=DIRECTION('ref_axis',(1.,0.,0.));
#12379=DIRECTION('',(0.,0.,-1.));
#12380=DIRECTION('center_axis',(0.,0.,-1.));
#12381=DIRECTION('ref_axis',(1.,0.,0.));
#12382=DIRECTION('',(0.,0.,-1.));
#12383=DIRECTION('center_axis',(0.,0.,-1.));
#12384=DIRECTION('ref_axis',(1.,0.,0.));
#12385=DIRECTION('',(0.,0.,-1.));
#12386=DIRECTION('center_axis',(0.,0.,-1.));
#12387=DIRECTION('ref_axis',(1.,0.,0.));
#12388=DIRECTION('',(0.,0.,-1.));
#12389=DIRECTION('center_axis',(0.,0.,-1.));
#12390=DIRECTION('ref_axis',(1.,0.,0.));
#12391=DIRECTION('',(0.,0.,-1.));
#12392=DIRECTION('center_axis',(0.,0.,-1.));
#12393=DIRECTION('ref_axis',(1.,0.,0.));
#12394=DIRECTION('',(0.,0.,-1.));
#12395=DIRECTION('center_axis',(0.,0.,-1.));
#12396=DIRECTION('ref_axis',(0.938438595705222,-0.345446091439475,0.));
#12397=DIRECTION('',(0.,0.,-1.));
#12398=DIRECTION('center_axis',(0.,0.,-1.));
#12399=DIRECTION('ref_axis',(1.,0.,0.));
#12400=DIRECTION('center_axis',(0.,0.,-1.));
#12401=DIRECTION('ref_axis',(0.450153019553355,0.892951431482697,0.));
#12402=DIRECTION('',(1.22464679914735E-16,-6.89669277429462E-30,-1.));
#12403=DIRECTION('center_axis',(0.,0.,1.));
#12404=DIRECTION('ref_axis',(1.,-5.61933055413145E-14,0.));
#12405=DIRECTION('center_axis',(0.,0.,-1.));
#12406=DIRECTION('ref_axis',(1.,-5.61933055413145E-14,0.));
#12407=DIRECTION('',(1.22464679914735E-16,-6.89669277429462E-30,-1.));
#12408=DIRECTION('center_axis',(0.,0.,-1.));
#12409=DIRECTION('ref_axis',(1.,-5.61933055413145E-14,0.));
#12410=DIRECTION('',(1.22464679914735E-16,-6.89669277429462E-30,-1.));
#12411=DIRECTION('center_axis',(0.,0.,-1.));
#12412=DIRECTION('ref_axis',(1.,-5.61933055413145E-14,0.));
#12413=DIRECTION('',(1.22464679914735E-16,-6.89669277429462E-30,-1.));
#12414=DIRECTION('center_axis',(0.,0.,-1.));
#12415=DIRECTION('ref_axis',(1.,-5.61933055413145E-14,0.));
#12416=DIRECTION('',(1.22464679914735E-16,-6.89669277429462E-30,-1.));
#12417=DIRECTION('center_axis',(0.,0.,-1.));
#12418=DIRECTION('ref_axis',(1.,-5.61933055413145E-14,0.));
#12419=DIRECTION('',(1.22464679914735E-16,-6.89669277429462E-30,-1.));
#12420=DIRECTION('center_axis',(0.,0.,-1.));
#12421=DIRECTION('ref_axis',(1.,-5.61933055413145E-14,0.));
#12422=DIRECTION('',(1.22464679914735E-16,-6.89669277429462E-30,-1.));
#12423=DIRECTION('center_axis',(0.,0.,-1.));
#12424=DIRECTION('ref_axis',(1.,-5.61933055413145E-14,0.));
#12425=DIRECTION('',(1.22464679914735E-16,-6.89669277429462E-30,-1.));
#12426=DIRECTION('center_axis',(0.,0.,-1.));
#12427=DIRECTION('ref_axis',(1.,-5.61933055413145E-14,0.));
#12428=DIRECTION('',(1.22464679914735E-16,-6.89669277429462E-30,-1.));
#12429=DIRECTION('center_axis',(0.,0.,-1.));
#12430=DIRECTION('ref_axis',(1.,-5.61933055413145E-14,0.));
#12431=DIRECTION('',(1.22464679914735E-16,-6.89669277429462E-30,-1.));
#12432=DIRECTION('center_axis',(0.,0.,-1.));
#12433=DIRECTION('ref_axis',(1.,-5.61933055413145E-14,0.));
#12434=DIRECTION('',(1.22464679914735E-16,-6.89669277429462E-30,-1.));
#12435=DIRECTION('center_axis',(0.,0.,-1.));
#12436=DIRECTION('ref_axis',(1.,-5.61933055413145E-14,0.));
#12437=DIRECTION('',(1.22464679914735E-16,-6.89669277429462E-30,-1.));
#12438=DIRECTION('center_axis',(0.,0.,-1.));
#12439=DIRECTION('ref_axis',(-0.609341511570002,-0.792907890159749,0.));
#12440=DIRECTION('',(1.22464679914735E-16,-6.89669277429462E-30,-1.));
#12441=DIRECTION('center_axis',(0.,0.,-1.));
#12442=DIRECTION('ref_axis',(1.,-5.61933055413145E-14,0.));
#12443=DIRECTION('center_axis',(0.,0.,-1.));
#12444=DIRECTION('ref_axis',(1.,0.,0.));
#12445=DIRECTION('',(0.,0.,-1.));
#12446=DIRECTION('center_axis',(0.,0.,1.));
#12447=DIRECTION('ref_axis',(1.,0.,0.));
#12448=DIRECTION('',(0.,0.,-1.));
#12449=DIRECTION('center_axis',(0.,0.,1.));
#12450=DIRECTION('ref_axis',(1.,0.,0.));
#12451=DIRECTION('center_axis',(0.,0.,-1.));
#12452=DIRECTION('ref_axis',(1.,0.,0.));
#12453=DIRECTION('',(0.,0.,-1.));
#12454=DIRECTION('center_axis',(0.,0.,-1.));
#12455=DIRECTION('ref_axis',(1.,0.,0.));
#12456=DIRECTION('',(0.,0.,-1.));
#12457=DIRECTION('center_axis',(0.,0.,-1.));
#12458=DIRECTION('ref_axis',(1.,0.,0.));
#12459=DIRECTION('',(0.,0.,-1.));
#12460=DIRECTION('center_axis',(0.,0.,-1.));
#12461=DIRECTION('ref_axis',(1.,0.,0.));
#12462=DIRECTION('',(0.,0.,-1.));
#12463=DIRECTION('center_axis',(0.,0.,-1.));
#12464=DIRECTION('ref_axis',(1.,0.,0.));
#12465=DIRECTION('',(0.,0.,-1.));
#12466=DIRECTION('center_axis',(0.,0.,-1.));
#12467=DIRECTION('ref_axis',(1.,0.,0.));
#12468=DIRECTION('',(0.,0.,-1.));
#12469=DIRECTION('center_axis',(0.,0.,-1.));
#12470=DIRECTION('ref_axis',(1.,0.,0.));
#12471=DIRECTION('',(0.,0.,-1.));
#12472=DIRECTION('center_axis',(0.,0.,-1.));
#12473=DIRECTION('ref_axis',(1.,0.,0.));
#12474=DIRECTION('',(0.,0.,-1.));
#12475=DIRECTION('center_axis',(0.,0.,-1.));
#12476=DIRECTION('ref_axis',(1.,0.,0.));
#12477=DIRECTION('',(0.,0.,-1.));
#12478=DIRECTION('center_axis',(0.,0.,-1.));
#12479=DIRECTION('ref_axis',(1.,0.,0.));
#12480=DIRECTION('',(0.,0.,-1.));
#12481=DIRECTION('center_axis',(0.,0.,-1.));
#12482=DIRECTION('ref_axis',(0.938438601292299,-0.345446076261625,0.));
#12483=DIRECTION('',(0.,0.,-1.));
#12484=DIRECTION('center_axis',(0.,0.,-1.));
#12485=DIRECTION('ref_axis',(1.,0.,0.));
#12486=DIRECTION('center_axis',(0.,0.,-1.));
#12487=DIRECTION('ref_axis',(0.450153040552508,0.892951420896642,0.));
#12488=DIRECTION('',(1.22464679914735E-16,-7.42605394171526E-30,-1.));
#12489=DIRECTION('center_axis',(0.,0.,1.));
#12490=DIRECTION('ref_axis',(1.,-6.05158675060312E-14,0.));
#12491=DIRECTION('center_axis',(0.,0.,-1.));
#12492=DIRECTION('ref_axis',(1.,-6.05158675060312E-14,0.));
#12493=DIRECTION('',(1.22464679914735E-16,-7.42605394171526E-30,-1.));
#12494=DIRECTION('center_axis',(0.,0.,-1.));
#12495=DIRECTION('ref_axis',(1.,-6.05158675060312E-14,0.));
#12496=DIRECTION('',(1.22464679914735E-16,-7.42605394171526E-30,-1.));
#12497=DIRECTION('center_axis',(0.,0.,-1.));
#12498=DIRECTION('ref_axis',(1.,-6.05158675060312E-14,0.));
#12499=DIRECTION('',(1.22464679914735E-16,-7.42605394171526E-30,-1.));
#12500=DIRECTION('center_axis',(0.,0.,-1.));
#12501=DIRECTION('ref_axis',(1.,-6.05158675060312E-14,0.));
#12502=DIRECTION('',(1.22464679914735E-16,-7.42605394171526E-30,-1.));
#12503=DIRECTION('center_axis',(0.,0.,-1.));
#12504=DIRECTION('ref_axis',(1.,-6.05158675060312E-14,0.));
#12505=DIRECTION('',(1.22464679914735E-16,-7.42605394171526E-30,-1.));
#12506=DIRECTION('center_axis',(0.,0.,-1.));
#12507=DIRECTION('ref_axis',(1.,-6.05158675060312E-14,0.));
#12508=DIRECTION('',(1.22464679914735E-16,-7.42605394171526E-30,-1.));
#12509=DIRECTION('center_axis',(0.,0.,-1.));
#12510=DIRECTION('ref_axis',(1.,-6.05158675060312E-14,0.));
#12511=DIRECTION('',(1.22464679914735E-16,-7.42605394171526E-30,-1.));
#12512=DIRECTION('center_axis',(0.,0.,-1.));
#12513=DIRECTION('ref_axis',(1.,-6.05158675060312E-14,0.));
#12514=DIRECTION('',(1.22464679914735E-16,-7.42605394171526E-30,-1.));
#12515=DIRECTION('center_axis',(0.,0.,-1.));
#12516=DIRECTION('ref_axis',(1.,-6.05158675060312E-14,0.));
#12517=DIRECTION('',(1.22464679914735E-16,-7.42605394171526E-30,-1.));
#12518=DIRECTION('center_axis',(0.,0.,-1.));
#12519=DIRECTION('ref_axis',(1.,-6.05158675060312E-14,0.));
#12520=DIRECTION('',(1.22464679914735E-16,-7.42605394171526E-30,-1.));
#12521=DIRECTION('center_axis',(0.,0.,-1.));
#12522=DIRECTION('ref_axis',(1.,-6.05158675060312E-14,0.));
#12523=DIRECTION('',(1.22464679914735E-16,-7.42605394171526E-30,-1.));
#12524=DIRECTION('center_axis',(0.,0.,-1.));
#12525=DIRECTION('ref_axis',(-0.609341503082739,-0.792907896682123,0.));
#12526=DIRECTION('',(1.22464679914735E-16,-7.42605394171526E-30,-1.));
#12527=DIRECTION('center_axis',(0.,0.,-1.));
#12528=DIRECTION('ref_axis',(1.,-6.05158675060312E-14,0.));
#12529=DIRECTION('center_axis',(0.,0.,-1.));
#12530=DIRECTION('ref_axis',(1.,0.,0.));
#12531=DIRECTION('',(0.,0.,-1.));
#12532=DIRECTION('center_axis',(0.,0.,1.));
#12533=DIRECTION('ref_axis',(1.,0.,0.));
#12534=DIRECTION('',(0.,0.,-1.));
#12535=DIRECTION('center_axis',(0.,0.,1.));
#12536=DIRECTION('ref_axis',(1.,0.,0.));
#12537=DIRECTION('center_axis',(0.,0.,-1.));
#12538=DIRECTION('ref_axis',(1.,0.,0.));
#12539=DIRECTION('',(0.,0.,-1.));
#12540=DIRECTION('center_axis',(0.,0.,-1.));
#12541=DIRECTION('ref_axis',(1.,0.,0.));
#12542=DIRECTION('',(0.,0.,-1.));
#12543=DIRECTION('center_axis',(0.,0.,-1.));
#12544=DIRECTION('ref_axis',(1.,0.,0.));
#12545=DIRECTION('',(0.,0.,-1.));
#12546=DIRECTION('center_axis',(0.,0.,-1.));
#12547=DIRECTION('ref_axis',(1.,0.,0.));
#12548=DIRECTION('',(0.,0.,-1.));
#12549=DIRECTION('center_axis',(0.,0.,-1.));
#12550=DIRECTION('ref_axis',(1.,0.,0.));
#12551=DIRECTION('',(0.,0.,-1.));
#12552=DIRECTION('center_axis',(0.,0.,-1.));
#12553=DIRECTION('ref_axis',(1.,0.,0.));
#12554=DIRECTION('',(0.,0.,-1.));
#12555=DIRECTION('center_axis',(0.,0.,-1.));
#12556=DIRECTION('ref_axis',(1.,0.,0.));
#12557=DIRECTION('',(0.,0.,-1.));
#12558=DIRECTION('center_axis',(0.,0.,-1.));
#12559=DIRECTION('ref_axis',(1.,0.,0.));
#12560=DIRECTION('',(0.,0.,-1.));
#12561=DIRECTION('center_axis',(0.,0.,-1.));
#12562=DIRECTION('ref_axis',(1.,0.,0.));
#12563=DIRECTION('',(0.,0.,-1.));
#12564=DIRECTION('center_axis',(0.,0.,-1.));
#12565=DIRECTION('ref_axis',(1.,0.,0.));
#12566=DIRECTION('',(0.,0.,-1.));
#12567=DIRECTION('center_axis',(0.,0.,-1.));
#12568=DIRECTION('ref_axis',(0.938438612980319,-0.345446044509957,0.));
#12569=DIRECTION('',(0.,0.,-1.));
#12570=DIRECTION('center_axis',(0.,0.,-1.));
#12571=DIRECTION('ref_axis',(1.,0.,0.));
#12572=DIRECTION('center_axis',(0.,0.,-1.));
#12573=DIRECTION('ref_axis',(0.450153049056661,0.892951416609544,0.));
#12574=DIRECTION('',(1.22464679914735E-16,-7.42605394171526E-30,-1.));
#12575=DIRECTION('center_axis',(0.,0.,1.));
#12576=DIRECTION('ref_axis',(1.,-6.05158675060312E-14,0.));
#12577=DIRECTION('center_axis',(0.,0.,-1.));
#12578=DIRECTION('ref_axis',(1.,-6.05158675060312E-14,0.));
#12579=DIRECTION('',(1.22464679914735E-16,-7.42605394171526E-30,-1.));
#12580=DIRECTION('center_axis',(0.,0.,-1.));
#12581=DIRECTION('ref_axis',(1.,-6.05158675060312E-14,0.));
#12582=DIRECTION('',(1.22464679914735E-16,-7.42605394171526E-30,-1.));
#12583=DIRECTION('center_axis',(0.,0.,-1.));
#12584=DIRECTION('ref_axis',(1.,-6.05158675060312E-14,0.));
#12585=DIRECTION('',(1.22464679914735E-16,-7.42605394171526E-30,-1.));
#12586=DIRECTION('center_axis',(0.,0.,-1.));
#12587=DIRECTION('ref_axis',(1.,-6.05158675060312E-14,0.));
#12588=DIRECTION('',(1.22464679914735E-16,-7.42605394171526E-30,-1.));
#12589=DIRECTION('center_axis',(0.,0.,-1.));
#12590=DIRECTION('ref_axis',(1.,-6.05158675060312E-14,0.));
#12591=DIRECTION('',(1.22464679914735E-16,-7.42605394171526E-30,-1.));
#12592=DIRECTION('center_axis',(0.,0.,-1.));
#12593=DIRECTION('ref_axis',(1.,-6.05158675060312E-14,0.));
#12594=DIRECTION('',(1.22464679914735E-16,-7.42605394171526E-30,-1.));
#12595=DIRECTION('center_axis',(0.,0.,-1.));
#12596=DIRECTION('ref_axis',(1.,-6.05158675060312E-14,0.));
#12597=DIRECTION('',(1.22464679914735E-16,-7.42605394171526E-30,-1.));
#12598=DIRECTION('center_axis',(0.,0.,-1.));
#12599=DIRECTION('ref_axis',(1.,-6.05158675060312E-14,0.));
#12600=DIRECTION('',(1.22464679914735E-16,-7.42605394171526E-30,-1.));
#12601=DIRECTION('center_axis',(0.,0.,-1.));
#12602=DIRECTION('ref_axis',(1.,-6.05158675060312E-14,0.));
#12603=DIRECTION('',(1.22464679914735E-16,-7.42605394171526E-30,-1.));
#12604=DIRECTION('center_axis',(0.,0.,-1.));
#12605=DIRECTION('ref_axis',(1.,-6.05158675060312E-14,0.));
#12606=DIRECTION('',(1.22464679914735E-16,-7.42605394171526E-30,-1.));
#12607=DIRECTION('center_axis',(0.,0.,-1.));
#12608=DIRECTION('ref_axis',(1.,-6.05158675060312E-14,0.));
#12609=DIRECTION('',(1.22464679914735E-16,-7.42605394171526E-30,-1.));
#12610=DIRECTION('center_axis',(0.,0.,-1.));
#12611=DIRECTION('ref_axis',(-0.609341531225801,-0.792907875054471,0.));
#12612=DIRECTION('',(1.22464679914735E-16,-7.42605394171526E-30,-1.));
#12613=DIRECTION('center_axis',(0.,0.,-1.));
#12614=DIRECTION('ref_axis',(1.,-6.05158675060312E-14,0.));
#12615=DIRECTION('center_axis',(0.,1.,0.));
#12616=DIRECTION('ref_axis',(0.,0.,-1.));
#12617=DIRECTION('center_axis',(0.,1.,0.));
#12618=DIRECTION('ref_axis',(0.,0.,-1.));
#12619=DIRECTION('',(0.,1.,0.));
#12620=DIRECTION('center_axis',(0.,-1.,0.));
#12621=DIRECTION('ref_axis',(0.,0.,-1.));
#12622=DIRECTION('center_axis',(0.,0.,1.));
#12623=DIRECTION('ref_axis',(-1.,0.,0.));
#12624=DIRECTION('center_axis',(0.,0.,1.));
#12625=DIRECTION('ref_axis',(-1.,0.,0.));
#12626=DIRECTION('center_axis',(0.,0.,1.));
#12627=DIRECTION('ref_axis',(-1.,0.,0.));
#12628=DIRECTION('center_axis',(0.,0.,1.));
#12629=DIRECTION('ref_axis',(-1.,0.,0.));
#12630=DIRECTION('center_axis',(0.,0.,1.));
#12631=DIRECTION('ref_axis',(-1.,0.,0.));
#12632=DIRECTION('',(0.,0.,1.));
#12633=DIRECTION('center_axis',(0.,0.,1.));
#12634=DIRECTION('ref_axis',(-1.,0.,0.));
#12635=DIRECTION('',(0.,0.,1.));
#12636=DIRECTION('center_axis',(0.,0.,-1.));
#12637=DIRECTION('ref_axis',(-1.,0.,0.));
#12638=DIRECTION('center_axis',(0.,0.,1.));
#12639=DIRECTION('ref_axis',(-1.,0.,0.));
#12640=DIRECTION('center_axis',(0.,0.,1.));
#12641=DIRECTION('ref_axis',(-1.,0.,0.));
#12642=DIRECTION('center_axis',(0.,0.,1.));
#12643=DIRECTION('ref_axis',(-1.,0.,0.));
#12644=DIRECTION('center_axis',(0.,0.,1.));
#12645=DIRECTION('ref_axis',(-1.,0.,0.));
#12646=DIRECTION('center_axis',(0.,0.,1.));
#12647=DIRECTION('ref_axis',(-1.,0.,0.));
#12648=DIRECTION('',(0.,0.,1.));
#12649=DIRECTION('center_axis',(0.,0.,1.));
#12650=DIRECTION('ref_axis',(-1.,0.,0.));
#12651=DIRECTION('',(0.,0.,1.));
#12652=DIRECTION('center_axis',(0.,0.,-1.));
#12653=DIRECTION('ref_axis',(-1.,0.,0.));
#12654=DIRECTION('center_axis',(0.,0.,1.));
#12655=DIRECTION('ref_axis',(1.,0.,0.));
#12656=DIRECTION('center_axis',(0.,0.,-1.));
#12657=DIRECTION('ref_axis',(1.,-6.05158675060312E-14,0.));
#12658=DIRECTION('center_axis',(0.,0.,-1.));
#12659=DIRECTION('ref_axis',(1.,0.,0.));
#12660=DIRECTION('center_axis',(0.,0.,1.));
#12661=DIRECTION('ref_axis',(1.,0.,0.));
#12662=DIRECTION('center_axis',(0.,0.,-1.));
#12663=DIRECTION('ref_axis',(1.,-6.05158675060312E-14,0.));
#12664=DIRECTION('center_axis',(0.,0.,-1.));
#12665=DIRECTION('ref_axis',(1.,0.,0.));
#12666=DIRECTION('center_axis',(0.,0.,1.));
#12667=DIRECTION('ref_axis',(1.,0.,0.));
#12668=DIRECTION('center_axis',(0.,0.,-1.));
#12669=DIRECTION('ref_axis',(1.,-5.61933055413145E-14,0.));
#12670=DIRECTION('center_axis',(0.,0.,-1.));
#12671=DIRECTION('ref_axis',(1.,0.,0.));
#12672=DIRECTION('center_axis',(0.,0.,1.));
#12673=DIRECTION('ref_axis',(1.,0.,0.));
#12674=DIRECTION('center_axis',(0.,0.,-1.));
#12675=DIRECTION('ref_axis',(1.,-5.61933055413145E-14,0.));
#12676=DIRECTION('center_axis',(0.,0.,-1.));
#12677=DIRECTION('ref_axis',(1.,0.,0.));
#12678=DIRECTION('center_axis',(0.,0.,-1.));
#12679=DIRECTION('ref_axis',(1.,0.,0.));
#12680=DIRECTION('center_axis',(0.,0.,-1.));
#12681=DIRECTION('ref_axis',(1.,0.,0.));
#12682=DIRECTION('center_axis',(0.,0.,-1.));
#12683=DIRECTION('ref_axis',(1.,0.,0.));
#12684=DIRECTION('center_axis',(0.,0.,-1.));
#12685=DIRECTION('ref_axis',(1.,0.,0.));
#12686=DIRECTION('center_axis',(0.,0.,-1.));
#12687=DIRECTION('ref_axis',(1.,0.,0.));
#12688=DIRECTION('center_axis',(0.,0.,-1.));
#12689=DIRECTION('ref_axis',(1.,0.,0.));
#12690=DIRECTION('',(0.,0.,-1.));
#12691=DIRECTION('center_axis',(0.,0.,1.));
#12692=DIRECTION('ref_axis',(1.,0.,0.));
#12693=DIRECTION('center_axis',(0.,0.,-1.));
#12694=DIRECTION('ref_axis',(1.,0.,0.));
#12695=DIRECTION('center_axis',(0.,0.,-1.));
#12696=DIRECTION('ref_axis',(1.,0.,0.));
#12697=DIRECTION('',(0.,0.,-1.));
#12698=DIRECTION('center_axis',(0.,0.,1.));
#12699=DIRECTION('ref_axis',(1.,0.,0.));
#12700=DIRECTION('center_axis',(0.,1.,0.));
#12701=DIRECTION('ref_axis',(-1.,0.,0.));
#12702=DIRECTION('',(-1.,0.,0.));
#12703=DIRECTION('',(0.,0.,-1.));
#12704=DIRECTION('',(-1.,0.,0.));
#12705=DIRECTION('',(0.,0.,1.));
#12706=DIRECTION('center_axis',(1.,0.,0.));
#12707=DIRECTION('ref_axis',(0.,1.,0.));
#12708=DIRECTION('',(0.,1.,0.));
#12709=DIRECTION('',(0.,1.,0.));
#12710=DIRECTION('',(0.,0.,1.));
#12711=DIRECTION('center_axis',(0.,-1.,0.));
#12712=DIRECTION('ref_axis',(1.,0.,0.));
#12713=DIRECTION('',(1.,0.,0.));
#12714=DIRECTION('',(1.,0.,0.));
#12715=DIRECTION('',(0.,0.,1.));
#12716=DIRECTION('center_axis',(0.,0.,1.));
#12717=DIRECTION('ref_axis',(1.,0.,0.));
#12718=DIRECTION('',(0.,1.,0.));
#12719=DIRECTION('center_axis',(0.,1.,0.));
#12720=DIRECTION('ref_axis',(-1.,0.,0.));
#12721=DIRECTION('',(-1.,0.,0.));
#12722=DIRECTION('',(0.,0.,1.));
#12723=DIRECTION('',(-1.,0.,0.));
#12724=DIRECTION('',(0.,0.,1.));
#12725=DIRECTION('center_axis',(0.,-1.,0.));
#12726=DIRECTION('ref_axis',(1.,0.,0.));
#12727=DIRECTION('',(1.,0.,0.));
#12728=DIRECTION('',(0.,0.,-1.));
#12729=DIRECTION('',(1.,0.,0.));
#12730=DIRECTION('',(0.,0.,1.));
#12731=DIRECTION('center_axis',(-1.,0.,0.));
#12732=DIRECTION('ref_axis',(0.,-1.,0.));
#12733=DIRECTION('',(0.,-1.,0.));
#12734=DIRECTION('',(0.,-1.,0.));
#12735=DIRECTION('center_axis',(0.,0.,1.));
#12736=DIRECTION('ref_axis',(1.,0.,0.));
#12737=DIRECTION('',(0.,-1.,0.));
#12738=DIRECTION('center_axis',(0.,0.,1.));
#12739=DIRECTION('ref_axis',(1.,0.,0.));
#12740=DIRECTION('center_axis',(0.,0.,-1.));
#12741=DIRECTION('ref_axis',(1.,0.,0.));
#12742=DIRECTION('',(0.,0.,-1.));
#12743=DIRECTION('center_axis',(0.,0.,1.));
#12744=DIRECTION('ref_axis',(1.,0.,0.));
#12745=DIRECTION('center_axis',(0.,0.,1.));
#12746=DIRECTION('ref_axis',(1.,0.,0.));
#12747=DIRECTION('center_axis',(0.,0.,1.));
#12748=DIRECTION('ref_axis',(1.,0.,0.));
#12749=DIRECTION('',(0.,0.,-1.));
#12750=DIRECTION('center_axis',(0.,0.,-1.));
#12751=DIRECTION('ref_axis',(1.,0.,0.));
#12752=DIRECTION('center_axis',(0.,0.,1.));
#12753=DIRECTION('ref_axis',(1.,0.,0.));
#12754=DIRECTION('center_axis',(0.,0.,-1.));
#12755=DIRECTION('ref_axis',(-1.,0.,0.));
#12756=DIRECTION('center_axis',(0.,0.,1.));
#12757=DIRECTION('ref_axis',(-0.707106781186547,0.707106781186547,0.));
#12758=DIRECTION('',(0.,1.,0.));
#12759=DIRECTION('center_axis',(0.,0.,1.));
#12760=DIRECTION('ref_axis',(-0.707106781186548,-0.707106781186547,0.));
#12761=DIRECTION('',(-1.,0.,0.));
#12762=DIRECTION('center_axis',(0.,0.,1.));
#12763=DIRECTION('ref_axis',(0.707106781186547,-0.707106781186547,0.));
#12764=DIRECTION('',(0.,-1.,0.));
#12765=DIRECTION('center_axis',(0.,0.,1.));
#12766=DIRECTION('ref_axis',(0.707106781186548,0.707106781186547,0.));
#12767=DIRECTION('',(1.,0.,0.));
#12768=DIRECTION('center_axis',(0.,0.,-1.));
#12769=DIRECTION('ref_axis',(-0.707106781186547,0.707106781186547,0.));
#12770=DIRECTION('',(0.,0.,1.));
#12771=DIRECTION('center_axis',(0.,0.,1.));
#12772=DIRECTION('ref_axis',(-0.707106781186547,0.707106781186547,0.));
#12773=DIRECTION('',(0.,0.,-1.));
#12774=DIRECTION('center_axis',(0.,1.,0.));
#12775=DIRECTION('ref_axis',(1.,0.,0.));
#12776=DIRECTION('',(0.,0.,-1.));
#12777=DIRECTION('',(1.,0.,0.));
#12778=DIRECTION('center_axis',(0.,0.,-1.));
#12779=DIRECTION('ref_axis',(0.707106781186548,0.707106781186547,0.));
#12780=DIRECTION('',(0.,0.,1.));
#12781=DIRECTION('center_axis',(0.,0.,1.));
#12782=DIRECTION('ref_axis',(0.707106781186548,0.707106781186547,0.));
#12783=DIRECTION('center_axis',(1.,0.,0.));
#12784=DIRECTION('ref_axis',(0.,-1.,0.));
#12785=DIRECTION('',(0.,0.,-1.));
#12786=DIRECTION('',(0.,-1.,0.));
#12787=DIRECTION('center_axis',(0.,0.,-1.));
#12788=DIRECTION('ref_axis',(-0.707106781186548,-0.707106781186547,0.));
#12789=DIRECTION('',(0.,0.,1.));
#12790=DIRECTION('center_axis',(0.,0.,1.));
#12791=DIRECTION('ref_axis',(-0.707106781186548,-0.707106781186547,0.));
#12792=DIRECTION('',(0.,0.,-1.));
#12793=DIRECTION('center_axis',(0.,0.,-1.));
#12794=DIRECTION('ref_axis',(-1.,0.,0.));
#12795=DIRECTION('center_axis',(0.,-1.,0.));
#12796=DIRECTION('ref_axis',(-1.,0.,0.));
#12797=DIRECTION('',(-1.,0.,0.));
#12798=DIRECTION('',(0.,0.,1.));
#12799=DIRECTION('center_axis',(0.,0.,-1.));
#12800=DIRECTION('ref_axis',(0.707106781186547,-0.707106781186547,0.));
#12801=DIRECTION('center_axis',(0.,0.,1.));
#12802=DIRECTION('ref_axis',(0.707106781186547,-0.707106781186547,0.));
#12803=DIRECTION('center_axis',(-1.,0.,0.));
#12804=DIRECTION('ref_axis',(0.,1.,0.));
#12805=DIRECTION('',(0.,1.,0.));
#12806=DIRECTION('center_axis',(0.,1.,0.));
#12807=DIRECTION('ref_axis',(-1.,0.,0.));
#12808=DIRECTION('',(-1.,0.,0.));
#12809=DIRECTION('',(0.,0.,1.));
#12810=DIRECTION('',(-1.,0.,0.));
#12811=DIRECTION('',(0.,0.,1.));
#12812=DIRECTION('center_axis',(1.,0.,0.));
#12813=DIRECTION('ref_axis',(0.,1.,0.));
#12814=DIRECTION('',(0.,1.,0.));
#12815=DIRECTION('',(0.,1.,0.));
#12816=DIRECTION('',(0.,0.,1.));
#12817=DIRECTION('',(0.,1.,0.));
#12818=DIRECTION('center_axis',(0.,-1.,0.));
#12819=DIRECTION('ref_axis',(1.,0.,0.));
#12820=DIRECTION('',(1.,0.,0.));
#12821=DIRECTION('',(1.,0.,0.));
#12822=DIRECTION('',(0.,0.,1.));
#12823=DIRECTION('center_axis',(-1.,0.,0.));
#12824=DIRECTION('ref_axis',(0.,-1.,0.));
#12825=DIRECTION('',(0.,-1.,0.));
#12826=DIRECTION('',(0.,-1.,0.));
#12827=DIRECTION('',(0.,-1.,0.));
#12828=DIRECTION('center_axis',(0.,0.,1.));
#12829=DIRECTION('ref_axis',(1.,0.,0.));
#12830=DIRECTION('center_axis',(0.,0.,1.));
#12831=DIRECTION('ref_axis',(1.,0.,0.));
#14562=CARTESIAN_POINT('',(0.,0.,0.));
#14563=CARTESIAN_POINT('Origin',(-3.6,-2.4,4.7));
#14564=CARTESIAN_POINT('',(-3.76675587540948,-2.40012144305632,4.38714803633902));
#14565=CARTESIAN_POINT('',(-3.76680083731002,-2.3999030629831,4.36785196366098));
#14566=CARTESIAN_POINT('',(-3.7666,-2.4,4.7));
#14567=CARTESIAN_POINT('',(-3.76351293272515,-2.4319230454628,4.3));
#14568=CARTESIAN_POINT('Ctrl Pts',(-3.76680083731002,-2.3999030629831,4.36785196366098));
#14569=CARTESIAN_POINT('Ctrl Pts',(-3.76684159509423,-2.39409443145766,
4.36746222055426));
#14570=CARTESIAN_POINT('Ctrl Pts',(-3.76656457427738,-2.38828969174785,
4.36707247744754));
#14571=CARTESIAN_POINT('Ctrl Pts',(-3.76595694000634,-2.38251974073322,
4.36668273434082));
#14572=CARTESIAN_POINT('Ctrl Pts',(-3.76018123887082,-2.32767505172373,
4.36297813798855));
#14573=CARTESIAN_POINT('Ctrl Pts',(-3.72453483587179,-2.27597349778246,
4.35927354163629));
#14574=CARTESIAN_POINT('Ctrl Pts',(-3.675321975809,-2.25108560394313,4.35556894528402));
#14575=CARTESIAN_POINT('Ctrl Pts',(-3.6261091157462,-2.22619771010379,4.35186434893175));
#14576=CARTESIAN_POINT('Ctrl Pts',(-3.56332979861965,-2.22812347636638,
4.34815975257948));
#14577=CARTESIAN_POINT('Ctrl Pts',(-3.51573443717815,-2.25596350777206,
4.34445515622722));
#14578=CARTESIAN_POINT('Ctrl Pts',(-3.46813907573665,-2.28380353917775,
4.34075055987495));
#14579=CARTESIAN_POINT('Ctrl Pts',(-3.43572766998022,-2.33755783572652,
4.33704596352268));
#14580=CARTESIAN_POINT('Ctrl Pts',(-3.43329506857802,-2.39266164758784,
4.33334136717041));
#14581=CARTESIAN_POINT('Ctrl Pts',(-3.43086246717583,-2.44776545944916,
4.32963677081814));
#14582=CARTESIAN_POINT('Ctrl Pts',(-3.45840867012789,-2.50421878662303,
4.32593217446588));
#14583=CARTESIAN_POINT('Ctrl Pts',(-3.5034058713341,-2.53611223252088,4.32222757811361));
#14584=CARTESIAN_POINT('Ctrl Pts',(-3.5484030725403,-2.56800567841873,4.31852298176134));
#14585=CARTESIAN_POINT('Ctrl Pts',(-3.61085127200066,-2.57533924304056,
4.31481838540907));
#14586=CARTESIAN_POINT('Ctrl Pts',(-3.66197494402253,-2.55491156986817,
4.3111137890568));
#14587=CARTESIAN_POINT('Ctrl Pts',(-3.7130986160444,-2.53448389669578,4.30740919270454));
#14588=CARTESIAN_POINT('Ctrl Pts',(-3.75289776062778,-2.48629498572916,
4.30370459635227));
#14589=CARTESIAN_POINT('Ctrl Pts',(-3.76351293272515,-2.4319230454628,4.3));
#14590=CARTESIAN_POINT('',(-3.60525667617797,-2.23318013248672,4.3));
#14591=CARTESIAN_POINT('Origin',(-3.6,-2.4,4.3));
#14592=CARTESIAN_POINT('',(-3.766345497777,-2.40006497186855,4.31714803633902));
#14593=CARTESIAN_POINT('Ctrl Pts',(-3.60525667255608,-2.23317994016621,
4.3));
#14594=CARTESIAN_POINT('Ctrl Pts',(-3.65930633468078,-2.23495318766097,
4.30363229181855));
#14595=CARTESIAN_POINT('Ctrl Pts',(-3.71251718041942,-2.26542183293127,
4.30726458363711));
#14596=CARTESIAN_POINT('Ctrl Pts',(-3.74128612006692,-2.31121589839408,
4.31089687545566));
#14597=CARTESIAN_POINT('Ctrl Pts',(-3.75778986656855,-2.33748637123519,
4.31298059575011));
#14598=CARTESIAN_POINT('Ctrl Pts',(-3.76624997632687,-2.36880031787527,
4.31506431604457));
#14599=CARTESIAN_POINT('Ctrl Pts',(-3.766345497777,-2.40006497186855,4.31714803633902));
#14600=CARTESIAN_POINT('',(-3.7666,-2.4,4.2));
#14601=CARTESIAN_POINT('',(-3.7666,-2.4,4.7));
#14602=CARTESIAN_POINT('Origin',(-3.6,-2.4,4.2));
#14603=CARTESIAN_POINT('Ctrl Pts',(-3.766345497777,-2.40006497186855,4.31714803633902));
#14604=CARTESIAN_POINT('Ctrl Pts',(-3.76641980162283,-2.42438499660917,
4.31876891239684));
#14605=CARTESIAN_POINT('Ctrl Pts',(-3.76143276745508,-2.44867519480749,
4.32038978845465));
#14606=CARTESIAN_POINT('Ctrl Pts',(-3.75123332790854,-2.47053847327949,
4.32201066451247));
#14607=CARTESIAN_POINT('Ctrl Pts',(-3.72792197948242,-2.52050813091336,
4.32571526086474));
#14608=CARTESIAN_POINT('Ctrl Pts',(-3.67738234157418,-2.55780017273342,
4.329419857217));
#14609=CARTESIAN_POINT('Ctrl Pts',(-3.6227496090289,-2.56532196535192,4.33312445356927));
#14610=CARTESIAN_POINT('Ctrl Pts',(-3.56811687648362,-2.57284375797042,
4.33682904992154));
#14611=CARTESIAN_POINT('Ctrl Pts',(-3.5093910493013,-2.55059530138736,4.34053364627381));
#14612=CARTESIAN_POINT('Ctrl Pts',(-3.47344562081921,-2.50877156715293,
4.34423824262608));
#14613=CARTESIAN_POINT('Ctrl Pts',(-3.43750019233712,-2.4669478329185,4.34794283897835));
#14614=CARTESIAN_POINT('Ctrl Pts',(-3.42433516255526,-2.40554882103269,
4.35164743533061));
#14615=CARTESIAN_POINT('Ctrl Pts',(-3.4399769373371,-2.35266772584057,4.35535203168288));
#14616=CARTESIAN_POINT('Ctrl Pts',(-3.45561871211893,-2.29978663064845,
4.35905662803515));
#14617=CARTESIAN_POINT('Ctrl Pts',(-3.50006729146445,-2.25542345215002,
4.36276122438742));
#14618=CARTESIAN_POINT('Ctrl Pts',(-3.55297985415763,-2.23988445249497,
4.36646582073969));
#14619=CARTESIAN_POINT('Ctrl Pts',(-3.60589241685081,-2.22434545283993,
4.37017041709195));
#14620=CARTESIAN_POINT('Ctrl Pts',(-3.66726896289165,-2.23763063202826,
4.37387501344422));
#14621=CARTESIAN_POINT('Ctrl Pts',(-3.70902050597011,-2.2736583534049,4.37757960979649));
#14622=CARTESIAN_POINT('Ctrl Pts',(-3.74496653400264,-2.3046764520682,4.38076908531067));
#14623=CARTESIAN_POINT('Ctrl Pts',(-3.76636579491573,-2.35255215149476,
4.38395856082485));
#14624=CARTESIAN_POINT('Ctrl Pts',(-3.76675587540948,-2.40012144305632,
4.38714803633902));
#14625=CARTESIAN_POINT('Origin',(-3.6,-2.4,4.7));
#14626=CARTESIAN_POINT('',(-3.76672469163696,-2.39986752250016,4.45714803633902));
#14627=CARTESIAN_POINT('',(-3.76637108132843,-2.3999167674636,4.43785196366098));
#14628=CARTESIAN_POINT('',(-3.7666,-2.4,4.7));
#14629=CARTESIAN_POINT('Ctrl Pts',(-3.76637108132843,-2.3999167674636,4.43785196366098));
#14630=CARTESIAN_POINT('Ctrl Pts',(-3.76647256500337,-2.37748041616576,
4.43635646533454));
#14631=CARTESIAN_POINT('Ctrl Pts',(-3.7622516281058,-2.3550806593951,4.43486096700809));
#14632=CARTESIAN_POINT('Ctrl Pts',(-3.7535269013147,-2.3345994559913,4.43336546868165));
#14633=CARTESIAN_POINT('Ctrl Pts',(-3.73191431207048,-2.28386413246858,
4.42966087232938));
#14634=CARTESIAN_POINT('Ctrl Pts',(-3.68266490417161,-2.24490171859149,
4.42595627597712));
#14635=CARTESIAN_POINT('Ctrl Pts',(-3.62831780053848,-2.23554372384707,
4.42225167962485));
#14636=CARTESIAN_POINT('Ctrl Pts',(-3.57397069690535,-2.22618572910265,
4.41854708327258));
#14637=CARTESIAN_POINT('Ctrl Pts',(-3.51452589753796,-2.2464321534909,4.41484248692031));
#14638=CARTESIAN_POINT('Ctrl Pts',(-3.47718894803579,-2.28701682605767,
4.41113789056804));
#14639=CARTESIAN_POINT('Ctrl Pts',(-3.43985199853362,-2.32760149862444,
4.40743329421577));
#14640=CARTESIAN_POINT('Ctrl Pts',(-3.42462289889666,-2.38852441936972,
4.40372869786351));
#14641=CARTESIAN_POINT('Ctrl Pts',(-3.4384707400222,-2.441904428893,4.40002410151124));
#14642=CARTESIAN_POINT('Ctrl Pts',(-3.45231858114774,-2.49528443841629,
4.39631950515897));
#14643=CARTESIAN_POINT('Ctrl Pts',(-3.49524336303579,-2.54112153671759,
4.3926149088067));
#14644=CARTESIAN_POINT('Ctrl Pts',(-3.54760150310682,-2.55843699301478,
4.38891031245443));
#14645=CARTESIAN_POINT('Ctrl Pts',(-3.59995964317784,-2.57575244931197,
4.38520571610217));
#14646=CARTESIAN_POINT('Ctrl Pts',(-3.66175114143183,-2.56454626360505,
4.3815011197499));
#14647=CARTESIAN_POINT('Ctrl Pts',(-3.70469439092283,-2.52994925871274,
4.37779652339763));
#14648=CARTESIAN_POINT('Ctrl Pts',(-3.74311978370889,-2.49899204150246,
4.37448167015208));
#14649=CARTESIAN_POINT('Ctrl Pts',(-3.76645418313973,-2.44930678746824,
4.37116681690653));
#14650=CARTESIAN_POINT('Ctrl Pts',(-3.76680083731002,-2.3999030629831,4.36785196366098));
#14651=CARTESIAN_POINT('Ctrl Pts',(-3.76675587540948,-2.40012144305632,
4.38714803633902));
#14652=CARTESIAN_POINT('Ctrl Pts',(-3.76681887592163,-2.40780419002449,
4.38766315717712));
#14653=CARTESIAN_POINT('Ctrl Pts',(-3.76633386603033,-2.41547894454867,
4.38817827801521));
#14654=CARTESIAN_POINT('Ctrl Pts',(-3.76527362096253,-2.42307339831024,
4.3886933988533));
#14655=CARTESIAN_POINT('Ctrl Pts',(-3.75764865276043,-2.47769045827401,
4.39239799520556));
#14656=CARTESIAN_POINT('Ctrl Pts',(-3.72027217624014,-2.52815431463659,
4.39610259155783));
#14657=CARTESIAN_POINT('Ctrl Pts',(-3.67024983212249,-2.55136949856929,
4.3998071879101));
#14658=CARTESIAN_POINT('Ctrl Pts',(-3.62022748800484,-2.57458468250198,
4.40351178426236));
#14659=CARTESIAN_POINT('Ctrl Pts',(-3.55755927628983,-2.57055119400479,
4.40721638061464));
#14660=CARTESIAN_POINT('Ctrl Pts',(-3.51092561732084,-2.54111518112976,
4.4109209769669));
#14661=CARTESIAN_POINT('Ctrl Pts',(-3.46429195835185,-2.51167916825472,
4.41462557331917));
#14662=CARTESIAN_POINT('Ctrl Pts',(-3.43369285212889,-2.45684063100183,
4.41833016967144));
#14663=CARTESIAN_POINT('Ctrl Pts',(-3.433132174149,-2.40169663743424,4.4220347660237));
#14664=CARTESIAN_POINT('Ctrl Pts',(-3.4325714961691,-2.34655264386664,4.42573936237597));
#14665=CARTESIAN_POINT('Ctrl Pts',(-3.46204924643229,-2.29110319398435,
4.42944395872824));
#14666=CARTESIAN_POINT('Ctrl Pts',(-3.50807475488023,-2.26072509261964,
4.43314855508051));
#14667=CARTESIAN_POINT('Ctrl Pts',(-3.55410026332817,-2.23034699125494,
4.43685315143278));
#14668=CARTESIAN_POINT('Ctrl Pts',(-3.61667352996086,-2.22504023840783,
4.44055774778505));
#14669=CARTESIAN_POINT('Ctrl Pts',(-3.66715754973313,-2.24723347480277,
4.44426234413731));
#14670=CARTESIAN_POINT('Ctrl Pts',(-3.71764156950539,-2.26942671119771,
4.44796694048958));
#14671=CARTESIAN_POINT('Ctrl Pts',(-3.75603634241723,-2.3191199368347,4.45167153684185));
#14672=CARTESIAN_POINT('Ctrl Pts',(-3.76477028031358,-2.37357077761011,
4.45537613319412));
#14673=CARTESIAN_POINT('Ctrl Pts',(-3.76616275698799,-2.38225203073804,
4.45596676757575));
#14674=CARTESIAN_POINT('Ctrl Pts',(-3.76680128976178,-2.39105421690488,
4.45655740195739));
#14675=CARTESIAN_POINT('Ctrl Pts',(-3.76672469163696,-2.39986752250016,
4.45714803633902));
#14676=CARTESIAN_POINT('Origin',(-3.6,-2.4,4.7));
#14677=CARTESIAN_POINT('',(-3.76633791767176,-2.39996197521538,4.52714803633902));
#14678=CARTESIAN_POINT('',(-3.76649857915956,-2.40014312937522,4.50785196366098));
#14679=CARTESIAN_POINT('',(-3.7666,-2.4,4.7));
#14680=CARTESIAN_POINT('Ctrl Pts',(-3.76649857915956,-2.40014312937522,
4.50785196366098));
#14681=CARTESIAN_POINT('Ctrl Pts',(-3.76617946285532,-2.36119271347016,
4.50525071011481));
#14682=CARTESIAN_POINT('Ctrl Pts',(-3.75254367029535,-2.32204100961925,
4.50264945656865));
#14683=CARTESIAN_POINT('Ctrl Pts',(-3.7275842614224,-2.29243603978678,4.50004820302248));
#14684=CARTESIAN_POINT('Ctrl Pts',(-3.69203811667935,-2.25027388169498,
4.49634360667021));
#14685=CARTESIAN_POINT('Ctrl Pts',(-3.63352511503972,-2.22747466102272,
4.49263901031794));
#14686=CARTESIAN_POINT('Ctrl Pts',(-3.57882406120147,-2.23447257256027,
4.48893441396567));
#14687=CARTESIAN_POINT('Ctrl Pts',(-3.52412300736323,-2.24147048409781,
4.4852298176134));
#14688=CARTESIAN_POINT('Ctrl Pts',(-3.47323390132638,-2.27826552784516,
4.48152522126114));
#14689=CARTESIAN_POINT('Ctrl Pts',(-3.44944643562249,-2.32801823904553,
4.47782062490887));
#14690=CARTESIAN_POINT('Ctrl Pts',(-3.42565896991859,-2.37777095024589,
4.4741160285566));
#14691=CARTESIAN_POINT('Ctrl Pts',(-3.42897314454765,-2.44048132889927,
4.47041143220433));
#14692=CARTESIAN_POINT('Ctrl Pts',(-3.45787219950101,-2.4874496233209,4.46670683585206));
#14693=CARTESIAN_POINT('Ctrl Pts',(-3.48677125445436,-2.53441791774253,
4.46300223949979));
#14694=CARTESIAN_POINT('Ctrl Pts',(-3.54125518973201,-2.56564412793241,
4.45929764314753));
#14695=CARTESIAN_POINT('Ctrl Pts',(-3.59638914182557,-2.56683738431542,
4.45559304679526));
#14696=CARTESIAN_POINT('Ctrl Pts',(-3.65152309391912,-2.56803064069842,
4.45188845044299));
#14697=CARTESIAN_POINT('Ctrl Pts',(-3.7073070628286,-2.53919094327454,4.44818385409072));
#14698=CARTESIAN_POINT('Ctrl Pts',(-3.73821116198855,-2.49351697797843,
4.44447925773846));
#14699=CARTESIAN_POINT('Ctrl Pts',(-3.75663967023947,-2.4662810102851,4.44227015971263));
#14700=CARTESIAN_POINT('Ctrl Pts',(-3.76622117317942,-2.43305896393576,
4.4400610616868));
#14701=CARTESIAN_POINT('Ctrl Pts',(-3.76637108132843,-2.3999167674636,4.43785196366098));
#14702=CARTESIAN_POINT('Ctrl Pts',(-3.76672469163696,-2.39986752250016,
4.45714803633902));
#14703=CARTESIAN_POINT('Ctrl Pts',(-3.76632084848944,-2.44633332149978,
4.46026199830965));
#14704=CARTESIAN_POINT('Ctrl Pts',(-3.74603891301781,-2.49310820101244,
4.46337596028029));
#14705=CARTESIAN_POINT('Ctrl Pts',(-3.71156690339415,-2.52409905358083,
4.46648992225092));
#14706=CARTESIAN_POINT('Ctrl Pts',(-3.67055648569751,-2.56096803286229,
4.47019451860319));
#14707=CARTESIAN_POINT('Ctrl Pts',(-3.60946254742337,-2.57549753551134,
4.47389911495546));
#14708=CARTESIAN_POINT('Ctrl Pts',(-3.55624507519594,-2.56103805534263,
4.47760371130773));
#14709=CARTESIAN_POINT('Ctrl Pts',(-3.5030276029685,-2.54657857517392,4.48130830765999));
#14710=CARTESIAN_POINT('Ctrl Pts',(-3.45768659678778,-2.50313011218745,
4.48501290401226));
#14711=CARTESIAN_POINT('Ctrl Pts',(-3.44097262555956,-2.45057710029542,
4.48871750036453));
#14712=CARTESIAN_POINT('Ctrl Pts',(-3.42425865433133,-2.39802408840339,
4.4924220967168));
#14713=CARTESIAN_POINT('Ctrl Pts',(-3.43617171805559,-2.33636652760581,
4.49612669306907));
#14714=CARTESIAN_POINT('Ctrl Pts',(-3.47125973540437,-2.29382235099447,
4.49983128942134));
#14715=CARTESIAN_POINT('Ctrl Pts',(-3.50634775275315,-2.25127817438312,
4.5035358857736));
#14716=CARTESIAN_POINT('Ctrl Pts',(-3.56461072372645,-2.22784738195801,
4.50724048212587));
#14717=CARTESIAN_POINT('Ctrl Pts',(-3.61938426936618,-2.23425320834927,
4.51094507847814));
#14718=CARTESIAN_POINT('Ctrl Pts',(-3.67415781500591,-2.24065903474052,
4.51464967483041));
#14719=CARTESIAN_POINT('Ctrl Pts',(-3.72544193531206,-2.27690147994813,
4.51835427118268));
#14720=CARTESIAN_POINT('Ctrl Pts',(-3.74976616178516,-2.3263939836064,4.52205886753495));
#14721=CARTESIAN_POINT('Ctrl Pts',(-3.76090458576616,-2.34905733490504,
4.52375525713631));
#14722=CARTESIAN_POINT('Ctrl Pts',(-3.76638989772718,-2.37449903782319,
4.52545164673766));
#14723=CARTESIAN_POINT('Ctrl Pts',(-3.76633791767176,-2.39996197521538,
4.52714803633902));
#14724=CARTESIAN_POINT('Origin',(-3.6,-2.4,4.7));
#14725=CARTESIAN_POINT('',(-3.7665852438883,-2.4001523433009,4.59714803633902));
#14726=CARTESIAN_POINT('',(-3.76687644757351,-2.39999932887962,4.57785196366098));
#14727=CARTESIAN_POINT('',(-3.7666,-2.4,4.7));
#14728=CARTESIAN_POINT('Ctrl Pts',(-3.76687644620932,-2.39999932888293,
4.57785196366098));
#14729=CARTESIAN_POINT('Ctrl Pts',(-3.76687974213825,-2.34481655618538,
4.57414495489509));
#14730=CARTESIAN_POINT('Ctrl Pts',(-3.73679498392134,-2.28963687265016,
4.57043794612919));
#14731=CARTESIAN_POINT('Ctrl Pts',(-3.69041339984634,-2.25973893422683,
4.5667309373633));
#14732=CARTESIAN_POINT('Ctrl Pts',(-3.64406199955899,-2.22986045251336,
4.56302634101103));
#14733=CARTESIAN_POINT('Ctrl Pts',(-3.58143498915818,-2.22523082136041,
4.55932174465877));
#14734=CARTESIAN_POINT('Ctrl Pts',(-3.53119397503756,-2.24796881775056,
4.5556171483065));
#14735=CARTESIAN_POINT('Ctrl Pts',(-3.48095296091694,-2.27070681414072,
4.55191255195423));
#14736=CARTESIAN_POINT('Ctrl Pts',(-3.44309794307651,-2.32081243807398,
4.54820795560196));
#14737=CARTESIAN_POINT('Ctrl Pts',(-3.43495348515474,-2.3753545665717,4.54450335924969));
#14738=CARTESIAN_POINT('Ctrl Pts',(-3.42680902723298,-2.42989669506942,
4.54079876289742));
#14739=CARTESIAN_POINT('Ctrl Pts',(-3.44837512922987,-2.4888753281316,4.53709416654516));
#14740=CARTESIAN_POINT('Ctrl Pts',(-3.48978194213576,-2.52529856004066,
4.53338957019289));
#14741=CARTESIAN_POINT('Ctrl Pts',(-3.53118875504166,-2.56172179194972,
4.52968497384062));
#14742=CARTESIAN_POINT('Ctrl Pts',(-3.59243627885656,-2.57558962270566,
4.52598037748835));
#14743=CARTESIAN_POINT('Ctrl Pts',(-3.64549423729516,-2.5605553606569,4.52227578113609));
#14744=CARTESIAN_POINT('Ctrl Pts',(-3.69855219573377,-2.54552109860814,
4.51857118478382));
#14745=CARTESIAN_POINT('Ctrl Pts',(-3.74342058879608,-2.50158474375469,
4.51486658843155));
#14746=CARTESIAN_POINT('Ctrl Pts',(-3.759565141404,-2.4488540185723,4.51116199207928));
#14747=CARTESIAN_POINT('Ctrl Pts',(-3.76437348603424,-2.43314918577593,
4.51005864927318));
#14748=CARTESIAN_POINT('Ctrl Pts',(-3.76663393493028,-2.41666426444364,
4.50895530646708));
#14749=CARTESIAN_POINT('Ctrl Pts',(-3.76649857915956,-2.40014312937522,
4.50785196366098));
#14750=CARTESIAN_POINT('Ctrl Pts',(-3.76633791767176,-2.39996197521538,
4.52714803633902));
#14751=CARTESIAN_POINT('Ctrl Pts',(-3.76627638304661,-2.43010531182154,
4.52915624308993));
#14752=CARTESIAN_POINT('Ctrl Pts',(-3.75845482433377,-2.46027840666142,
4.53116444984084));
#14753=CARTESIAN_POINT('Ctrl Pts',(-3.74306538783811,-2.48590718051351,
4.53317265659175));
#14754=CARTESIAN_POINT('Ctrl Pts',(-3.71467605477792,-2.53318531165342,
4.53687725294402));
#14755=CARTESIAN_POINT('Ctrl Pts',(-3.66053305601751,-2.56499901182434,
4.54058184929628));
#14756=CARTESIAN_POINT('Ctrl Pts',(-3.60541524194112,-2.56678856079501,
4.54428644564855));
#14757=CARTESIAN_POINT('Ctrl Pts',(-3.55029742786473,-2.56857810976569,
4.54799104200082));
#14758=CARTESIAN_POINT('Ctrl Pts',(-3.49420479847236,-2.54034350753613,
4.55169563835309));
#14759=CARTESIAN_POINT('Ctrl Pts',(-3.46280846367734,-2.49500647989383,
4.55540023470536));
#14760=CARTESIAN_POINT('Ctrl Pts',(-3.43141212888233,-2.44966945225154,
4.55910483105763));
#14761=CARTESIAN_POINT('Ctrl Pts',(-3.42471208868465,-2.38722999919651,
4.56280942740989));
#14762=CARTESIAN_POINT('Ctrl Pts',(-3.44577465447007,-2.33626389048712,
4.56651402376216));
#14763=CARTESIAN_POINT('Ctrl Pts',(-3.46683722025548,-2.28529778177773,
4.57021862011443));
#14764=CARTESIAN_POINT('Ctrl Pts',(-3.515662392024,-2.24580501741397,4.5739232164667));
#14765=CARTESIAN_POINT('Ctrl Pts',(-3.56990505305945,-2.23585968494016,
4.57762781281897));
#14766=CARTESIAN_POINT('Ctrl Pts',(-3.62414771409491,-2.22591435246634,
4.58133240917123));
#14767=CARTESIAN_POINT('Ctrl Pts',(-3.68380786439731,-2.24551645188247,
4.5850370055235));
#14768=CARTESIAN_POINT('Ctrl Pts',(-3.72158169788407,-2.28569497124226,
4.58874160187577));
#14769=CARTESIAN_POINT('Ctrl Pts',(-3.75015370460556,-2.31608587465984,
4.59154374669686));
#14770=CARTESIAN_POINT('Ctrl Pts',(-3.76620375900909,-2.35824929108539,
4.59434589151794));
#14771=CARTESIAN_POINT('Ctrl Pts',(-3.7665852438883,-2.4001523433009,4.59714803633902));
#14772=CARTESIAN_POINT('Origin',(-3.6,-2.4,4.7));
#14773=CARTESIAN_POINT('',(-3.76685427080137,-2.39994496470643,4.66714803633902));
#14774=CARTESIAN_POINT('',(-3.76649662121988,-2.39985729252779,4.64785196366098));
#14775=CARTESIAN_POINT('',(-3.7666,-2.4,4.7));
#14776=CARTESIAN_POINT('Ctrl Pts',(-3.76649662121988,-2.39985729252779,
4.64785196366098));
#14777=CARTESIAN_POINT('Ctrl Pts',(-3.76663205173418,-2.38326341802857,
4.64674379602763));
#14778=CARTESIAN_POINT('Ctrl Pts',(-3.76435139460867,-2.36670593234144,
4.64563562839428));
#14779=CARTESIAN_POINT('Ctrl Pts',(-3.7595015341574,-2.35093871131677,4.64452746076093));
#14780=CARTESIAN_POINT('Ctrl Pts',(-3.74328848588199,-2.29822900591163,
4.64082286440866));
#14781=CARTESIAN_POINT('Ctrl Pts',(-3.69836304774957,-2.25435098262799,
4.63711826805639));
#14782=CARTESIAN_POINT('Ctrl Pts',(-3.64528560126629,-2.23938566762668,
4.63341367170413));
#14783=CARTESIAN_POINT('Ctrl Pts',(-3.59220815478301,-2.22442035262536,
4.62970907535186));
#14784=CARTESIAN_POINT('Ctrl Pts',(-3.53097869994887,-2.23836774590636,
4.62600447899959));
#14785=CARTESIAN_POINT('Ctrl Pts',(-3.48961924396277,-2.27484474384805,
4.62229988264732));
#14786=CARTESIAN_POINT('Ctrl Pts',(-3.44825978797668,-2.31132174178974,
4.61859528629506));
#14787=CARTESIAN_POINT('Ctrl Pts',(-3.42677033083864,-2.37032834439211,
4.61489068994278));
#14788=CARTESIAN_POINT('Ctrl Pts',(-3.43498564446249,-2.42485984538296,
4.61118609359052));
#14789=CARTESIAN_POINT('Ctrl Pts',(-3.44320095808634,-2.47939134637381,
4.60748149723825));
#14790=CARTESIAN_POINT('Ctrl Pts',(-3.48112104247208,-2.52944774575313,
4.60377690088598));
#14791=CARTESIAN_POINT('Ctrl Pts',(-3.53139155597687,-2.55212044850799,
4.60007230453371));
#14792=CARTESIAN_POINT('Ctrl Pts',(-3.58166206948165,-2.57479315126284,
4.59636770818145));
#14793=CARTESIAN_POINT('Ctrl Pts',(-3.64428301210547,-2.57008215739322,
4.59266311182917));
#14794=CARTESIAN_POINT('Ctrl Pts',(-3.69059555437608,-2.54014347995252,
4.58895851547691));
#14795=CARTESIAN_POINT('Ctrl Pts',(-3.73687793816318,-2.51022429842083,
4.58525633153826));
#14796=CARTESIAN_POINT('Ctrl Pts',(-3.76687315457017,-2.45511027888938,
4.58155414759962));
#14797=CARTESIAN_POINT('Ctrl Pts',(-3.76687644620932,-2.39999932888293,
4.57785196366098));
#14798=CARTESIAN_POINT('Ctrl Pts',(-3.7665852438883,-2.4001523433009,4.59714803633902));
#14799=CARTESIAN_POINT('Ctrl Pts',(-3.76670810392422,-2.41364753218216,
4.59805048787021));
#14800=CARTESIAN_POINT('Ctrl Pts',(-3.76520580454733,-2.42711571583196,
4.59895293940139));
#14801=CARTESIAN_POINT('Ctrl Pts',(-3.76197323580484,-2.44015494667501,
4.59985539093257));
#14802=CARTESIAN_POINT('Ctrl Pts',(-3.74870342356775,-2.49368146344449,
4.60355998728484));
#14803=CARTESIAN_POINT('Ctrl Pts',(-3.70627628242244,-2.53997955767999,
4.60726458363711));
#14804=CARTESIAN_POINT('Ctrl Pts',(-3.65410883409218,-2.55786064402731,
4.61096917998938));
#14805=CARTESIAN_POINT('Ctrl Pts',(-3.60194138576191,-2.57574173037463,
4.61467377634165));
#14806=CARTESIAN_POINT('Ctrl Pts',(-3.54003363024668,-2.56520580883379,
4.61837837269391));
#14807=CARTESIAN_POINT('Ctrl Pts',(-3.49671800289895,-2.53107470364031,
4.62208296904618));
#14808=CARTESIAN_POINT('Ctrl Pts',(-3.45340237555123,-2.49694359844684,
4.62578756539845));
#14809=CARTESIAN_POINT('Ctrl Pts',(-3.42867887637101,-2.43921730960073,
4.62949216175072));
#14810=CARTESIAN_POINT('Ctrl Pts',(-3.43386235494986,-2.38431460052291,
4.63319675810299));
#14811=CARTESIAN_POINT('Ctrl Pts',(-3.43904583352872,-2.3294118914451,4.63690135445526));
#14812=CARTESIAN_POINT('Ctrl Pts',(-3.47413628986665,-2.27733276213558,
4.64060595080752));
#14813=CARTESIAN_POINT('Ctrl Pts',(-3.52307437764419,-2.25191152143151,
4.64431054715979));
#14814=CARTESIAN_POINT('Ctrl Pts',(-3.57201246542174,-2.22649028072744,
4.64801514351206));
#14815=CARTESIAN_POINT('Ctrl Pts',(-3.6347981846389,-2.22772692862883,4.65171973986433));
#14816=CARTESIAN_POINT('Ctrl Pts',(-3.68269729487669,-2.25505550621137,
4.65542433621659));
#14817=CARTESIAN_POINT('Ctrl Pts',(-3.73059640511449,-2.28238408379392,
4.65912893256886));
#14818=CARTESIAN_POINT('Ctrl Pts',(-3.76360890637291,-2.33580459105762,
4.66283352892113));
#14819=CARTESIAN_POINT('Ctrl Pts',(-3.76662644025744,-2.39086882993835,
4.6665381252734));
#14820=CARTESIAN_POINT('Ctrl Pts',(-3.76679203880333,-2.3938906876002,4.66674142896194));
#14821=CARTESIAN_POINT('Ctrl Pts',(-3.76686730212629,-2.39691749565456,
4.66694473265048));
#14822=CARTESIAN_POINT('Ctrl Pts',(-3.76685427080137,-2.39994496470643,
4.66714803633902));
#14823=CARTESIAN_POINT('Origin',(-3.6,-2.4,4.7));
#14824=CARTESIAN_POINT('',(-3.7664227625968,-2.39988235338239,4.73714803633902));
#14825=CARTESIAN_POINT('',(-3.76637219995946,-2.40008425137793,4.71785196366098));
#14826=CARTESIAN_POINT('',(-3.7666,-2.4,4.7));
#14827=CARTESIAN_POINT('Ctrl Pts',(-3.76637219995946,-2.40008425137793,
4.71785196366098));
#14828=CARTESIAN_POINT('Ctrl Pts',(-3.76622009461901,-2.36687021016323,
4.7156380408079));
#14829=CARTESIAN_POINT('Ctrl Pts',(-3.7565937463241,-2.33357496437374,4.71342411795483));
#14830=CARTESIAN_POINT('Ctrl Pts',(-3.73808953535598,-2.30630352370031,
4.71121019510175));
#14831=CARTESIAN_POINT('Ctrl Pts',(-3.70712611115225,-2.26066973862981,
4.70750559874949));
#14832=CARTESIAN_POINT('Ctrl Pts',(-3.65130474062691,-2.23190256095558,
4.70380100239722));
#14833=CARTESIAN_POINT('Ctrl Pts',(-3.5961723905296,-2.23316745266121,4.70009640604495));
#14834=CARTESIAN_POINT('Ctrl Pts',(-3.54104004043228,-2.23443234436684,
4.69639180969269));
#14835=CARTESIAN_POINT('Ctrl Pts',(-3.48659671076299,-2.26572930545233,
4.69268721334042));
#14836=CARTESIAN_POINT('Ctrl Pts',(-3.45775870005953,-2.31273510421107,
4.68898261698815));
#14837=CARTESIAN_POINT('Ctrl Pts',(-3.42892068935607,-2.35974090296982,
4.68527802063588));
#14838=CARTESIAN_POINT('Ctrl Pts',(-3.42568799761845,-2.42245553940182,
4.68157342428361));
#14839=CARTESIAN_POINT('Ctrl Pts',(-3.44954008455102,-2.47217730452778,
4.67786882793134));
#14840=CARTESIAN_POINT('Ctrl Pts',(-3.47339217148359,-2.52189906965374,
4.67416423157907));
#14841=CARTESIAN_POINT('Ctrl Pts',(-3.52432903708635,-2.55862796347366,
4.6704596352268));
#14842=CARTESIAN_POINT('Ctrl Pts',(-3.57903913598448,-2.56555479946389,
4.66675503887454));
#14843=CARTESIAN_POINT('Ctrl Pts',(-3.63374923488261,-2.57248163545412,
4.66305044252227));
#14844=CARTESIAN_POINT('Ctrl Pts',(-3.69223256707613,-2.54960641361466,
4.65934584617));
#14845=CARTESIAN_POINT('Ctrl Pts',(-3.72772390396368,-2.50739810893161,
4.65564124981774));
#14846=CARTESIAN_POINT('Ctrl Pts',(-3.75259860490409,-2.47781570803419,
4.65304482109882));
#14847=CARTESIAN_POINT('Ctrl Pts',(-3.76617930850818,-2.43873661999706,
4.6504483923799));
#14848=CARTESIAN_POINT('Ctrl Pts',(-3.76649662121988,-2.39985729252779,
4.64785196366098));
#14849=CARTESIAN_POINT('Ctrl Pts',(-3.76685427080137,-2.39994496470643,
4.66714803633902));
#14850=CARTESIAN_POINT('Ctrl Pts',(-3.76662984554536,-2.45208398518876,
4.67064932900275));
#14851=CARTESIAN_POINT('Ctrl Pts',(-3.74021751929721,-2.50441905534817,
4.67415062166648));
#14852=CARTESIAN_POINT('Ctrl Pts',(-3.6980405151982,-2.53504001717725,4.6776519143302));
#14853=CARTESIAN_POINT('Ctrl Pts',(-3.65341448974379,-2.56743899503768,
4.68135651068247));
#14854=CARTESIAN_POINT('Ctrl Pts',(-3.59113987232435,-2.57552898026078,
4.68506110703474));
#14855=CARTESIAN_POINT('Ctrl Pts',(-3.53971699472298,-2.55560754523587,
4.68876570338701));
#14856=CARTESIAN_POINT('Ctrl Pts',(-3.48829411712161,-2.53568611021095,
4.69247029973928));
#14857=CARTESIAN_POINT('Ctrl Pts',(-3.4477229793383,-2.48775325493802,4.69617489609154));
#14858=CARTESIAN_POINT('Ctrl Pts',(-3.4365711926336,-2.4337457224305,4.69987949244381));
#14859=CARTESIAN_POINT('Ctrl Pts',(-3.42541940592889,-2.37973818992299,
4.70358408879608));
#14860=CARTESIAN_POINT('Ctrl Pts',(-3.44368697030278,-2.31965598018089,
4.70728868514835));
#14861=CARTESIAN_POINT('Ctrl Pts',(-3.48301363133541,-2.28099605718198,
4.71099328150062));
#14862=CARTESIAN_POINT('Ctrl Pts',(-3.52234029236805,-2.24233613418307,
4.71469787785288));
#14863=CARTESIAN_POINT('Ctrl Pts',(-3.58272605005944,-2.22509849792735,
4.71840247420515));
#14864=CARTESIAN_POINT('Ctrl Pts',(-3.63653501999159,-2.23717205039129,
4.72210707055742));
#14865=CARTESIAN_POINT('Ctrl Pts',(-3.69034398992373,-2.24924560285524,
4.72581166690969));
#14866=CARTESIAN_POINT('Ctrl Pts',(-3.73757617209662,-2.29063034403885,
4.72951626326196));
#14867=CARTESIAN_POINT('Ctrl Pts',(-3.75661549051415,-2.342386312472,4.73322085961422));
#14868=CARTESIAN_POINT('Ctrl Pts',(-3.76334323815838,-2.36067483977454,
4.73452991852249));
#14869=CARTESIAN_POINT('Ctrl Pts',(-3.76655071734768,-2.38025835805218,
4.73583897743076));
#14870=CARTESIAN_POINT('Ctrl Pts',(-3.7664227625968,-2.39988235338239,4.73714803633902));
#14871=CARTESIAN_POINT('Origin',(-3.6,-2.4,4.7));
#14872=CARTESIAN_POINT('',(-3.76642911325459,-2.40012064491874,4.80714803633902));
#14873=CARTESIAN_POINT('',(-3.76680409091049,-2.40009747380892,4.78785196366098));
#14874=CARTESIAN_POINT('',(-3.7666,-2.4,4.7));
#14875=CARTESIAN_POINT('Ctrl Pts',(-3.76680409091049,-2.40009747380892,
4.78785196366098));
#14876=CARTESIAN_POINT('Ctrl Pts',(-3.76646019447366,-2.35062358790434,
4.78453228558818));
#14877=CARTESIAN_POINT('Ctrl Pts',(-3.74304697023447,-2.30086701998663,
4.78121260751538));
#14878=CARTESIAN_POINT('Ctrl Pts',(-3.70452480595454,-2.26991420375009,
4.77789292944258));
#14879=CARTESIAN_POINT('Ctrl Pts',(-3.66153597807928,-2.23537239348787,
4.77418833309031));
#14880=CARTESIAN_POINT('Ctrl Pts',(-3.59973129997326,-2.22424775044289,
4.77048373673805));
#14881=CARTESIAN_POINT('Ctrl Pts',(-3.54739603302806,-2.24163153058572,
4.76677914038578));
#14882=CARTESIAN_POINT('Ctrl Pts',(-3.49506076608285,-2.25901531072854,
4.76307454403351));
#14883=CARTESIAN_POINT('Ctrl Pts',(-3.45219491029846,-2.30490751405916,
4.75936994768124));
#14884=CARTESIAN_POINT('Ctrl Pts',(-3.43841626764055,-2.35830531349683,
4.75566535132897));
#14885=CARTESIAN_POINT('Ctrl Pts',(-3.42463762498264,-2.4117031129345,4.7519607549767));
#14886=CARTESIAN_POINT('Ctrl Pts',(-3.4399461954512,-2.47260650847922,4.74825615862444));
#14887=CARTESIAN_POINT('Ctrl Pts',(-3.47733592496581,-2.51314271581421,
4.74455156227217));
#14888=CARTESIAN_POINT('Ctrl Pts',(-3.51472565448041,-2.55367892314919,
4.7408469659199));
#14889=CARTESIAN_POINT('Ctrl Pts',(-3.57419654304106,-2.57384794227444,
4.73714236956763));
#14890=CARTESIAN_POINT('Ctrl Pts',(-3.62853140127509,-2.56441930722117,
4.73343777321536));
#14891=CARTESIAN_POINT('Ctrl Pts',(-3.68286625950912,-2.55499067216789,
4.7297331768631));
#14892=CARTESIAN_POINT('Ctrl Pts',(-3.73206508741654,-2.5159643829361,4.72602858051083));
#14893=CARTESIAN_POINT('Ctrl Pts',(-3.75361176242918,-2.46520104208683,
4.72232398415856));
#14894=CARTESIAN_POINT('Ctrl Pts',(-3.7622818183227,-2.4447746420856,4.72083331065936));
#14895=CARTESIAN_POINT('Ctrl Pts',(-3.76647461518129,-2.42244785405319,
4.71934263716017));
#14896=CARTESIAN_POINT('Ctrl Pts',(-3.76637219995946,-2.40008425137793,
4.71785196366098));
#14897=CARTESIAN_POINT('Ctrl Pts',(-3.7664227625968,-2.39988235338239,4.73714803633902));
#14898=CARTESIAN_POINT('Ctrl Pts',(-3.76618860934753,-2.43579365983134,
4.73954357378302));
#14899=CARTESIAN_POINT('Ctrl Pts',(-3.75478479773435,-2.47184051531438,
4.74193911122703));
#14900=CARTESIAN_POINT('Ctrl Pts',(-3.73334402642865,-2.50033503613074,
4.74433464867103));
#14901=CARTESIAN_POINT('Ctrl Pts',(-3.70018678926345,-2.54440059567364,
4.7480392450233));
#14902=CARTESIAN_POINT('Ctrl Pts',(-3.64302586027087,-2.57040451907673,
4.75174384137556));
#14903=CARTESIAN_POINT('Ctrl Pts',(-3.58802126272889,-2.56644596334232,
4.75544843772783));
#14904=CARTESIAN_POINT('Ctrl Pts',(-3.53301666518691,-2.56248740760791,
4.7591530340801));
#14905=CARTESIAN_POINT('Ctrl Pts',(-3.48016839909552,-2.52856637273599,
4.76285763043237));
#14906=CARTESIAN_POINT('Ctrl Pts',(-3.4536627731015,-2.48020701268106,4.76656222678464));
#14907=CARTESIAN_POINT('Ctrl Pts',(-3.42715714710748,-2.43184765262612,
4.77026682313691));
#14908=CARTESIAN_POINT('Ctrl Pts',(-3.42699416121083,-2.36904996738817,
4.77397141948918));
#14909=CARTESIAN_POINT('Ctrl Pts',(-3.45324840683133,-2.32055367370344,
4.77767601584144));
#14910=CARTESIAN_POINT('Ctrl Pts',(-3.47950265245184,-2.2720573800187,4.78138061219371));
#14911=CARTESIAN_POINT('Ctrl Pts',(-3.53217412958951,-2.23786247788719,
4.78508520854597));
#14912=CARTESIAN_POINT('Ctrl Pts',(-3.58715743806471,-2.23361845816768,
4.78878980489824));
#14913=CARTESIAN_POINT('Ctrl Pts',(-3.6421407465399,-2.22937443844816,4.79249440125051));
#14914=CARTESIAN_POINT('Ctrl Pts',(-3.69943588635261,-2.25508130114064,
4.79619899760278));
#14915=CARTESIAN_POINT('Ctrl Pts',(-3.73282141188201,-2.29897415476607,
4.79990359395505));
#14916=CARTESIAN_POINT('Ctrl Pts',(-3.75458352333835,-2.32758539144982,
4.80231840808304));
#14917=CARTESIAN_POINT('Ctrl Pts',(-3.76618646552292,-2.36392383602884,
4.80473322221103));
#14918=CARTESIAN_POINT('Ctrl Pts',(-3.76642911325459,-2.40012064491874,
4.80714803633902));
#14919=CARTESIAN_POINT('Origin',(-3.6,-2.4,4.7));
#14920=CARTESIAN_POINT('',(-3.76685810224694,-2.40005005741615,4.87714803633902));
#14921=CARTESIAN_POINT('',(-3.76666750911963,-2.3998541249347,4.85785196366098));
#14922=CARTESIAN_POINT('',(-3.7666,-2.4,4.7));
#14923=CARTESIAN_POINT('Ctrl Pts',(-3.76666750911963,-2.3998541249347,4.85785196366098));
#14924=CARTESIAN_POINT('Ctrl Pts',(-3.76676617376365,-2.38908842257499,
4.85713112672072));
#14925=CARTESIAN_POINT('Ctrl Pts',(-3.76581236816026,-2.37834012863908,
4.85641028978047));
#14926=CARTESIAN_POINT('Ctrl Pts',(-3.76374257749965,-2.36781121686714,
4.85568945284021));
#14927=CARTESIAN_POINT('Ctrl Pts',(-3.75310530504175,-2.31369999425172,
4.85198485648794));
#14928=CARTESIAN_POINT('Ctrl Pts',(-3.71299219872321,-2.26538317916478,
4.84828026013567));
#14929=CARTESIAN_POINT('Ctrl Pts',(-3.66176124910748,-2.24497323600586,
4.8445756637834));
#14930=CARTESIAN_POINT('Ctrl Pts',(-3.61053029949175,-2.22456329284695,
4.84087106743114));
#14931=CARTESIAN_POINT('Ctrl Pts',(-3.54818150657882,-2.23206022161606,
4.83716647107887));
#14932=CARTESIAN_POINT('Ctrl Pts',(-3.50324914898701,-2.26403301035152,
4.8334618747266));
#14933=CARTESIAN_POINT('Ctrl Pts',(-3.45831679139521,-2.29600579908698,
4.82975727837433));
#14934=CARTESIAN_POINT('Ctrl Pts',(-3.43080086912452,-2.35245444778878,
4.82605268202206));
#14935=CARTESIAN_POINT('Ctrl Pts',(-3.43329420002801,-2.40754491229296,
4.82234808566979));
#14936=CARTESIAN_POINT('Ctrl Pts',(-3.43578753093151,-2.46263537679713,
4.81864348931753));
#14937=CARTESIAN_POINT('Ctrl Pts',(-3.4682901150092,-2.51636765710367,4.81493889296526));
#14938=CARTESIAN_POINT('Ctrl Pts',(-3.51592696035573,-2.54415087044753,
4.81123429661299));
#14939=CARTESIAN_POINT('Ctrl Pts',(-3.56356380570226,-2.5719340837914,4.80752970026073));
#14940=CARTESIAN_POINT('Ctrl Pts',(-3.62633491231765,-2.57376823017258,
4.80382510390846));
#14941=CARTESIAN_POINT('Ctrl Pts',(-3.67551272732296,-2.54881390209942,
4.80012050755619));
#14942=CARTESIAN_POINT('Ctrl Pts',(-3.72469054232828,-2.52385957402626,
4.79641591120392));
#14943=CARTESIAN_POINT('Ctrl Pts',(-3.76027506572354,-2.47211677149876,
4.79271131485165));
#14944=CARTESIAN_POINT('Ctrl Pts',(-3.76598083859892,-2.41726588149528,
4.78900671849938));
#14945=CARTESIAN_POINT('Ctrl Pts',(-3.76657368490912,-2.41156671532445,
4.78862180021991));
#14946=CARTESIAN_POINT('Ctrl Pts',(-3.7668439658688,-2.40583399482793,4.78823688194045));
#14947=CARTESIAN_POINT('Ctrl Pts',(-3.76680409091049,-2.40009747380892,
4.78785196366098));
#14948=CARTESIAN_POINT('Ctrl Pts',(-3.76642911325459,-2.40012064491874,
4.80714803633902));
#14949=CARTESIAN_POINT('Ctrl Pts',(-3.76655871442242,-2.41945381020902,
4.8084378185633));
#14950=CARTESIAN_POINT('Ctrl Pts',(-3.76344749532011,-2.43874657022512,
4.80972760078758));
#14951=CARTESIAN_POINT('Ctrl Pts',(-3.75691244110645,-2.45679995321808,
4.81101738301185));
#14952=CARTESIAN_POINT('Ctrl Pts',(-3.73814203355539,-2.50865405348629,
4.81472197936412));
#14953=CARTESIAN_POINT('Ctrl Pts',(-3.69112530720718,-2.55028340946432,
4.81842657571639));
#14954=CARTESIAN_POINT('Ctrl Pts',(-3.63737973347804,-2.56263611033431,
4.82213117206866));
#14955=CARTESIAN_POINT('Ctrl Pts',(-3.58363415974891,-2.5749888112043,4.82583576842093));
#14956=CARTESIAN_POINT('Ctrl Pts',(-3.52315973863885,-2.55806485696625,
4.82954036477319));
#14957=CARTESIAN_POINT('Ctrl Pts',(-3.48363293188217,-2.51960959124259,
4.83324496112546));
#14958=CARTESIAN_POINT('Ctrl Pts',(-3.44410612512549,-2.48115432551893,
4.83694955747773));
#14959=CARTESIAN_POINT('Ctrl Pts',(-3.42552693272221,-2.42116774830966,
4.84065415383));
#14960=CARTESIAN_POINT('Ctrl Pts',(-3.43639822742686,-2.36710305682155,
4.84435875018227));
#14961=CARTESIAN_POINT('Ctrl Pts',(-3.44726952213151,-2.31303836533343,
4.84806334653454));
#14962=CARTESIAN_POINT('Ctrl Pts',(-3.48759130394411,-2.26489555956646,
4.8517679428868));
#14963=CARTESIAN_POINT('Ctrl Pts',(-3.53891008077804,-2.24470746756836,
4.85547253923907));
#14964=CARTESIAN_POINT('Ctrl Pts',(-3.59022885761198,-2.22451937557026,
4.85917713559134));
#14965=CARTESIAN_POINT('Ctrl Pts',(-3.65254462946725,-2.23228599734102,
4.86288173194361));
#14966=CARTESIAN_POINT('Ctrl Pts',(-3.69733822999987,-2.26445289438714,
4.86658632829587));
#14967=CARTESIAN_POINT('Ctrl Pts',(-3.73990669414912,-2.29502189057005,
4.87010689764359));
#14968=CARTESIAN_POINT('Ctrl Pts',(-3.76665058750282,-2.34762719015485,
4.87362746699131));
#14969=CARTESIAN_POINT('Ctrl Pts',(-3.76685810224694,-2.40005005741615,
4.87714803633902));
#14970=CARTESIAN_POINT('Origin',(-3.6,-2.4,4.7));
#14971=CARTESIAN_POINT('',(-3.76657660157387,-2.39984780956506,4.94714803633902));
#14972=CARTESIAN_POINT('',(-3.76633014204238,-2.3999936674641,4.92785196366098));
#14973=CARTESIAN_POINT('',(-3.7666,-2.4,4.7));
#14974=CARTESIAN_POINT('Ctrl Pts',(-3.76633014204238,-2.3999936674641,4.92785196366098));
#14975=CARTESIAN_POINT('Ctrl Pts',(-3.76633943871615,-2.37257318075516,
4.926025371501));
#14976=CARTESIAN_POINT('Ctrl Pts',(-3.75993532676097,-2.34515678209823,
4.92419877934102));
#14977=CARTESIAN_POINT('Ctrl Pts',(-3.74709395990921,-2.32118936363805,
4.92237218718104));
#14978=CARTESIAN_POINT('Ctrl Pts',(-3.72104978768541,-2.27257992966252,
4.91866759082877));
#14979=CARTESIAN_POINT('Ctrl Pts',(-3.66852675339565,-2.23815745462599,
4.9149629944765));
#14980=CARTESIAN_POINT('Ctrl Pts',(-3.61356232150655,-2.23367557941999,
4.91125839812423));
#14981=CARTESIAN_POINT('Ctrl Pts',(-3.55859788961746,-2.22919370421399,
4.90755380177196));
#14982=CARTESIAN_POINT('Ctrl Pts',(-3.50119206012902,-2.25465242883852,
4.90384920541969));
#14983=CARTESIAN_POINT('Ctrl Pts',(-3.4676169364208,-2.2984004236072,4.90014460906743));
#14984=CARTESIAN_POINT('Ctrl Pts',(-3.43404181271257,-2.34214841837589,
4.89644001271516));
#14985=CARTESIAN_POINT('Ctrl Pts',(-3.42429739478456,-2.40418568328873,
4.89273541636289));
#14986=CARTESIAN_POINT('Ctrl Pts',(-3.44284327075563,-2.45612051228373,
4.88903082001062));
#14987=CARTESIAN_POINT('Ctrl Pts',(-3.46138914672669,-2.50805534127872,
4.88532622365836));
#14988=CARTESIAN_POINT('Ctrl Pts',(-3.50822531659685,-2.54988773435588,
4.88162162730609));
#14989=CARTESIAN_POINT('Ctrl Pts',(-3.56191694164611,-2.56247285961735,
4.87791703095382));
#14990=CARTESIAN_POINT('Ctrl Pts',(-3.61560856669538,-2.57505798487881,
4.87421243460155));
#14991=CARTESIAN_POINT('Ctrl Pts',(-3.67615564692375,-2.55839584232458,
4.87050783824928));
#14992=CARTESIAN_POINT('Ctrl Pts',(-3.7158484677393,-2.52011195597552,4.86680324189701));
#14993=CARTESIAN_POINT('Ctrl Pts',(-3.74781789610229,-2.48927731291044,
4.863819482485));
#14994=CARTESIAN_POINT('Ctrl Pts',(-3.76625910668661,-2.44441658275108,
4.86083572307299));
#14995=CARTESIAN_POINT('Ctrl Pts',(-3.76666750911963,-2.3998541249347,4.85785196366098));
#14996=CARTESIAN_POINT('Ctrl Pts',(-3.76685810224694,-2.40005005741615,
4.87714803633902));
#14997=CARTESIAN_POINT('Ctrl Pts',(-3.76686894944607,-2.40279030260928,
4.87733206334357));
#14998=CARTESIAN_POINT('Ctrl Pts',(-3.76680728980785,-2.40553004933232,
4.87751609034813));
#14999=CARTESIAN_POINT('Ctrl Pts',(-3.76667159341225,-2.40826612418172,
4.87770011735268));
#15000=CARTESIAN_POINT('Ctrl Pts',(-3.76393992708203,-2.46334528460871,
4.88140471370495));
#15001=CARTESIAN_POINT('Ctrl Pts',(-3.73120516521163,-2.5169364331412,4.88510931005721));
#15002=CARTESIAN_POINT('Ctrl Pts',(-3.6834485571899,-2.54451327676931,4.88881390640948));
#15003=CARTESIAN_POINT('Ctrl Pts',(-3.63569194916816,-2.57209012039741,
4.89251850276175));
#15004=CARTESIAN_POINT('Ctrl Pts',(-3.57291349499508,-2.57365265912114,
4.89622309911402));
#15005=CARTESIAN_POINT('Ctrl Pts',(-3.52384411020076,-2.5484857882364,4.89992769546629));
#15006=CARTESIAN_POINT('Ctrl Pts',(-3.47477472540644,-2.52331891735167,
4.90363229181856));
#15007=CARTESIAN_POINT('Ctrl Pts',(-3.43941440999087,-2.47142263685848,
4.90733688817082));
#15008=CARTESIAN_POINT('Ctrl Pts',(-3.43394601281114,-2.41654757379038,
4.91104148452309));
#15009=CARTESIAN_POINT('Ctrl Pts',(-3.42847761563141,-2.36167251072229,
4.91474608087536));
#15010=CARTESIAN_POINT('Ctrl Pts',(-3.45290113668751,-2.30381866507929,
4.91845067722763));
#15011=CARTESIAN_POINT('Ctrl Pts',(-3.4960390130763,-2.2694631773857,4.9221552735799));
#15012=CARTESIAN_POINT('Ctrl Pts',(-3.53917688946509,-2.23510768969211,
4.92585986993217));
#15013=CARTESIAN_POINT('Ctrl Pts',(-3.60102912118658,-2.22425055994793,
4.92956446628443));
#15014=CARTESIAN_POINT('Ctrl Pts',(-3.65328868366947,-2.24186061512031,
4.9332690626367));
#15015=CARTESIAN_POINT('Ctrl Pts',(-3.70554824615237,-2.25947067029269,
4.93697365898897));
#15016=CARTESIAN_POINT('Ctrl Pts',(-3.74821513939667,-2.30554791038164,
4.94067825534123));
#15017=CARTESIAN_POINT('Ctrl Pts',(-3.76176261776726,-2.35900482523354,
4.9443828516935));
#15018=CARTESIAN_POINT('Ctrl Pts',(-3.76513332050279,-2.37230526124053,
4.94530457990868));
#15019=CARTESIAN_POINT('Ctrl Pts',(-3.76670139313906,-2.38606253416914,
4.94622630812385));
#15020=CARTESIAN_POINT('Ctrl Pts',(-3.76657660157387,-2.39984780956506,
4.94714803633902));
#15021=CARTESIAN_POINT('Origin',(-3.6,-2.4,4.7));
#15022=CARTESIAN_POINT('',(-3.76634000649331,-2.40004261214866,5.01714803633902));
#15023=CARTESIAN_POINT('',(-3.76664426409402,-2.40014916296054,4.99785196366098));
#15024=CARTESIAN_POINT('',(-3.7666,-2.4,4.7));
#15025=CARTESIAN_POINT('Ctrl Pts',(-3.76664426409402,-2.40014916296054,
4.99785196366098));
#15026=CARTESIAN_POINT('Ctrl Pts',(-3.76623994861442,-2.35633882629306,
4.99491961628127));
#15027=CARTESIAN_POINT('Ctrl Pts',(-3.74849621908403,-2.31223872253049,
4.99198726890157));
#15028=CARTESIAN_POINT('Ctrl Pts',(-3.71750016680111,-2.28150333241251,
4.98905492152186));
#15029=CARTESIAN_POINT('Ctrl Pts',(-3.678341142527,-2.24267361704367,4.98535032516959));
#15030=CARTESIAN_POINT('Ctrl Pts',(-3.61803053121903,-2.22517487203488,
4.98164572881732));
#15031=CARTESIAN_POINT('Ctrl Pts',(-3.56416982600182,-2.23701549741557,
4.97794113246506));
#15032=CARTESIAN_POINT('Ctrl Pts',(-3.51030912078461,-2.24885612279626,
4.97423653611279));
#15033=CARTESIAN_POINT('Ctrl Pts',(-3.46289832165815,-2.29003611856643,
4.97053193976052));
#15034=CARTESIAN_POINT('Ctrl Pts',(-3.44363524974256,-2.34170922607974,
4.96682734340825));
#15035=CARTESIAN_POINT('Ctrl Pts',(-3.42437217782697,-2.39338233359304,
4.96312274705598));
#15036=CARTESIAN_POINT('Ctrl Pts',(-3.43325683312225,-2.45554855284948,
4.95941815070371));
#15037=CARTESIAN_POINT('Ctrl Pts',(-3.46622310272193,-2.4997571611377,4.95571355435145));
#15038=CARTESIAN_POINT('Ctrl Pts',(-3.49918937232162,-2.54396576942592,
4.95200895799918));
#15039=CARTESIAN_POINT('Ctrl Pts',(-3.55623725622572,-2.57021676674591,
4.94830436164691));
#15040=CARTESIAN_POINT('Ctrl Pts',(-3.61125846689758,-2.56649623530203,
4.94459976529464));
#15041=CARTESIAN_POINT('Ctrl Pts',(-3.66627967756944,-2.56277570385816,
4.94089516894238));
#15042=CARTESIAN_POINT('Ctrl Pts',(-3.71927421500904,-2.52908364365041,
4.93719057259011));
#15043=CARTESIAN_POINT('Ctrl Pts',(-3.74598882864993,-2.48083941708926,
4.93348597623784));
#15044=CARTESIAN_POINT('Ctrl Pts',(-3.7595315068913,-2.45638253943781,4.93160797204555));
#15045=CARTESIAN_POINT('Ctrl Pts',(-3.76632058370052,-2.4281859427416,4.92972996785327));
#15046=CARTESIAN_POINT('Ctrl Pts',(-3.76633014204238,-2.3999936674641,4.92785196366098));
#15047=CARTESIAN_POINT('Ctrl Pts',(-3.76657660157387,-2.39984780956506,
4.94714803633902));
#15048=CARTESIAN_POINT('Ctrl Pts',(-3.76619983273375,-2.44146810829183,
4.94993090447612));
#15049=CARTESIAN_POINT('Ctrl Pts',(-3.75039179589374,-2.48334366291991,
4.95271377261321));
#15050=CARTESIAN_POINT('Ctrl Pts',(-3.7221733933057,-2.5136723837762,4.95549664075031));
#15051=CARTESIAN_POINT('Ctrl Pts',(-3.68460862697666,-2.55404643785209,
4.95920123710258));
#15052=CARTESIAN_POINT('Ctrl Pts',(-3.62505103082171,-2.57395795638902,
4.96290583345484));
#15053=CARTESIAN_POINT('Ctrl Pts',(-3.57075747641916,-2.56429432021831,
4.96661042980711));
#15054=CARTESIAN_POINT('Ctrl Pts',(-3.51646392201662,-2.5546306840476,4.97031502615938));
#15055=CARTESIAN_POINT('Ctrl Pts',(-3.46743440936648,-2.51539189316926,
4.97401962251165));
#15056=CARTESIAN_POINT('Ctrl Pts',(-3.44610757298242,-2.46453580233588,
4.97772421886392));
#15057=CARTESIAN_POINT('Ctrl Pts',(-3.42478073659837,-2.41367971150249,
4.98142881521618));
#15058=CARTESIAN_POINT('Ctrl Pts',(-3.43115657648041,-2.35120632071406,
4.98513341156845));
#15059=CARTESIAN_POINT('Ctrl Pts',(-3.46231715328677,-2.30570693229799,
4.98883800792072));
#15060=CARTESIAN_POINT('Ctrl Pts',(-3.49347773009313,-2.26020754388192,
4.99254260427299));
#15061=CARTESIAN_POINT('Ctrl Pts',(-3.54942304382382,-2.2316821578382,4.99624720062526));
#15062=CARTESIAN_POINT('Ctrl Pts',(-3.60454940455119,-2.2331855772681,4.99995179697753));
#15063=CARTESIAN_POINT('Ctrl Pts',(-3.65967576527857,-2.23468899669801,
5.00365639332979));
#15064=CARTESIAN_POINT('Ctrl Pts',(-3.71398317300263,-2.26622122160152,
5.00736098968206));
#15065=CARTESIAN_POINT('Ctrl Pts',(-3.74261753436876,-2.31335135359861,
5.01106558603433));
#15066=CARTESIAN_POINT('Ctrl Pts',(-3.75828879455967,-2.33914513862194,
5.01309306946923));
#15067=CARTESIAN_POINT('Ctrl Pts',(-3.76627033973982,-2.36961088421597,
5.01512055290412));
#15068=CARTESIAN_POINT('Ctrl Pts',(-3.76634000649331,-2.40004261214866,
5.01714803633902));
#15069=CARTESIAN_POINT('Origin',(-3.6,-2.4,4.7));
#15070=CARTESIAN_POINT('',(-3.76673281282141,-2.40013003219325,5.08714803633902));
#15071=CARTESIAN_POINT('',(-3.7668206250807,-2.39991359866148,5.06785196366098));
#15072=CARTESIAN_POINT('',(-3.7666,-2.4,4.7));
#15073=CARTESIAN_POINT('Ctrl Pts',(-3.7668206250807,-2.39991359866148,5.06785196366098));
#15074=CARTESIAN_POINT('Ctrl Pts',(-3.76685198944486,-2.39494457920613,
5.06751845741382));
#15075=CARTESIAN_POINT('Ctrl Pts',(-3.7666492146414,-2.38997815520014,5.06718495116665));
#15076=CARTESIAN_POINT('Ctrl Pts',(-3.7662039619217,-2.38503356610626,5.06685144491949));
#15077=CARTESIAN_POINT('Ctrl Pts',(-3.76125808275068,-2.33010893762799,
5.06314684856722));
#15078=CARTESIAN_POINT('Ctrl Pts',(-3.72639327521678,-2.27787848097877,
5.05944225221495));
#15079=CARTESIAN_POINT('Ctrl Pts',(-3.67756563230702,-2.25224574125102,
5.05573765586268));
#15080=CARTESIAN_POINT('Ctrl Pts',(-3.62873798939725,-2.22661300152326,
5.05203305951042));
#15081=CARTESIAN_POINT('Ctrl Pts',(-3.56594751111163,-2.22757797871697,
5.04832846315815));
#15082=CARTESIAN_POINT('Ctrl Pts',(-3.51793060783244,-2.25469905531577,
5.04462386680588));
#15083=CARTESIAN_POINT('Ctrl Pts',(-3.46991370455325,-2.28182013191457,
5.04091927045361));
#15084=CARTESIAN_POINT('Ctrl Pts',(-3.43667037628051,-2.33509730791846,
5.03721467410135));
#15085=CARTESIAN_POINT('Ctrl Pts',(-3.43341462472151,-2.39014797674899,
5.03351007774908));
#15086=CARTESIAN_POINT('Ctrl Pts',(-3.43015887316251,-2.44519864557951,
5.02980548139681));
#15087=CARTESIAN_POINT('Ctrl Pts',(-3.45689069831725,-2.50202280723666,
5.02610088504454));
#15088=CARTESIAN_POINT('Ctrl Pts',(-3.50137612681596,-2.53461456435925,
5.02239628869227));
#15089=CARTESIAN_POINT('Ctrl Pts',(-3.54586155531466,-2.56720632148184,
5.01869169234));
#15090=CARTESIAN_POINT('Ctrl Pts',(-3.60810058715733,-2.57556567406988,
5.01498709598774));
#15091=CARTESIAN_POINT('Ctrl Pts',(-3.65960917750461,-2.5558669157941,5.01128249963547));
#15092=CARTESIAN_POINT('Ctrl Pts',(-3.71111776785188,-2.53616815751832,
5.0075779032832));
#15093=CARTESIAN_POINT('Ctrl Pts',(-3.75189591670377,-2.48841128837874,
5.00387330693093));
#15094=CARTESIAN_POINT('Ctrl Pts',(-3.7632812725096,-2.4344525109445,5.00016871057867));
#15095=CARTESIAN_POINT('Ctrl Pts',(-3.76565462941201,-2.42320442708544,
4.9993964616061));
#15096=CARTESIAN_POINT('Ctrl Pts',(-3.7667507426838,-2.41168684356181,4.99862421263354));
#15097=CARTESIAN_POINT('Ctrl Pts',(-3.76664426409402,-2.40014916296054,
4.99785196366098));
#15098=CARTESIAN_POINT('Ctrl Pts',(-3.76634000649331,-2.40004261214866,
5.01714803633902));
#15099=CARTESIAN_POINT('Ctrl Pts',(-3.76639763409716,-2.42521541658955,
5.01882514925639));
#15100=CARTESIAN_POINT('Ctrl Pts',(-3.76104161906272,-2.45036494470439,
5.02050226217376));
#15101=CARTESIAN_POINT('Ctrl Pts',(-3.75014621732021,-2.47282762178721,
5.02217937509113));
#15102=CARTESIAN_POINT('Ctrl Pts',(-3.72607922389733,-2.52244571888807,
5.0258839714434));
#15103=CARTESIAN_POINT('Ctrl Pts',(-3.67498392204337,-2.55895387399913,
5.02958856779567));
#15104=CARTESIAN_POINT('Ctrl Pts',(-3.62024436531629,-2.56564393553624,
5.03329316414794));
#15105=CARTESIAN_POINT('Ctrl Pts',(-3.5655048085892,-2.57233399707334,5.03699776050021));
#15106=CARTESIAN_POINT('Ctrl Pts',(-3.50712099698899,-2.54920596503651,
5.04070235685248));
#15107=CARTESIAN_POINT('Ctrl Pts',(-3.47181261508692,-2.50684448916664,
5.04440695320474));
#15108=CARTESIAN_POINT('Ctrl Pts',(-3.43650423318484,-2.46448301329678,
5.04811154955701));
#15109=CARTESIAN_POINT('Ctrl Pts',(-3.42427128098091,-2.4028880935939,5.05181614590928));
#15110=CARTESIAN_POINT('Ctrl Pts',(-3.44071223414431,-2.35024904491843,
5.05552074226155));
#15111=CARTESIAN_POINT('Ctrl Pts',(-3.45715318730771,-2.29760999624296,
5.05922533861381));
#15112=CARTESIAN_POINT('Ctrl Pts',(-3.50226804583846,-2.2539268185949,5.06292993496608));
#15113=CARTESIAN_POINT('Ctrl Pts',(-3.55540974746646,-2.23919126462175,
5.06663453131835));
#15114=CARTESIAN_POINT('Ctrl Pts',(-3.60855144909447,-2.2244557106486,5.07033912767062));
#15115=CARTESIAN_POINT('Ctrl Pts',(-3.66971999381974,-2.23866778035036,
5.07404372402289));
#15116=CARTESIAN_POINT('Ctrl Pts',(-3.71092123316877,-2.27532344228896,
5.07774832037516));
#15117=CARTESIAN_POINT('Ctrl Pts',(-3.74576802981578,-2.30632572323287,
5.08088155902978));
#15118=CARTESIAN_POINT('Ctrl Pts',(-3.76633165591099,-2.35338253179949,
5.0840147976844));
#15119=CARTESIAN_POINT('Ctrl Pts',(-3.76673281282141,-2.40013003219325,
5.08714803633902));
#15120=CARTESIAN_POINT('Origin',(-3.6,-2.4,4.7));
#15121=CARTESIAN_POINT('',(-3.76674783764939,-2.3998784327954,5.15714803633902));
#15122=CARTESIAN_POINT('',(-3.76638442554721,-2.39990578503699,5.13785196366098));
#15123=CARTESIAN_POINT('',(-3.7666,-2.4,4.7));
#15124=CARTESIAN_POINT('',(-3.47309291201476,-2.29206413469515,5.2));
#15125=CARTESIAN_POINT('Ctrl Pts',(-3.76674783764939,-2.3998784327954,5.15714803633902));
#15126=CARTESIAN_POINT('Ctrl Pts',(-3.7663543041176,-2.44715561431286,5.16031823516921));
#15127=CARTESIAN_POINT('Ctrl Pts',(-3.74524548348422,-2.49473161213543,
5.1634884339994));
#15128=CARTESIAN_POINT('Ctrl Pts',(-3.70967617757414,-2.52575977295725,
5.16665863282959));
#15129=CARTESIAN_POINT('Ctrl Pts',(-3.66811098624533,-2.56201832251683,
5.17036322918186));
#15130=CARTESIAN_POINT('Ctrl Pts',(-3.60679922558629,-2.57567991185357,
5.17406782553412));
#15131=CARTESIAN_POINT('Ctrl Pts',(-3.55380862744679,-2.56038491971217,
5.17777242188639));
#15132=CARTESIAN_POINT('Ctrl Pts',(-3.5008180293073,-2.54508992757078,5.18147701823866));
#15133=CARTESIAN_POINT('Ctrl Pts',(-3.45614859368735,-2.50083835395125,
5.18518161459093));
#15134=CARTESIAN_POINT('Ctrl Pts',(-3.44024450358536,-2.44813181223257,
5.1888862109432));
#15135=CARTESIAN_POINT('Ctrl Pts',(-3.42434041348337,-2.39542527051388,
5.19259080729547));
#15136=CARTESIAN_POINT('Ctrl Pts',(-3.43720166889934,-2.33426376069605,
5.19629540364773));
#15137=CARTESIAN_POINT('Ctrl Pts',(-3.47309291201476,-2.29206413469515,
5.2));
#15138=CARTESIAN_POINT('',(-3.7271475418302,-2.29187968016137,5.2));
#15139=CARTESIAN_POINT('Origin',(-3.6,-2.4,5.2));
#15140=CARTESIAN_POINT('Ctrl Pts',(-3.72714769448933,-2.29187956305504,
5.2));
#15141=CARTESIAN_POINT('Ctrl Pts',(-3.69206190113039,-2.25072743961435,
5.19636770818144));
#15142=CARTESIAN_POINT('Ctrl Pts',(-3.6350641341643,-2.22812240899828,5.19273541636289));
#15143=CARTESIAN_POINT('Ctrl Pts',(-3.58132375070445,-2.23418207790235,
5.18910312454434));
#15144=CARTESIAN_POINT('Ctrl Pts',(-3.52651360920706,-2.24036237079714,
5.18539852819207));
#15145=CARTESIAN_POINT('Ctrl Pts',(-3.47509182514536,-2.27635992272048,
5.1816939318398));
#15146=CARTESIAN_POINT('Ctrl Pts',(-3.45055836147391,-2.3257410419838,5.17798933548753));
#15147=CARTESIAN_POINT('Ctrl Pts',(-3.42602489780247,-2.37512216124712,
5.17428473913526));
#15148=CARTESIAN_POINT('Ctrl Pts',(-3.42837975452128,-2.43788684785041,
5.170580142783));
#15149=CARTESIAN_POINT('Ctrl Pts',(-3.45656193213921,-2.48529019920904,
5.16687554643073));
#15150=CARTESIAN_POINT('Ctrl Pts',(-3.48474410975714,-2.53269355056767,
5.16317095007846));
#15151=CARTESIAN_POINT('Ctrl Pts',(-3.53875360827419,-2.56473556668165,
5.15946635372619));
#15152=CARTESIAN_POINT('Ctrl Pts',(-3.59386432904901,-2.56676216280164,
5.15576175737392));
#15153=CARTESIAN_POINT('Ctrl Pts',(-3.64897504982384,-2.56878875892163,
5.15205716102165));
#15154=CARTESIAN_POINT('Ctrl Pts',(-3.70518699285644,-2.54079993504764,
5.14835256466939));
#15155=CARTESIAN_POINT('Ctrl Pts',(-3.73677861120293,-2.49559987891255,
5.14464796831712));
#15156=CARTESIAN_POINT('Ctrl Pts',(-3.75609666594378,-2.46796035917884,
5.14238263343174));
#15157=CARTESIAN_POINT('Ctrl Pts',(-3.76620859684834,-2.43388515114326,
5.14011729854636));
#15158=CARTESIAN_POINT('Ctrl Pts',(-3.76638442554721,-2.39990578503699,
5.13785196366098));
#15159=CARTESIAN_POINT('Origin',(-3.6,-2.4,5.35459252805377));
#15160=CARTESIAN_POINT('',(-3.8057227013582,-2.39988044337606,4.34540747194623));
#15161=CARTESIAN_POINT('',(-3.80516111137892,-2.40008013262119,4.33959252805377));
#15162=CARTESIAN_POINT('',(-3.805475,-2.39999999999999,5.35459252805377));
#15163=CARTESIAN_POINT('',(-3.41173724903364,-2.48232321801035,4.3));
#15164=CARTESIAN_POINT('Ctrl Pts',(-3.80516111137892,-2.40008013262119,
4.33959252805377));
#15165=CARTESIAN_POINT('Ctrl Pts',(-3.80504330063484,-2.36152007992449,
4.33750880775931));
#15166=CARTESIAN_POINT('Ctrl Pts',(-3.77605833105766,-2.25423615375421,
4.33172049111259));
#15167=CARTESIAN_POINT('Ctrl Pts',(-3.60297473301061,-2.15700944143379,
4.32222757811361));
#15168=CARTESIAN_POINT('Ctrl Pts',(-3.39749761512046,-2.26611614077921,
4.3111137890568));
#15169=CARTESIAN_POINT('Ctrl Pts',(-3.38436282049399,-2.419721374356,4.30370459635227));
#15170=CARTESIAN_POINT('Ctrl Pts',(-3.41173724903364,-2.48232321801035,
4.3));
#15171=CARTESIAN_POINT('',(-3.47764162637991,-2.56553534042572,4.3));
#15172=CARTESIAN_POINT('Origin',(-3.6,-2.4,4.3));
#15173=CARTESIAN_POINT('Ctrl Pts',(-3.8057227013582,-2.39988044337606,4.34540747194623));
#15174=CARTESIAN_POINT('Ctrl Pts',(-3.8057729696998,-2.39271640638513,4.34501772883951));
#15175=CARTESIAN_POINT('Ctrl Pts',(-3.80218373546239,-2.3175070024762,4.34092338938053));
#15176=CARTESIAN_POINT('Ctrl Pts',(-3.70962995644976,-2.18326697275372,
4.33312445356927));
#15177=CARTESIAN_POINT('Ctrl Pts',(-3.47734459894833,-2.19039236572141,
4.32201066451247));
#15178=CARTESIAN_POINT('Ctrl Pts',(-3.35820162590419,-2.3879909133699,4.31096917998938));
#15179=CARTESIAN_POINT('Ctrl Pts',(-3.42405718781536,-2.52582031335719,
4.30363229181855));
#15180=CARTESIAN_POINT('Ctrl Pts',(-3.47764149510761,-2.56553553810743,
4.3));
#15181=CARTESIAN_POINT('Origin',(-3.6,-2.4,5.35459252805377));
#15182=CARTESIAN_POINT('',(-3.80519266468163,-2.39989734570579,4.41540747194623));
#15183=CARTESIAN_POINT('',(-3.80566724789774,-2.40014978098439,4.40959252805377));
#15184=CARTESIAN_POINT('',(-3.805475,-2.39999999999999,5.35459252805377));
#15185=CARTESIAN_POINT('Ctrl Pts',(-3.80566724789774,-2.40014978098439,
4.40959252805377));
#15186=CARTESIAN_POINT('Ctrl Pts',(-3.80518614471975,-2.34148051217519,
4.40640305253959));
#15187=CARTESIAN_POINT('Ctrl Pts',(-3.74813829229662,-2.21384966330463,
4.39950898067315));
#15188=CARTESIAN_POINT('Ctrl Pts',(-3.53156901893564,-2.16697244735031,
4.38891031245443));
#15189=CARTESIAN_POINT('Ctrl Pts',(-3.36710794136624,-2.33111753922242,
4.37779652339762));
#15190=CARTESIAN_POINT('Ctrl Pts',(-3.41581894666805,-2.55829572590735,
4.36668273434083));
#15191=CARTESIAN_POINT('Ctrl Pts',(-3.63310626972243,-2.64061568298545,
4.35556894528402));
#15192=CARTESIAN_POINT('Ctrl Pts',(-3.7850442261316,-2.5285041432322,4.34653887652167));
#15193=CARTESIAN_POINT('Ctrl Pts',(-3.80525275353212,-2.43007507309885,
4.34121340411158));
#15194=CARTESIAN_POINT('Ctrl Pts',(-3.80516111137892,-2.40008013262119,
4.33959252805377));
#15195=CARTESIAN_POINT('Ctrl Pts',(-3.80519266468163,-2.39989734570579,
4.41540747194623));
#15196=CARTESIAN_POINT('Ctrl Pts',(-3.80531782889597,-2.37222562131849,
4.41391197361979));
#15197=CARTESIAN_POINT('Ctrl Pts',(-3.78721617857279,-2.2761634023784,4.40871187894108));
#15198=CARTESIAN_POINT('Ctrl Pts',(-3.64121277969171,-2.16065653443092,
4.3998071879101));
#15199=CARTESIAN_POINT('Ctrl Pts',(-3.42126523797479,-2.23556891230323,
4.38869339885329));
#15200=CARTESIAN_POINT('Ctrl Pts',(-3.36491711226222,-2.46098554747977,
4.37757960979649));
#15201=CARTESIAN_POINT('Ctrl Pts',(-3.52374009350676,-2.63058418685777,
4.36646582073969));
#15202=CARTESIAN_POINT('Ctrl Pts',(-3.74435278297668,-2.59057501347053,
4.3557417747896));
#15203=CARTESIAN_POINT('Ctrl Pts',(-3.80529515774691,-2.46081219780934,
4.34872232519178));
#15204=CARTESIAN_POINT('Ctrl Pts',(-3.8057227013582,-2.39988044337606,4.34540747194623));
#15205=CARTESIAN_POINT('Origin',(-3.6,-2.4,5.35459252805377));
#15206=CARTESIAN_POINT('',(-3.80534991328218,-2.40017652766129,4.48540747194623));
#15207=CARTESIAN_POINT('',(-3.80562878759967,-2.39983660975823,4.47959252805377));
#15208=CARTESIAN_POINT('',(-3.805475,-2.39999999999999,5.35459252805377));
#15209=CARTESIAN_POINT('Ctrl Pts',(-3.80562878759967,-2.39983660975823,
4.47959252805377));
#15210=CARTESIAN_POINT('Ctrl Pts',(-3.80572325938657,-2.3889667780224,4.47900189367213));
#15211=CARTESIAN_POINT('Ctrl Pts',(-3.79999615684062,-2.31001856287219,
4.47470666293823));
#15212=CARTESIAN_POINT('Ctrl Pts',(-3.69773850858379,-2.17766949547173,
4.46670683585206));
#15213=CARTESIAN_POINT('Ctrl Pts',(-3.46621554409366,-2.19730464027232,
4.45559304679525));
#15214=CARTESIAN_POINT('Ctrl Pts',(-3.35714698343348,-2.40246926898597,
4.44447925773846));
#15215=CARTESIAN_POINT('Ctrl Pts',(-3.47036459479899,-2.60537350263611,
4.43336546868164));
#15216=CARTESIAN_POINT('Ctrl Pts',(-3.70223885894321,-2.62029753112878,
4.42225167962485));
#15217=CARTESIAN_POINT('Ctrl Pts',(-3.80084480548257,-2.48716469502641,
4.41432736608222));
#15218=CARTESIAN_POINT('Ctrl Pts',(-3.80574494915964,-2.40962524577001,
4.41010764889186));
#15219=CARTESIAN_POINT('Ctrl Pts',(-3.80566724789774,-2.40014978098439,
4.40959252805377));
#15220=CARTESIAN_POINT('Ctrl Pts',(-3.80534991328218,-2.40017652766129,
4.48540747194623));
#15221=CARTESIAN_POINT('Ctrl Pts',(-3.8049563333145,-2.35213729171836,4.48280621840006));
#15222=CARTESIAN_POINT('Ctrl Pts',(-3.76418777806192,-2.23508077339291,
4.47650036850163));
#15223=CARTESIAN_POINT('Ctrl Pts',(-3.56918135654791,-2.15909775573836,
4.46648992225092));
#15224=CARTESIAN_POINT('Ctrl Pts',(-3.38089013692747,-2.29524052189659,
4.45537613319412));
#15225=CARTESIAN_POINT('Ctrl Pts',(-3.39315268252002,-2.52727080497827,
4.44426234413731));
#15226=CARTESIAN_POINT('Ctrl Pts',(-3.59474487821944,-2.64280871984201,
4.43314855508051));
#15227=CARTESIAN_POINT('Ctrl Pts',(-3.77337323688511,-2.5504598261374,4.42353026435015));
#15228=CARTESIAN_POINT('Ctrl Pts',(-3.80500777646484,-2.44077305290937,
4.41761656997206));
#15229=CARTESIAN_POINT('Ctrl Pts',(-3.80519266468163,-2.39989734570579,
4.41540747194623));
#15230=CARTESIAN_POINT('Origin',(-3.6,-2.4,5.35459252805377));
#15231=CARTESIAN_POINT('',(-3.80581595477291,-2.39999917227814,4.55540747194623));
#15232=CARTESIAN_POINT('',(-3.80515176250663,-2.39995310238523,4.54959252805377));
#15233=CARTESIAN_POINT('',(-3.805475,-2.39999999999999,5.35459252805377));
#15234=CARTESIAN_POINT('Ctrl Pts',(-3.80515176250663,-2.39995310238523,
4.54959252805377));
#15235=CARTESIAN_POINT('Ctrl Pts',(-3.80521587176166,-2.36854855820361,
4.54789613845241));
#15236=CARTESIAN_POINT('Ctrl Pts',(-3.78367651299531,-2.26864576859469,
4.54249515249878));
#15237=CARTESIAN_POINT('Ctrl Pts',(-3.62821111895818,-2.15877850380716,
4.53338957019289));
#15238=CARTESIAN_POINT('Ctrl Pts',(-3.4126363777684,-2.24547313898512,4.52227578113608));
#15239=CARTESIAN_POINT('Ctrl Pts',(-3.3685576844537,-2.47360796440317,4.51116199207928));
#15240=CARTESIAN_POINT('Ctrl Pts',(-3.53632076809686,-2.63436858142862,
4.50004820302248));
#15241=CARTESIAN_POINT('Ctrl Pts',(-3.75035693907624,-2.58346600089298,
4.4895250483473));
#15242=CARTESIAN_POINT('Ctrl Pts',(-3.80513071034435,-2.45714489336835,
4.4827064900244));
#15243=CARTESIAN_POINT('Ctrl Pts',(-3.80562878759967,-2.39983660975823,
4.47959252805377));
#15244=CARTESIAN_POINT('Ctrl Pts',(-3.80581595309039,-2.39999917228222,
4.55540747194623));
#15245=CARTESIAN_POINT('Ctrl Pts',(-3.80581595573579,-2.39995488126346,
4.55540505953261));
#15246=CARTESIAN_POINT('Ctrl Pts',(-3.805795885724,-2.33189557869137,4.55169805076671));
#15247=CARTESIAN_POINT('Ctrl Pts',(-3.73158417960078,-2.19586944742698,
4.54428644564855));
#15248=CARTESIAN_POINT('Ctrl Pts',(-3.49986236155564,-2.17873967321655,
4.53317265659175));
#15249=CARTESIAN_POINT('Ctrl Pts',(-3.35979765944108,-2.36413198553984,
4.52205886753494));
#15250=CARTESIAN_POINT('Ctrl Pts',(-3.43959288407154,-2.58235469793693,
4.51094507847814));
#15251=CARTESIAN_POINT('Ctrl Pts',(-3.66621056034765,-2.6336660879353,4.49983128942134));
#15252=CARTESIAN_POINT('Ctrl Pts',(-3.79336822690886,-2.50914983096546,
4.4913187539107));
#15253=CARTESIAN_POINT('Ctrl Pts',(-3.80551685342017,-2.42055275952314,
4.48651081475233));
#15254=CARTESIAN_POINT('Ctrl Pts',(-3.80534991328218,-2.40017652766129,
4.48540747194623));
#15255=CARTESIAN_POINT('Origin',(-3.6,-2.4,5.35459252805377));
#15256=CARTESIAN_POINT('',(-3.80534749847032,-2.39982399268994,4.62540747194623));
#15257=CARTESIAN_POINT('',(-3.80545680064795,-2.40018789159516,4.61959252805377));
#15258=CARTESIAN_POINT('',(-3.805475,-2.39999999999999,5.35459252805377));
#15259=CARTESIAN_POINT('Ctrl Pts',(-3.80545680064795,-2.40018789159516,
4.61959252805377));
#15260=CARTESIAN_POINT('Ctrl Pts',(-3.80498629881388,-2.34850704133116,
4.61679038323269));
#15261=CARTESIAN_POINT('Ctrl Pts',(-3.75902064354221,-2.22775548399901,
4.61028364205933));
#15262=CARTESIAN_POINT('Ctrl Pts',(-3.55620097341096,-2.16111650777606,
4.60007230453371));
#15263=CARTESIAN_POINT('Ctrl Pts',(-3.37554637252617,-2.307240921179,4.58895851547691));
#15264=CARTESIAN_POINT('Ctrl Pts',(-3.40033672233922,-2.53826877141577,
4.57784472642011));
#15265=CARTESIAN_POINT('Ctrl Pts',(-3.60788113454322,-2.64273764704216,
4.5667309373633));
#15266=CARTESIAN_POINT('Ctrl Pts',(-3.7776337191139,-2.54299330423865,4.55731353790786));
#15267=CARTESIAN_POINT('Ctrl Pts',(-3.80507586918669,-2.43713018575349,
4.55160073480468));
#15268=CARTESIAN_POINT('Ctrl Pts',(-3.80515176250663,-2.39995310238523,
4.54959252805377));
#15269=CARTESIAN_POINT('Ctrl Pts',(-3.80534749847032,-2.39982399268994,
4.62540747194623));
#15270=CARTESIAN_POINT('Ctrl Pts',(-3.8055145307928,-2.37935804813576,4.62429930431288));
#15271=CARTESIAN_POINT('Ctrl Pts',(-3.79329841632202,-2.29066951260838,
4.61948654032727));
#15272=CARTESIAN_POINT('Ctrl Pts',(-3.66590691978443,-2.16624808716256,
4.61096917998938));
#15273=CARTESIAN_POINT('Ctrl Pts',(-3.4393560992794,-2.21785386089149,4.59985539093257));
#15274=CARTESIAN_POINT('Ctrl Pts',(-3.35984446292695,-2.43618006142673,
4.58874160187577));
#15275=CARTESIAN_POINT('Ctrl Pts',(-3.50014991321196,-2.62139024142312,
4.57762781281897));
#15276=CARTESIAN_POINT('Ctrl Pts',(-3.73179898649779,-2.60396320633826,
4.56651643617578));
#15277=CARTESIAN_POINT('Ctrl Pts',(-3.80581189336919,-2.46796989528688,
4.55910965588487));
#15278=CARTESIAN_POINT('Ctrl Pts',(-3.80581595309039,-2.39999917228222,
4.55540747194623));
#15279=CARTESIAN_POINT('Origin',(-3.6,-2.4,5.35459252805377));
#15280=CARTESIAN_POINT('',(-3.80519404433776,-2.40010391087563,4.69540747194623));
#15281=CARTESIAN_POINT('',(-3.80578860319875,-2.39993212258736,4.68959252805377));
#15282=CARTESIAN_POINT('',(-3.805475,-2.39999999999999,5.35459252805377));
#15283=CARTESIAN_POINT('Ctrl Pts',(-3.80578860319875,-2.39993212258736,
4.68959252805377));
#15284=CARTESIAN_POINT('Ctrl Pts',(-3.80580467529652,-2.39619821380325,
4.68938922436523));
#15285=CARTESIAN_POINT('Ctrl Pts',(-3.8040203847709,-2.32444075317719,4.68548132432442));
#15286=CARTESIAN_POINT('Ctrl Pts',(-3.72035445765201,-2.18905336667194,
4.67786882793134));
#15287=CARTESIAN_POINT('Ctrl Pts',(-3.4880454122232,-2.18447773232253,4.66675503887454));
#15288=CARTESIAN_POINT('Ctrl Pts',(-3.35820967063793,-2.37717207376684,
4.65564124981773));
#15289=CARTESIAN_POINT('Ctrl Pts',(-3.4496873596065,-2.5907610749791,4.64452746076093));
#15290=CARTESIAN_POINT('Ctrl Pts',(-3.67874791298872,-2.62974430088435,
4.63341367170412));
#15291=CARTESIAN_POINT('Ctrl Pts',(-3.79614945789441,-2.50163131370898,
4.62510202746841));
#15292=CARTESIAN_POINT('Ctrl Pts',(-3.80560832925468,-2.41683209288794,
4.62049497958495));
#15293=CARTESIAN_POINT('Ctrl Pts',(-3.80545680064795,-2.40018789159516,
4.61959252805377));
#15294=CARTESIAN_POINT('Ctrl Pts',(-3.80519404433776,-2.40010391087563,
4.69540747194623));
#15295=CARTESIAN_POINT('Ctrl Pts',(-3.80500644622954,-2.35913959443751,
4.69319354909316));
#15296=CARTESIAN_POINT('Ctrl Pts',(-3.77326723416865,-2.24936122008858,
4.68727502988781));
#15297=CARTESIAN_POINT('Ctrl Pts',(-3.59442944460758,-2.15719833661306,
4.6776519143302));
#15298=CARTESIAN_POINT('Ctrl Pts',(-3.3929874908777,-2.27299803191391,4.6665381252734));
#15299=CARTESIAN_POINT('Ctrl Pts',(-3.38102643442896,-2.50504406890429,
4.65542433621659));
#15300=CARTESIAN_POINT('Ctrl Pts',(-3.5694943658766,-2.64094207834572,4.64431054715979));
#15301=CARTESIAN_POINT('Ctrl Pts',(-3.76430796656755,-2.56474251573525,
4.63430492573634));
#15302=CARTESIAN_POINT('Ctrl Pts',(-3.8049561429515,-2.44777555218424,4.62800390066515));
#15303=CARTESIAN_POINT('Ctrl Pts',(-3.80534749847032,-2.39982399268994,
4.62540747194623));
#15304=CARTESIAN_POINT('Origin',(-3.6,-2.4,5.35459252805377));
#15305=CARTESIAN_POINT('',(-3.80572671416466,-2.40012021867279,4.76540747194623));
#15306=CARTESIAN_POINT('',(-3.80525640542964,-2.39985490132803,4.75959252805377));
#15307=CARTESIAN_POINT('',(-3.805475,-2.39999999999999,5.35459252805377));
#15308=CARTESIAN_POINT('Ctrl Pts',(-3.80525640542964,-2.39985490132803,
4.75959252805377));
#15309=CARTESIAN_POINT('Ctrl Pts',(-3.80541421756911,-2.37565177743561,
4.7582834691455));
#15310=CARTESIAN_POINT('Ctrl Pts',(-3.7902631541036,-2.2831457592228,4.75326981388497));
#15311=CARTESIAN_POINT('Ctrl Pts',(-3.65317166084996,-2.16302647390142,
4.74455156227217));
#15312=CARTESIAN_POINT('Ctrl Pts',(-3.42974254509416,-2.22680624538361,
4.73343777321536));
#15313=CARTESIAN_POINT('Ctrl Pts',(-3.36215200866455,-2.44911222461694,
4.72232398415856));
#15314=CARTESIAN_POINT('Ctrl Pts',(-3.51226643608395,-2.62646522768789,
4.71121019510176));
#15315=CARTESIAN_POINT('Ctrl Pts',(-3.73846937161942,-2.59707960507412,
4.70029970973349));
#15316=CARTESIAN_POINT('Ctrl Pts',(-3.80551180980452,-2.46423743611441,
4.6930938207175));
#15317=CARTESIAN_POINT('Ctrl Pts',(-3.80578860319875,-2.39993212258736,
4.68959252805377));
#15318=CARTESIAN_POINT('Ctrl Pts',(-3.80572671416466,-2.40012021867279,
4.76540747194623));
#15319=CARTESIAN_POINT('Ctrl Pts',(-3.80530257178557,-2.33910193112031,
4.76208779387343));
#15320=CARTESIAN_POINT('Ctrl Pts',(-3.74420123427486,-2.20925254264417,
4.75506351944836));
#15321=CARTESIAN_POINT('Ctrl Pts',(-3.52344221265408,-2.16951662960737,
4.74433464867103));
#15322=CARTESIAN_POINT('Ctrl Pts',(-3.36483725976158,-2.33931915924769,
4.73322085961422));
#15323=CARTESIAN_POINT('Ctrl Pts',(-3.42147942993616,-2.56466355059616,
4.72210707055742));
#15324=CARTESIAN_POINT('Ctrl Pts',(-3.64152350245114,-2.63928952667227,
4.71099328150061));
#15325=CARTESIAN_POINT('Ctrl Pts',(-3.78729792557216,-2.52365598332802,
4.70209341529689));
#15326=CARTESIAN_POINT('Ctrl Pts',(-3.80532035746924,-2.42768591123397,
4.69689814544542));
#15327=CARTESIAN_POINT('Ctrl Pts',(-3.80519404433776,-2.40010391087563,
4.69540747194623));
#15328=CARTESIAN_POINT('Origin',(-3.6,-2.4,5.35459252805377));
#15329=CARTESIAN_POINT('',(-3.80555826192291,-2.39982008596012,4.83540747194623));
#15330=CARTESIAN_POINT('',(-3.80526423797111,-2.40014879660671,4.82959252805377));
#15331=CARTESIAN_POINT('',(-3.805475,-2.39999999999999,5.35459252805377));
#15332=CARTESIAN_POINT('Ctrl Pts',(-3.80526423797112,-2.40014879660671,
4.82959252805377));
#15333=CARTESIAN_POINT('Ctrl Pts',(-3.80496497000794,-2.35550570352956,
4.82717771392578));
#15334=CARTESIAN_POINT('Ctrl Pts',(-3.7687007786119,-2.24193241424781,4.82105830344552));
#15335=CARTESIAN_POINT('Ctrl Pts',(-3.58130943002562,-2.15785471265546,
4.81123429661298));
#15336=CARTESIAN_POINT('Ctrl Pts',(-3.38642338383962,-2.28437687679961,
4.8001205075562));
#15337=CARTESIAN_POINT('Ctrl Pts',(-3.38702643654876,-2.51673019686447,
4.78900671849938));
#15338=CARTESIAN_POINT('Ctrl Pts',(-3.58256660716932,-2.64223904392882,
4.77789292944258));
#15339=CARTESIAN_POINT('Ctrl Pts',(-3.76915216315368,-2.5573566497576,4.76808819929404));
#15340=CARTESIAN_POINT('Ctrl Pts',(-3.80496761407973,-2.44414587187183,
4.76198806549777));
#15341=CARTESIAN_POINT('Ctrl Pts',(-3.80525640542964,-2.39985490132803,
4.75959252805377));
#15342=CARTESIAN_POINT('Ctrl Pts',(-3.80555826192291,-2.39982008596012,
4.83540747194623));
#15343=CARTESIAN_POINT('Ctrl Pts',(-3.80567994930423,-2.38654227868304,
4.83468663500597));
#15344=CARTESIAN_POINT('Ctrl Pts',(-3.79845786380229,-2.30515766788849,
4.83026120171345));
#15345=CARTESIAN_POINT('Ctrl Pts',(-3.68988494304833,-2.17438001896094,
4.82213117206866));
#15346=CARTESIAN_POINT('Ctrl Pts',(-3.45919253805822,-2.20211888040452,
4.81101738301185));
#15347=CARTESIAN_POINT('Ctrl Pts',(-3.35738279984868,-2.41098057473832,
4.79990359395505));
#15348=CARTESIAN_POINT('Ctrl Pts',(-3.47764333640382,-2.60979162448597,
4.78878980489824));
#15349=CARTESIAN_POINT('Ctrl Pts',(-3.7098983147675,-2.61657802114276,4.77767601584144));
#15350=CARTESIAN_POINT('Ctrl Pts',(-3.80223426786157,-2.48231400602396,
4.76988190485744));
#15351=CARTESIAN_POINT('Ctrl Pts',(-3.80577589367883,-2.40719531865107,
4.7657923902257));
#15352=CARTESIAN_POINT('Ctrl Pts',(-3.80572671416466,-2.40012021867279,
4.76540747194623));
#15353=CARTESIAN_POINT('Origin',(-3.6,-2.4,5.35459252805377));
#15354=CARTESIAN_POINT('',(-3.80514217248594,-2.39999218980904,4.90540747194623));
#15355=CARTESIAN_POINT('',(-3.80579332868662,-2.40006173798069,4.89959252805377));
#15356=CARTESIAN_POINT('',(-3.805475,-2.39999999999999,5.35459252805377));
#15357=CARTESIAN_POINT('Ctrl Pts',(-3.80579332868662,-2.40006173798069,
4.89959252805377));
#15358=CARTESIAN_POINT('Ctrl Pts',(-3.80553739175956,-2.33540634391997,
4.89607195870605));
#15359=CARTESIAN_POINT('Ctrl Pts',(-3.73784442753819,-2.20225412798971,
4.88884679300607));
#15360=CARTESIAN_POINT('Ctrl Pts',(-3.511092084609,-2.17399322981363,4.87791703095382));
#15361=CARTESIAN_POINT('Ctrl Pts',(-3.36190028176488,-2.35212305601353,
4.86680324189701));
#15362=CARTESIAN_POINT('Ctrl Pts',(-3.43064385125587,-2.57407519200526,
4.85568945284021));
#15363=CARTESIAN_POINT('Ctrl Pts',(-3.6544010243217,-2.63669433060785,4.84457566378341));
#15364=CARTESIAN_POINT('Ctrl Pts',(-3.79056542018395,-2.51613221267343,
4.83587668885459));
#15365=CARTESIAN_POINT('Ctrl Pts',(-3.80542408070796,-2.42399322720708,
4.83088231027805));
#15366=CARTESIAN_POINT('Ctrl Pts',(-3.80526423797112,-2.40014879660671,
4.82959252805377));
#15367=CARTESIAN_POINT('Ctrl Pts',(-3.80514217248594,-2.39999218980904,
4.90540747194623));
#15368=CARTESIAN_POINT('Ctrl Pts',(-3.80515363847659,-2.36617331522009,
4.90358087978625));
#15369=CARTESIAN_POINT('Ctrl Pts',(-3.78123591841218,-2.26378007899297,
4.898049691274));
#15370=CARTESIAN_POINT('Ctrl Pts',(-3.61973808033182,-2.15793784472475,
4.88881390640949));
#15371=CARTESIAN_POINT('Ctrl Pts',(-3.4073347883606,-2.25213588990288,4.87770011735268));
#15372=CARTESIAN_POINT('Ctrl Pts',(-3.37128014957741,-2.48167563194308,
4.86658632829587));
#15373=CARTESIAN_POINT('Ctrl Pts',(-3.54457538374435,-2.63645674180255,
4.85547253923907));
#15374=CARTESIAN_POINT('Ctrl Pts',(-3.75407113935919,-2.57880494205606,
4.84507958712253));
#15375=CARTESIAN_POINT('Ctrl Pts',(-3.8050545615032,-2.45478089640322,4.83839123135824));
#15376=CARTESIAN_POINT('Ctrl Pts',(-3.80555826192291,-2.39982008596012,
4.83540747194623));
#15377=CARTESIAN_POINT('Origin',(-3.6,-2.4,5.35459252805377));
#15378=CARTESIAN_POINT('',(-3.80552959282545,-2.40018396914357,4.97540747194623));
#15379=CARTESIAN_POINT('',(-3.80544614170703,-2.39981229694107,4.96959252805377));
#15380=CARTESIAN_POINT('',(-3.805475,-2.39999999999999,5.35459252805377));
#15381=CARTESIAN_POINT('Ctrl Pts',(-3.80544614170703,-2.39981229694107,
4.96959252805377));
#15382=CARTESIAN_POINT('Ctrl Pts',(-3.80560005255251,-2.38281031937819,
4.9686707998386));
#15383=CARTESIAN_POINT('Ctrl Pts',(-3.79589308932397,-2.29764759199308,
4.96404447527115));
#15384=CARTESIAN_POINT('Ctrl Pts',(-3.67755429765177,-2.16985003043886,
4.95571355435145));
#15385=CARTESIAN_POINT('Ctrl Pts',(-3.44869918397279,-2.21002173633656,
4.94459976529464));
#15386=CARTESIAN_POINT('Ctrl Pts',(-3.3583314230664,-2.42408270152555,4.93348597623784));
#15387=CARTESIAN_POINT('Ctrl Pts',(-3.48916565133794,-2.61610049686178,
4.92237218718103));
#15388=CARTESIAN_POINT('Ctrl Pts',(-3.7214478158856,-2.61031905668909,4.91125839812423));
#15389=CARTESIAN_POINT('Ctrl Pts',(-3.80419976839027,-2.4748431306509,4.90366517841514));
#15390=CARTESIAN_POINT('Ctrl Pts',(-3.8058067070074,-2.4034414011323,4.89977655505832));
#15391=CARTESIAN_POINT('Ctrl Pts',(-3.80579332868662,-2.40006173798069,
4.89959252805377));
#15392=CARTESIAN_POINT('Ctrl Pts',(-3.80552959282545,-2.40018396914357,
4.97540747194623));
#15393=CARTESIAN_POINT('Ctrl Pts',(-3.80503093302249,-2.34615078230832,
4.97247512456653));
#15394=CARTESIAN_POINT('Ctrl Pts',(-3.75549941719541,-2.22304560401132,
4.96583818083455));
#15395=CARTESIAN_POINT('Ctrl Pts',(-3.54785414492032,-2.16279863265717,
4.9554966407503));
#15396=CARTESIAN_POINT('Ctrl Pts',(-3.37243276525931,-2.31516585290104,
4.94438285169351));
#15397=CARTESIAN_POINT('Ctrl Pts',(-3.40530625649813,-2.54518272988275,
4.9332690626367));
#15398=CARTESIAN_POINT('Ctrl Pts',(-3.61638513906469,-2.64231220781178,
4.9221552735799));
#15399=CARTESIAN_POINT('Ctrl Pts',(-3.78023982132068,-2.53813917250258,
4.91286807668307));
#15400=CARTESIAN_POINT('Ctrl Pts',(-3.80513038376869,-2.43476294468685,
4.90728547613852));
#15401=CARTESIAN_POINT('Ctrl Pts',(-3.80514217248594,-2.39999218980904,
4.90540747194623));
#15402=CARTESIAN_POINT('Origin',(-3.6,-2.4,5.35459252805377));
#15403=CARTESIAN_POINT('',(-3.80574710647333,-2.39989343748479,5.04540747194623));
#15404=CARTESIAN_POINT('',(-3.80515433874078,-2.40005255540964,5.03959252805377));
#15405=CARTESIAN_POINT('',(-3.805475,-2.39999999999999,5.35459252805377));
#15406=CARTESIAN_POINT('Ctrl Pts',(-3.80515433874078,-2.40005255540964,
5.03959252805377));
#15407=CARTESIAN_POINT('Ctrl Pts',(-3.80506841571452,-2.36251978652027,
5.03756504461887));
#15408=CARTESIAN_POINT('Ctrl Pts',(-3.77723760351786,-2.25628892207963,
5.0318329648317));
#15409=CARTESIAN_POINT('Ctrl Pts',(-3.60662102802227,-2.15722471599323,
5.02239628869228));
#15410=CARTESIAN_POINT('Ctrl Pts',(-3.39962168818772,-2.262769500459,5.01128249963546));
#15411=CARTESIAN_POINT('Ctrl Pts',(-3.37603088927244,-2.49392292132789,
5.00016871057867));
#15412=CARTESIAN_POINT('Ctrl Pts',(-3.55744155755193,-2.63910762521254,
4.98905492152185));
#15413=CARTESIAN_POINT('Ctrl Pts',(-3.75953036700652,-2.57154453779223,
4.97886286068023));
#15414=CARTESIAN_POINT('Ctrl Pts',(-3.80498145636834,-2.45114441507362,
4.97237539619086));
#15415=CARTESIAN_POINT('Ctrl Pts',(-3.80544614170703,-2.39981229694107,
4.96959252805377));
#15416=CARTESIAN_POINT('Ctrl Pts',(-3.80574710647333,-2.39989343748479,
5.04540747194623));
#15417=CARTESIAN_POINT('Ctrl Pts',(-3.80578578950289,-2.39376493044645,
5.04507396569907));
#15418=CARTESIAN_POINT('Ctrl Pts',(-3.80275768152815,-2.31959956136467,
5.04103586309964));
#15419=CARTESIAN_POINT('Ctrl Pts',(-3.71288602579316,-2.18496415245566,
5.03329316414794));
#15420=CARTESIAN_POINT('Ctrl Pts',(-3.4805593716682,-2.1885345970333,5.02217937509112));
#15421=CARTESIAN_POINT('Ctrl Pts',(-3.35755805936012,-2.38566174720256,
5.01106558603434));
#15422=CARTESIAN_POINT('Ctrl Pts',(-3.45646661470834,-2.59591285074103,
4.99995179697752));
#15423=CARTESIAN_POINT('Ctrl Pts',(-3.68675290044432,-2.62684270619768,
4.98883800792072));
#15424=CARTESIAN_POINT('Ctrl Pts',(-3.79782383930996,-2.49676322878239,
4.98065656624362));
#15425=CARTESIAN_POINT('Ctrl Pts',(-3.80566091748472,-2.41441389064144,
4.9761797209188));
#15426=CARTESIAN_POINT('Ctrl Pts',(-3.80552959282545,-2.40018396914357,
4.97540747194623));
#15427=CARTESIAN_POINT('Origin',(-3.6,-2.4,5.35459252805377));
#15428=CARTESIAN_POINT('',(-3.80520912268496,-2.39988380060309,5.11540747194623));
#15429=CARTESIAN_POINT('',(-3.8056388038084,-2.40016037433918,5.10959252805377));
#15430=CARTESIAN_POINT('',(-3.805475,-2.39999999999999,5.35459252805377));
#15431=CARTESIAN_POINT('Ctrl Pts',(-3.8056388038084,-2.40016037433918,5.10959252805377));
#15432=CARTESIAN_POINT('Ctrl Pts',(-3.80514403960571,-2.34250465619148,
5.10645928939915));
#15433=CARTESIAN_POINT('Ctrl Pts',(-3.74979516025411,-2.21584695448232,
5.09962145439226));
#15434=CARTESIAN_POINT('Ctrl Pts',(-3.53510505567384,-2.16596525884485,
5.0890790230331));
#15435=CARTESIAN_POINT('Ctrl Pts',(-3.36817872512274,-2.32759432716241,
5.07796523397629));
#15436=CARTESIAN_POINT('Ctrl Pts',(-3.41344101541272,-2.5554973786501,5.06685144491949));
#15437=CARTESIAN_POINT('Ctrl Pts',(-3.62946287054873,-2.64107179130501,
5.05573765586269));
#15438=CARTESIAN_POINT('Ctrl Pts',(-3.78402795903722,-2.53063333570257,
5.04665135024078));
#15439=CARTESIAN_POINT('Ctrl Pts',(-3.80522541336203,-2.43109926604885,
5.04126964097114));
#15440=CARTESIAN_POINT('Ctrl Pts',(-3.80515433874078,-2.40005255540964,
5.03959252805377));
#15441=CARTESIAN_POINT('Ctrl Pts',(-3.80520912268496,-2.39988380060309,
5.11540747194623));
#15442=CARTESIAN_POINT('Ctrl Pts',(-3.80534690105405,-2.37325776244818,
5.11396821047934));
#15443=CARTESIAN_POINT('Ctrl Pts',(-3.78816006360229,-2.27826799235566,
5.10882435266019));
#15444=CARTESIAN_POINT('Ctrl Pts',(-3.64483147519039,-2.16130911215383,
5.09997589848876));
#15445=CARTESIAN_POINT('Ctrl Pts',(-3.42377645640768,-2.23288040078699,
5.08886210943196));
#15446=CARTESIAN_POINT('Ctrl Pts',(-3.36401956629289,-2.45741970591997,
5.07774832037515));
#15447=CARTESIAN_POINT('Ctrl Pts',(-3.52025888222192,-2.62940132794335,
5.06663453131835));
#15448=CARTESIAN_POINT('Ctrl Pts',(-3.74260711073009,-2.59254976529191,
5.05585424850871));
#15449=CARTESIAN_POINT('Ctrl Pts',(-3.8053560973714,-2.46184055125472,5.04877856205134));
#15450=CARTESIAN_POINT('Ctrl Pts',(-3.80574710647333,-2.39989343748479,
5.04540747194623));
#15451=CARTESIAN_POINT('Origin',(-3.6,-2.4,5.35459252805377));
#15452=CARTESIAN_POINT('',(-3.80526708169851,-2.40022955265959,5.18540747194623));
#15453=CARTESIAN_POINT('',(-3.80565733457988,-2.39985006589819,5.17959252805377));
#15454=CARTESIAN_POINT('',(-3.805475,-2.39999999999999,5.35459252805377));
#15455=CARTESIAN_POINT('',(-3.65301702171886,-2.59851743256717,5.2));
#15456=CARTESIAN_POINT('Ctrl Pts',(-3.65301702171886,-2.59851743256717,
5.2));
#15457=CARTESIAN_POINT('Ctrl Pts',(-3.71902879097456,-2.58088801151799,
5.19629540364773));
#15458=CARTESIAN_POINT('Ctrl Pts',(-3.79249438127854,-2.51127182149751,
5.19143122762981));
#15459=CARTESIAN_POINT('Ctrl Pts',(-3.80542872863858,-2.42165306802236,
5.18656705161189));
#15460=CARTESIAN_POINT('Ctrl Pts',(-3.80526708169851,-2.40022955265959,
5.18540747194623));
#15461=CARTESIAN_POINT('',(-3.54686845990025,-2.59887322544328,5.2));
#15462=CARTESIAN_POINT('Origin',(-3.6,-2.4,5.2));
#15463=CARTESIAN_POINT('Ctrl Pts',(-3.54686838721289,-2.59887345127292,
5.2));
#15464=CARTESIAN_POINT('Ctrl Pts',(-3.61132827149734,-2.61600531405712,
5.19636770818144));
#15465=CARTESIAN_POINT('Ctrl Pts',(-3.74930830903252,-2.58406706978518,
5.18956521753271));
#15466=CARTESIAN_POINT('Ctrl Pts',(-3.80517197262043,-2.45815906273072,
5.18276272688396));
#15467=CARTESIAN_POINT('Ctrl Pts',(-3.80565733457988,-2.39985006589818,
5.17959252805377));
#15468=CARTESIAN_POINT('Origin',(3.6,-2.4,4.7));
#15469=CARTESIAN_POINT('',(3.4332441194689,-2.40012144310043,4.38714803633902));
#15470=CARTESIAN_POINT('',(3.43319918361158,-2.39990306414324,4.36785196366098));
#15471=CARTESIAN_POINT('',(3.4334,-2.4,4.7));
#15472=CARTESIAN_POINT('',(3.43648706727485,-2.43192304546281,4.3));
#15473=CARTESIAN_POINT('Ctrl Pts',(3.43319918361158,-2.39990306414324,4.36785196366098));
#15474=CARTESIAN_POINT('Ctrl Pts',(3.43315842575224,-2.39409443322767,4.36746222055426));
#15475=CARTESIAN_POINT('Ctrl Pts',(3.43343544638748,-2.38828969410672,4.36707247744754));
#15476=CARTESIAN_POINT('Ctrl Pts',(3.43404308035483,-2.38251974365232,4.36668273434082));
#15477=CARTESIAN_POINT('Ctrl Pts',(3.43981877860357,-2.32767505996788,4.36297813798856));
#15478=CARTESIAN_POINT('Ctrl Pts',(3.47546516768456,-2.27597350876472,4.35927354163629));
#15479=CARTESIAN_POINT('Ctrl Pts',(3.52467802663468,-2.2510856178596,4.35556894528402));
#15480=CARTESIAN_POINT('Ctrl Pts',(3.57389088558479,-2.22619772695447,4.35186434893175));
#15481=CARTESIAN_POINT('Ctrl Pts',(3.63667021440403,-2.22812349634739,4.34815975257949));
#15482=CARTESIAN_POINT('Ctrl Pts',(3.68426556377096,-2.25596352517201,4.34445515622722));
#15483=CARTESIAN_POINT('Ctrl Pts',(3.73186091313788,-2.28380355399663,4.34075055987495));
#15484=CARTESIAN_POINT('Ctrl Pts',(3.7642722830525,-2.33755784225296,4.33704596352268));
#15485=CARTESIAN_POINT('Ctrl Pts',(3.76670489686818,-2.39266164590465,4.33334136717041));
#15486=CARTESIAN_POINT('Ctrl Pts',(3.76913751068386,-2.44776544955635,4.32963677081814));
#15487=CARTESIAN_POINT('Ctrl Pts',(3.74159136840061,-2.50421876860342,4.32593217446587));
#15488=CARTESIAN_POINT('Ctrl Pts',(3.69659414024548,-2.53611221831126,4.32222757811361));
#15489=CARTESIAN_POINT('Ctrl Pts',(3.65159691209034,-2.56800566801911,4.31852298176134));
#15490=CARTESIAN_POINT('Ctrl Pts',(3.58914859806332,-2.57533924838774,4.31481838540907));
#15491=CARTESIAN_POINT('Ctrl Pts',(3.53802492988379,-2.55491157781525,4.3111137890568));
#15492=CARTESIAN_POINT('Ctrl Pts',(3.48690126170426,-2.53448390724277,4.30740919270454));
#15493=CARTESIAN_POINT('Ctrl Pts',(3.44710223937223,-2.48629498572918,4.30370459635227));
#15494=CARTESIAN_POINT('Ctrl Pts',(3.43648706727485,-2.43192304546281,4.3));
#15495=CARTESIAN_POINT('',(3.59474332937116,-2.23318013131002,4.3));
#15496=CARTESIAN_POINT('Origin',(3.6,-2.4,4.3));
#15497=CARTESIAN_POINT('',(3.43365449489478,-2.40006497081539,4.31714803633902));
#15498=CARTESIAN_POINT('Ctrl Pts',(3.5947433329992,-2.23317993884958,4.3));
#15499=CARTESIAN_POINT('Ctrl Pts',(3.54069367702075,-2.23495318942066,4.30363229181855));
#15500=CARTESIAN_POINT('Ctrl Pts',(3.48748281579126,-2.26542182682866,4.30726458363711));
#15501=CARTESIAN_POINT('Ctrl Pts',(3.45871387185408,-2.31121589220503,4.31089687545567));
#15502=CARTESIAN_POINT('Ctrl Pts',(3.44221012289161,-2.33748636499654,4.31298059575012));
#15503=CARTESIAN_POINT('Ctrl Pts',(3.43375001435867,-2.36880031414598,4.31506431604457));
#15504=CARTESIAN_POINT('Ctrl Pts',(3.43365449489478,-2.40006497081539,4.31714803633902));
#15505=CARTESIAN_POINT('',(3.4334,-2.4,4.2));
#15506=CARTESIAN_POINT('',(3.4334,-2.4,4.7));
#15507=CARTESIAN_POINT('Origin',(3.6,-2.4,4.2));
#15508=CARTESIAN_POINT('Ctrl Pts',(3.43365449489478,-2.40006497081539,4.31714803633902));
#15509=CARTESIAN_POINT('Ctrl Pts',(3.43358019259399,-2.42438499763772,4.31876891239684));
#15510=CARTESIAN_POINT('Ctrl Pts',(3.43856722876717,-2.44867519801865,4.32038978845465));
#15511=CARTESIAN_POINT('Ctrl Pts',(3.44876666940262,-2.4705384776482,4.32201066451247));
#15512=CARTESIAN_POINT('Ctrl Pts',(3.47207802031749,-2.52050813792769,4.32571526086474));
#15513=CARTESIAN_POINT('Ctrl Pts',(3.52261765592676,-2.55780017703868,4.329419857217));
#15514=CARTESIAN_POINT('Ctrl Pts',(3.57725038923478,-2.56532196913419,4.33312445356927));
#15515=CARTESIAN_POINT('Ctrl Pts',(3.6318831225428,-2.57284376122971,4.33682904992154));
#15516=CARTESIAN_POINT('Ctrl Pts',(3.69060895354956,-2.55059530630975,4.34053364627381));
#15517=CARTESIAN_POINT('Ctrl Pts',(3.72655438362155,-2.50877157126828,4.34423824262608));
#15518=CARTESIAN_POINT('Ctrl Pts',(3.76249981369354,-2.4669478362268,4.34794283897835));
#15519=CARTESIAN_POINT('Ctrl Pts',(3.77566484283074,-2.40554882106382,4.35164743533061));
#15520=CARTESIAN_POINT('Ctrl Pts',(3.76002306731497,-2.35266772394791,4.35535203168288));
#15521=CARTESIAN_POINT('Ctrl Pts',(3.74438129179919,-2.29978662683201,4.35905662803515));
#15522=CARTESIAN_POINT('Ctrl Pts',(3.69993271163044,-2.25542344776319,4.36276122438742));
#15523=CARTESIAN_POINT('Ctrl Pts',(3.64702014743753,-2.23988444780227,4.36646582073969));
#15524=CARTESIAN_POINT('Ctrl Pts',(3.59410758324462,-2.22434544784136,4.37017041709196));
#15525=CARTESIAN_POINT('Ctrl Pts',(3.53273103502755,-2.23763062698835,4.37387501344422));
#15526=CARTESIAN_POINT('Ctrl Pts',(3.49097949059372,-2.27365834937589,4.37757960979649));
#15527=CARTESIAN_POINT('Ctrl Pts',(3.45503346139427,-2.30467644890953,4.38076908531067));
#15528=CARTESIAN_POINT('Ctrl Pts',(3.43363419992272,-2.35255214998637,4.38395856082484));
#15529=CARTESIAN_POINT('Ctrl Pts',(3.4332441194689,-2.40012144310043,4.38714803633902));
#15530=CARTESIAN_POINT('Origin',(3.6,-2.4,4.7));
#15531=CARTESIAN_POINT('',(3.4332753032246,-2.39986752249821,4.45714803633902));
#15532=CARTESIAN_POINT('',(3.43362893615635,-2.39991676750829,4.43785196366098));
#15533=CARTESIAN_POINT('',(3.4334,-2.4,4.7));
#15534=CARTESIAN_POINT('Ctrl Pts',(3.43362893615635,-2.39991676750829,4.43785196366098));
#15535=CARTESIAN_POINT('Ctrl Pts',(3.43352745251214,-2.37748041857078,4.43635646533454));
#15536=CARTESIAN_POINT('Ctrl Pts',(3.43774838897563,-2.35508066415019,4.43486096700809));
#15537=CARTESIAN_POINT('Ctrl Pts',(3.44647311482898,-2.33459946287839,4.43336546868165));
#15538=CARTESIAN_POINT('Ctrl Pts',(3.46808570175023,-2.28386414463698,4.42966087232938));
#15539=CARTESIAN_POINT('Ctrl Pts',(3.51733510423541,-2.24490173470295,4.42595627597711));
#15540=CARTESIAN_POINT('Ctrl Pts',(3.57168220229163,-2.23554374099052,4.42225167962485));
#15541=CARTESIAN_POINT('Ctrl Pts',(3.62602930034785,-2.22618574727809,4.41854708327258));
#15542=CARTESIAN_POINT('Ctrl Pts',(3.68547409397512,-2.24643216978725,4.41484248692031));
#15543=CARTESIAN_POINT('Ctrl Pts',(3.72281103935986,-2.2870168380163,4.41113789056804));
#15544=CARTESIAN_POINT('Ctrl Pts',(3.7601479847446,-2.32760150624535,4.40743329421577));
#15545=CARTESIAN_POINT('Ctrl Pts',(3.77537708188681,-2.38852442019428,4.4037286978635));
#15546=CARTESIAN_POINT('Ctrl Pts',(3.76152924259544,-2.44190442427593,4.40002410151124));
#15547=CARTESIAN_POINT('Ctrl Pts',(3.74768140330407,-2.49528442835759,4.39631950515897));
#15548=CARTESIAN_POINT('Ctrl Pts',(3.70475662757912,-2.54112152257198,4.3926149088067));
#15549=CARTESIAN_POINT('Ctrl Pts',(3.65239849228647,-2.55843697682615,4.38891031245443));
#15550=CARTESIAN_POINT('Ctrl Pts',(3.60004035699382,-2.57575243108032,4.38520571610217));
#15551=CARTESIAN_POINT('Ctrl Pts',(3.53824886213347,-2.56454624537428,4.3815011197499));
#15552=CARTESIAN_POINT('Ctrl Pts',(3.49530561841154,-2.52994924443839,4.37779652339763));
#15553=CARTESIAN_POINT('Ctrl Pts',(3.45688023078761,-2.49899203076829,4.37448167015208));
#15554=CARTESIAN_POINT('Ctrl Pts',(3.43354583842081,-2.4493067834413,4.37116681690653));
#15555=CARTESIAN_POINT('Ctrl Pts',(3.43319918361158,-2.39990306414324,4.36785196366098));
#15556=CARTESIAN_POINT('Ctrl Pts',(3.4332441194689,-2.40012144310043,4.38714803633902));
#15557=CARTESIAN_POINT('Ctrl Pts',(3.4331811189632,-2.40780419031934,4.38766315717711));
#15558=CARTESIAN_POINT('Ctrl Pts',(3.43366612887655,-2.41547894509172,4.3881782780152));
#15559=CARTESIAN_POINT('Ctrl Pts',(3.43472637398198,-2.42307339909524,4.3886933988533));
#15560=CARTESIAN_POINT('Ctrl Pts',(3.44235134245467,-2.47769046079897,4.39239799520556));
#15561=CARTESIAN_POINT('Ctrl Pts',(3.47972782005064,-2.52815431857834,4.39610259155783));
#15562=CARTESIAN_POINT('Ctrl Pts',(3.5297501656918,-2.5513695031952,4.3998071879101));
#15563=CARTESIAN_POINT('Ctrl Pts',(3.57977251133296,-2.57458468781207,4.40351178426237));
#15564=CARTESIAN_POINT('Ctrl Pts',(3.64244072501932,-2.57055119926642,4.40721638061463));
#15565=CARTESIAN_POINT('Ctrl Pts',(3.68907438543537,-2.54111518550135,4.4109209769669));
#15566=CARTESIAN_POINT('Ctrl Pts',(3.73570804585142,-2.51167917173628,4.41462557331917));
#15567=CARTESIAN_POINT('Ctrl Pts',(3.76630715299715,-2.4568406327518,4.41833016967144));
#15568=CARTESIAN_POINT('Ctrl Pts',(3.76686783098938,-2.40169663747488,4.42203476602371));
#15569=CARTESIAN_POINT('Ctrl Pts',(3.7674285089816,-2.34655264219797,4.42573936237597));
#15570=CARTESIAN_POINT('Ctrl Pts',(3.73795075782031,-2.29110319062863,4.42944395872824));
#15571=CARTESIAN_POINT('Ctrl Pts',(3.69192524795617,-2.26072508833266,4.43314855508051));
#15572=CARTESIAN_POINT('Ctrl Pts',(3.64589973809204,-2.23034698603669,4.43685315143278));
#15573=CARTESIAN_POINT('Ctrl Pts',(3.58332646952505,-2.2250402330141,4.44055774778505));
#15574=CARTESIAN_POINT('Ctrl Pts',(3.53284244819528,-2.24723347009038,4.44426234413732));
#15575=CARTESIAN_POINT('Ctrl Pts',(3.48235842686551,-2.26942670716666,4.44796694048958));
#15576=CARTESIAN_POINT('Ctrl Pts',(3.44396365277294,-2.31911993434182,4.45167153684185));
#15577=CARTESIAN_POINT('Ctrl Pts',(3.43522971460805,-2.37357077679719,4.45537613319412));
#15578=CARTESIAN_POINT('Ctrl Pts',(3.43383723789082,-2.38225203019296,4.45596676757575));
#15579=CARTESIAN_POINT('Ctrl Pts',(3.4331987050974,-2.39105421663124,4.45655740195739));
#15580=CARTESIAN_POINT('Ctrl Pts',(3.4332753032246,-2.39986752249821,4.45714803633902));
#15581=CARTESIAN_POINT('Origin',(3.6,-2.4,4.7));
#15582=CARTESIAN_POINT('',(3.43366207720083,-2.39996197521424,4.52714803633902));
#15583=CARTESIAN_POINT('',(3.43350143827108,-2.40014312936039,4.50785196366098));
#15584=CARTESIAN_POINT('',(3.4334,-2.4,4.7));
#15585=CARTESIAN_POINT('Ctrl Pts',(3.43350143827108,-2.40014312936039,4.50785196366098));
#15586=CARTESIAN_POINT('Ctrl Pts',(3.43382055454292,-2.36119271753362,4.50525071011481));
#15587=CARTESIAN_POINT('Ctrl Pts',(3.44745634567654,-2.3220410177822,4.50264945656865));
#15588=CARTESIAN_POINT('Ctrl Pts',(3.4724157519356,-2.29243605104842,4.50004820302248));
#15589=CARTESIAN_POINT('Ctrl Pts',(3.50796189295608,-2.25027389736965,4.49634360667021));
#15590=CARTESIAN_POINT('Ctrl Pts',(3.56647488846456,-2.22747467908062,4.49263901031794));
#15591=CARTESIAN_POINT('Ctrl Pts',(3.62117593657879,-2.23447258988711,4.48893441396567));
#15592=CARTESIAN_POINT('Ctrl Pts',(3.67587698469302,-2.2414705006936,4.4852298176134));
#15593=CARTESIAN_POINT('Ctrl Pts',(3.726766085413,-2.27826554059562,4.48152522126114));
#15594=CARTESIAN_POINT('Ctrl Pts',(3.75055354862185,-2.32801824658462,4.47782062490887));
#15595=CARTESIAN_POINT('Ctrl Pts',(3.7743410118307,-2.37777095257363,4.4741160285566));
#15596=CARTESIAN_POINT('Ctrl Pts',(3.77102683752841,-2.44048132464963,4.47041143220433));
#15597=CARTESIAN_POINT('Ctrl Pts',(3.74212778560952,-2.48744961415947,4.46670683585206));
#15598=CARTESIAN_POINT('Ctrl Pts',(3.71322873369063,-2.53441790366931,4.4630022394998));
#15599=CARTESIAN_POINT('Ctrl Pts',(3.65874480415513,-2.56564411061299,4.45929764314753));
#15600=CARTESIAN_POINT('Ctrl Pts',(3.60361085781629,-2.56683736686161,4.45559304679526));
#15601=CARTESIAN_POINT('Ctrl Pts',(3.54847691147744,-2.56803062311024,4.45188845044299));
#15602=CARTESIAN_POINT('Ctrl Pts',(3.49269294833524,-2.5391909286638,4.44818385409072));
#15603=CARTESIAN_POINT('Ctrl Pts',(3.46178885244281,-2.49351696816619,4.44447925773846));
#15604=CARTESIAN_POINT('Ctrl Pts',(3.44336034614035,-2.46628100333426,4.44227015971263));
#15605=CARTESIAN_POINT('Ctrl Pts',(3.43377884425998,-2.43305896049386,4.4400610616868));
#15606=CARTESIAN_POINT('Ctrl Pts',(3.43362893615635,-2.39991676750829,4.43785196366098));
#15607=CARTESIAN_POINT('Ctrl Pts',(3.4332753032246,-2.39986752249821,4.45714803633902));
#15608=CARTESIAN_POINT('Ctrl Pts',(3.43367914638464,-2.44633332293026,4.46026199830965));
#15609=CARTESIAN_POINT('Ctrl Pts',(3.45396108248041,-2.49310820388228,4.46337596028029));
#15610=CARTESIAN_POINT('Ctrl Pts',(3.48843309316639,-2.52409905740531,4.46648992225092));
#15611=CARTESIAN_POINT('Ctrl Pts',(3.52944351212684,-2.56096803782247,4.47019451860319));
#15612=CARTESIAN_POINT('Ctrl Pts',(3.59053745228497,-2.57549754092119,4.47389911495546));
#15613=CARTESIAN_POINT('Ctrl Pts',(3.64375492615303,-2.56103806030718,4.47760371130773));
#15614=CARTESIAN_POINT('Ctrl Pts',(3.69697240002109,-2.54657857969317,4.48130830766));
#15615=CARTESIAN_POINT('Ctrl Pts',(3.74231340759908,-2.50313011536643,4.48501290401227));
#15616=CARTESIAN_POINT('Ctrl Pts',(3.75902737934242,-2.45057710185421,4.48871750036453));
#15617=CARTESIAN_POINT('Ctrl Pts',(3.77574135108577,-2.39802408834199,4.4924220967168));
#15618=CARTESIAN_POINT('Ctrl Pts',(3.76382828699448,-2.33636652564429,4.49612669306907));
#15619=CARTESIAN_POINT('Ctrl Pts',(3.72874026856414,-2.29382234772163,4.49983128942134));
#15620=CARTESIAN_POINT('Ctrl Pts',(3.6936522501338,-2.25127816979896,4.5035358857736));
#15621=CARTESIAN_POINT('Ctrl Pts',(3.63538927736442,-2.22784737665133,4.50724048212587));
#15622=CARTESIAN_POINT('Ctrl Pts',(3.58061573003626,-2.23425320323999,4.51094507847814));
#15623=CARTESIAN_POINT('Ctrl Pts',(3.52584218270809,-2.24065902982864,4.51464967483041));
#15624=CARTESIAN_POINT('Ctrl Pts',(3.47455806082114,-2.27690147615359,4.51835427118267));
#15625=CARTESIAN_POINT('Ctrl Pts',(3.45023383359826,-2.32639398133752,4.52205886753494));
#15626=CARTESIAN_POINT('Ctrl Pts',(3.43909540927391,-2.34905733333477,4.5237552571363));
#15627=CARTESIAN_POINT('Ctrl Pts',(3.4336100971438,-2.37449903703717,4.52545164673766));
#15628=CARTESIAN_POINT('Ctrl Pts',(3.43366207720083,-2.39996197521424,4.52714803633902));
#15629=CARTESIAN_POINT('Origin',(3.6,-2.4,4.7));
#15630=CARTESIAN_POINT('',(3.43341475097665,-2.4001523433056,4.59714803633902));
#15631=CARTESIAN_POINT('',(3.43312356989615,-2.39999932887968,4.57785196366098));
#15632=CARTESIAN_POINT('',(3.4334,-2.4,4.7));
#15633=CARTESIAN_POINT('Ctrl Pts',(3.4331235712606,-2.39999932888299,4.57785196366098));
#15634=CARTESIAN_POINT('Ctrl Pts',(3.43312027533203,-2.34481656196242,4.57414495489509));
#15635=CARTESIAN_POINT('Ctrl Pts',(3.46320503039949,-2.28963688420389,4.57043794612919));
#15636=CARTESIAN_POINT('Ctrl Pts',(3.50958660961886,-2.25973894891049,4.5667309373633));
#15637=CARTESIAN_POINT('Ctrl Pts',(3.55593800505376,-2.22986047032491,4.56302634101103));
#15638=CARTESIAN_POINT('Ctrl Pts',(3.61856500889817,-2.22523083965654,4.55932174465877));
#15639=CARTESIAN_POINT('Ctrl Pts',(3.66880601775922,-2.24796883366633,4.5556171483065));
#15640=CARTESIAN_POINT('Ctrl Pts',(3.71904702662027,-2.27070682767613,4.55191255195423));
#15641=CARTESIAN_POINT('Ctrl Pts',(3.75690204049796,-2.32081244636408,4.54820795560196));
#15642=CARTESIAN_POINT('Ctrl Pts',(3.765046497567,-2.37535456915184,4.54450335924969));
#15643=CARTESIAN_POINT('Ctrl Pts',(3.77319095463605,-2.4298966919396,4.54079876289742));
#15644=CARTESIAN_POINT('Ctrl Pts',(3.75162485489646,-2.48887531882715,4.53709416654515));
#15645=CARTESIAN_POINT('Ctrl Pts',(3.71021804632554,-2.52529854692327,4.53338957019289));
#15646=CARTESIAN_POINT('Ctrl Pts',(3.66881123775463,-2.56172177501939,4.52968497384062));
#15647=CARTESIAN_POINT('Ctrl Pts',(3.60756372035239,-2.57558960432407,4.52598037748835));
#15648=CARTESIAN_POINT('Ctrl Pts',(3.55450576746795,-2.56055534384899,4.52227578113609));
#15649=CARTESIAN_POINT('Ctrl Pts',(3.5014478145835,-2.5455210833739,4.51857118478382));
#15650=CARTESIAN_POINT('Ctrl Pts',(3.45657942621685,-2.50158473311904,4.51486658843155));
#15651=CARTESIAN_POINT('Ctrl Pts',(3.44043487529976,-2.44885401345736,4.51116199207928));
#15652=CARTESIAN_POINT('Ctrl Pts',(3.43562653117309,-2.43314918230523,4.51005864927318));
#15653=CARTESIAN_POINT('Ctrl Pts',(3.43336608251409,-2.41666426269897,4.50895530646708));
#15654=CARTESIAN_POINT('Ctrl Pts',(3.43350143827108,-2.40014312936039,4.50785196366098));
#15655=CARTESIAN_POINT('Ctrl Pts',(3.43366207720083,-2.39996197521424,4.52714803633902));
#15656=CARTESIAN_POINT('Ctrl Pts',(3.43372361182786,-2.43010531274957,4.52915624308993));
#15657=CARTESIAN_POINT('Ctrl Pts',(3.4415451707818,-2.46027840851952,4.53116444984084));
#15658=CARTESIAN_POINT('Ctrl Pts',(3.45693460775185,-2.48590718316162,4.53317265659175));
#15659=CARTESIAN_POINT('Ctrl Pts',(3.48532394168714,-2.53318531575888,4.53687725294402));
#15660=CARTESIAN_POINT('Ctrl Pts',(3.53946694211655,-2.5649990169105,4.54058184929628));
#15661=CARTESIAN_POINT('Ctrl Pts',(3.59458475789197,-2.56678856593634,4.54428644564855));
#15662=CARTESIAN_POINT('Ctrl Pts',(3.64970257366739,-2.56857811496219,4.54799104200082));
#15663=CARTESIAN_POINT('Ctrl Pts',(3.70579520478882,-2.54034351186226,4.55169563835309));
#15664=CARTESIAN_POINT('Ctrl Pts',(3.73719154055164,-2.49500648282243,4.55540023470536));
#15665=CARTESIAN_POINT('Ctrl Pts',(3.76858787631446,-2.4496694537826,4.55910483105763));
#15666=CARTESIAN_POINT('Ctrl Pts',(3.77528791671867,-2.38722999880286,4.56280942740989));
#15667=CARTESIAN_POINT('Ctrl Pts',(3.75422535028399,-2.33626388852243,4.56651402376216));
#15668=CARTESIAN_POINT('Ctrl Pts',(3.73316278384931,-2.28529777824199,4.57021862011443));
#15669=CARTESIAN_POINT('Ctrl Pts',(3.68433761057573,-2.24580501266085,4.5739232164667));
#15670=CARTESIAN_POINT('Ctrl Pts',(3.63009494786823,-2.23585967988047,4.57762781281896));
#15671=CARTESIAN_POINT('Ctrl Pts',(3.57585228516072,-2.22591434710008,4.58133240917123));
#15672=CARTESIAN_POINT('Ctrl Pts',(3.51619213301928,-2.24551644712046,4.5850370055235));
#15673=CARTESIAN_POINT('Ctrl Pts',(3.47841829836813,-2.28569496771878,4.58874160187577));
#15674=CARTESIAN_POINT('Ctrl Pts',(3.4498462907659,-2.31608587207317,4.59154374669685));
#15675=CARTESIAN_POINT('Ctrl Pts',(3.43379623586762,-2.35824928979842,4.59434589151794));
#15676=CARTESIAN_POINT('Ctrl Pts',(3.43341475097665,-2.4001523433056,4.59714803633902));
#15677=CARTESIAN_POINT('Origin',(3.6,-2.4,4.7));
#15678=CARTESIAN_POINT('',(3.43314572405529,-2.39994496470472,4.66714803633902));
#15679=CARTESIAN_POINT('',(3.43350339621029,-2.39985729254273,4.64785196366098));
#15680=CARTESIAN_POINT('',(3.4334,-2.4,4.7));
#15681=CARTESIAN_POINT('Ctrl Pts',(3.43350339621029,-2.39985729254273,4.64785196366098));
#15682=CARTESIAN_POINT('Ctrl Pts',(3.43336796571017,-2.38326341978069,4.64674379602763));
#15683=CARTESIAN_POINT('Ctrl Pts',(3.43564862259693,-2.36670593582693,4.64563562839428));
#15684=CARTESIAN_POINT('Ctrl Pts',(3.44049848254047,-2.3509387164529,4.64452746076093));
#15685=CARTESIAN_POINT('Ctrl Pts',(3.45671152911857,-2.29822901656582,4.64082286440866));
#15686=CARTESIAN_POINT('Ctrl Pts',(3.50163696254783,-2.25435099787568,4.6371182680564));
#15687=CARTESIAN_POINT('Ctrl Pts',(3.55471440347455,-2.23938568444105,4.63341367170413));
#15688=CARTESIAN_POINT('Ctrl Pts',(3.60779184440126,-2.22442037100641,4.62970907535186));
#15689=CARTESIAN_POINT('Ctrl Pts',(3.66902129282543,-2.23836776282728,4.62600447899959));
#15690=CARTESIAN_POINT('Ctrl Pts',(3.71038074448169,-2.27484475695027,4.62229988264732));
#15691=CARTESIAN_POINT('Ctrl Pts',(3.75174019613796,-2.31132175107326,4.61859528629505));
#15692=CARTESIAN_POINT('Ctrl Pts',(3.77322965102632,-2.37032834749837,4.61489068994278));
#15693=CARTESIAN_POINT('Ctrl Pts',(3.76501433826252,-2.42485984278043,4.61118609359052));
#15694=CARTESIAN_POINT('Ctrl Pts',(3.75679902549871,-2.47939133806249,4.60748149723825));
#15695=CARTESIAN_POINT('Ctrl Pts',(3.71887894508274,-2.52944773220152,4.60377690088598));
#15696=CARTESIAN_POINT('Ctrl Pts',(3.66860843684067,-2.55212043258282,4.60007230453372));
#15697=CARTESIAN_POINT('Ctrl Pts',(3.6183379285986,-2.57479313296412,4.59636770818145));
#15698=CARTESIAN_POINT('Ctrl Pts',(3.55571699253044,-2.5700821395877,4.59266311182918));
#15699=CARTESIAN_POINT('Ctrl Pts',(3.50940445510819,-2.54014346528121,4.58895851547691));
#15700=CARTESIAN_POINT('Ctrl Pts',(3.46312207616628,-2.51022428688169,4.58525633153827));
#15701=CARTESIAN_POINT('Ctrl Pts',(3.43312686289939,-2.45511027311999,4.58155414759963));
#15702=CARTESIAN_POINT('Ctrl Pts',(3.4331235712606,-2.39999932888299,4.57785196366098));
#15703=CARTESIAN_POINT('Ctrl Pts',(3.43341475097665,-2.4001523433056,4.59714803633902));
#15704=CARTESIAN_POINT('Ctrl Pts',(3.43329189093694,-2.41364753260286,4.5980504878702));
#15705=CARTESIAN_POINT('Ctrl Pts',(3.43479419036014,-2.42711571666781,4.59895293940139));
#15706=CARTESIAN_POINT('Ctrl Pts',(3.43802675920227,-2.44015494791281,4.59985539093257));
#15707=CARTESIAN_POINT('Ctrl Pts',(3.45129657184842,-2.49368146633226,4.60355998728484));
#15708=CARTESIAN_POINT('Ctrl Pts',(3.49372371430156,-2.53997956199491,4.60726458363711));
#15709=CARTESIAN_POINT('Ctrl Pts',(3.54589116423991,-2.55786064889342,4.61096917998938));
#15710=CARTESIAN_POINT('Ctrl Pts',(3.59805861417826,-2.57574173579194,4.61467377634165));
#15711=CARTESIAN_POINT('Ctrl Pts',(3.65996637160182,-2.56520581392632,4.61837837269391));
#15712=CARTESIAN_POINT('Ctrl Pts',(3.70328200028476,-2.53107470768073,4.62208296904618));
#15713=CARTESIAN_POINT('Ctrl Pts',(3.74659762896771,-2.49694360143515,4.62578756539845));
#15714=CARTESIAN_POINT('Ctrl Pts',(3.77132112891003,-2.43921731080961,4.62949216175072));
#15715=CARTESIAN_POINT('Ctrl Pts',(3.76613765017139,-2.3843146000394,4.63319675810299));
#15716=CARTESIAN_POINT('Ctrl Pts',(3.76095417143275,-2.32941188926919,4.63690135445526));
#15717=CARTESIAN_POINT('Ctrl Pts',(3.72586371401314,-2.27733275835431,4.64060595080752));
#15718=CARTESIAN_POINT('Ctrl Pts',(3.67692562472706,-2.25191151686662,4.64431054715979));
#15719=CARTESIAN_POINT('Ctrl Pts',(3.62798753544098,-2.22649027537894,4.64801514351206));
#15720=CARTESIAN_POINT('Ctrl Pts',(3.56520181428843,-2.22772692331845,4.65171973986433));
#15721=CARTESIAN_POINT('Ctrl Pts',(3.51730270257413,-2.25505550174341,4.6554243362166));
#15722=CARTESIAN_POINT('Ctrl Pts',(3.46940359085983,-2.28238408016837,4.65912893256887));
#15723=CARTESIAN_POINT('Ctrl Pts',(3.43639108858378,-2.33580458907878,4.66283352892113));
#15724=CARTESIAN_POINT('Ctrl Pts',(3.43337355460624,-2.39086882965689,4.6665381252734));
#15725=CARTESIAN_POINT('Ctrl Pts',(3.43320795605525,-2.39389068741188,4.66674142896194));
#15726=CARTESIAN_POINT('Ctrl Pts',(3.43313269272996,-2.39691749555954,4.66694473265048));
#15727=CARTESIAN_POINT('Ctrl Pts',(3.43314572405529,-2.39994496470472,4.66714803633902));
#15728=CARTESIAN_POINT('Origin',(3.6,-2.4,4.7));
#15729=CARTESIAN_POINT('',(3.43357723227316,-2.39988235337877,4.73714803633902));
#15730=CARTESIAN_POINT('',(3.43362781745768,-2.40008425136911,4.71785196366098));
#15731=CARTESIAN_POINT('',(3.4334,-2.4,4.7));
#15732=CARTESIAN_POINT('Ctrl Pts',(3.43362781745768,-2.40008425136911,4.71785196366098));
#15733=CARTESIAN_POINT('Ctrl Pts',(3.43377992278221,-2.36687021363152,4.7156380408079));
#15734=CARTESIAN_POINT('Ctrl Pts',(3.44340627006936,-2.33357497132763,4.71342411795483));
#15735=CARTESIAN_POINT('Ctrl Pts',(3.46191047910031,-2.30630353350919,4.71121019510175));
#15736=CARTESIAN_POINT('Ctrl Pts',(3.49287390006255,-2.260669753216,4.70750559874949));
#15737=CARTESIAN_POINT('Ctrl Pts',(3.54869526474406,-2.23190257855334,4.70380100239722));
#15738=CARTESIAN_POINT('Ctrl Pts',(3.60382760906969,-2.23316747012655,4.70009640604495));
#15739=CARTESIAN_POINT('Ctrl Pts',(3.65895995339532,-2.23443236169976,4.69639180969269));
#15740=CARTESIAN_POINT('Ctrl Pts',(3.71340327736507,-2.26572931950883,4.69268721334041));
#15741=CARTESIAN_POINT('Ctrl Pts',(3.74224128504954,-2.31273511334664,4.68898261698815));
#15742=CARTESIAN_POINT('Ctrl Pts',(3.77107929273401,-2.35974090718445,4.68527802063588));
#15743=CARTESIAN_POINT('Ctrl Pts',(3.7743119841332,-2.42245553705099,4.68157342428361));
#15744=CARTESIAN_POINT('Ctrl Pts',(3.75045989969766,-2.47217729697168,4.67786882793135));
#15745=CARTESIAN_POINT('Ctrl Pts',(3.72660781526212,-2.52189905689238,4.67416423157908));
#15746=CARTESIAN_POINT('Ctrl Pts',(3.67567095499184,-2.55862794686723,4.67045963522681));
#15747=CARTESIAN_POINT('Ctrl Pts',(3.62096086182118,-2.56555478213231,4.66675503887454));
#15748=CARTESIAN_POINT('Ctrl Pts',(3.56625076865053,-2.57248161739739,4.66305044252227));
#15749=CARTESIAN_POINT('Ctrl Pts',(3.50776744257951,-2.54960639795269,4.65934584617));
#15750=CARTESIAN_POINT('Ctrl Pts',(3.47227610940747,-2.50739809768834,4.65564124981773));
#15751=CARTESIAN_POINT('Ctrl Pts',(3.44740141107113,-2.47781569988784,4.65304482109882));
#15752=CARTESIAN_POINT('Ctrl Pts',(3.43382070888877,-2.43873661594181,4.6504483923799));
#15753=CARTESIAN_POINT('Ctrl Pts',(3.43350339621029,-2.39985729254273,4.64785196366098));
#15754=CARTESIAN_POINT('Ctrl Pts',(3.43314572405529,-2.39994496470472,4.66714803633902));
#15755=CARTESIAN_POINT('Ctrl Pts',(3.43337014931821,-2.45208398679426,4.67064932900275));
#15756=CARTESIAN_POINT('Ctrl Pts',(3.45978247638053,-2.50441905856693,4.67415062166648));
#15757=CARTESIAN_POINT('Ctrl Pts',(3.50195948177967,-2.53504002133992,4.67765191433021));
#15758=CARTESIAN_POINT('Ctrl Pts',(3.54658550860969,-2.56743900019905,4.68135651068247));
#15759=CARTESIAN_POINT('Ctrl Pts',(3.60886012794877,-2.57552898567153,4.68506110703474));
#15760=CARTESIAN_POINT('Ctrl Pts',(3.66028300713527,-2.55560755003253,4.68876570338701));
#15761=CARTESIAN_POINT('Ctrl Pts',(3.71170588632177,-2.53568611439352,4.69247029973927));
#15762=CARTESIAN_POINT('Ctrl Pts',(3.7522770253557,-2.48775325764304,4.69617489609154));
#15763=CARTESIAN_POINT('Ctrl Pts',(3.76342881240416,-2.43374572347072,4.69987949244381));
#15764=CARTESIAN_POINT('Ctrl Pts',(3.77458059945262,-2.3797381892984,4.70358408879608));
#15765=CARTESIAN_POINT('Ctrl Pts',(3.75631303451563,-2.31965597770425,4.70728868514835));
#15766=CARTESIAN_POINT('Ctrl Pts',(3.71698637227073,-2.28099605351363,4.71099328150061));
#15767=CARTESIAN_POINT('Ctrl Pts',(3.67765971002583,-2.24233612932302,4.71469787785288));
#15768=CARTESIAN_POINT('Ctrl Pts',(3.61727395047302,-2.22509849253594,4.71840247420515));
#15769=CARTESIAN_POINT('Ctrl Pts',(3.5634649788822,-2.23717204537206,4.72210707055742));
#15770=CARTESIAN_POINT('Ctrl Pts',(3.50965600729138,-2.24924559820818,4.72581166690969));
#15771=CARTESIAN_POINT('Ctrl Pts',(3.46242382366254,-2.29063034066749,4.72951626326196));
#15772=CARTESIAN_POINT('Ctrl Pts',(3.44338450465812,-2.34238631069604,4.73322085961423));
#15773=CARTESIAN_POINT('Ctrl Pts',(3.43665675680651,-2.36067483856233,4.73452991852249));
#15774=CARTESIAN_POINT('Ctrl Pts',(3.43344927751834,-2.38025835744364,4.73583897743076));
#15775=CARTESIAN_POINT('Ctrl Pts',(3.43357723227316,-2.39988235337877,4.73714803633902));
#15776=CARTESIAN_POINT('Origin',(3.6,-2.4,4.7));
#15777=CARTESIAN_POINT('',(3.43357088161517,-2.40012064492246,4.80714803633902));
#15778=CARTESIAN_POINT('',(3.43319592655187,-2.40009747379871,4.78785196366098));
#15779=CARTESIAN_POINT('',(3.4334,-2.4,4.7));
#15780=CARTESIAN_POINT('Ctrl Pts',(3.43319592655187,-2.40009747379871,4.78785196366098));
#15781=CARTESIAN_POINT('Ctrl Pts',(3.43353982295269,-2.35062359307345,4.78453228558818));
#15782=CARTESIAN_POINT('Ctrl Pts',(3.45695304474081,-2.30086703036466,4.78121260751538));
#15783=CARTESIAN_POINT('Ctrl Pts',(3.49547520498793,-2.2699142173685,4.77789292944258));
#15784=CARTESIAN_POINT('Ctrl Pts',(3.53846402836278,-2.23537241072238,4.77418833309031));
#15785=CARTESIAN_POINT('Ctrl Pts',(3.6002686999986,-2.22424776884202,4.77048373673804));
#15786=CARTESIAN_POINT('Ctrl Pts',(3.65260396146494,-2.24163154716497,4.76677914038577));
#15787=CARTESIAN_POINT('Ctrl Pts',(3.70493922293128,-2.25901532548792,4.76307454403351));
#15788=CARTESIAN_POINT('Ctrl Pts',(3.74780507422814,-2.30490752401418,4.75936994768124));
#15789=CARTESIAN_POINT('Ctrl Pts',(3.7615837154436,-2.35830531786175,4.75566535132897));
#15790=CARTESIAN_POINT('Ctrl Pts',(3.77536235665906,-2.41170311170932,4.75196075497671));
#15791=CARTESIAN_POINT('Ctrl Pts',(3.76005378779311,-2.4726065008782,4.74825615862444));
#15792=CARTESIAN_POINT('Ctrl Pts',(3.72266406219276,-2.51314270396953,4.74455156227217));
#15793=CARTESIAN_POINT('Ctrl Pts',(3.68527433659241,-2.55367890706087,4.7408469659199));
#15794=CARTESIAN_POINT('Ctrl Pts',(3.62580345425764,-2.57384792407467,4.73714236956763));
#15795=CARTESIAN_POINT('Ctrl Pts',(3.57146860171181,-2.56441929000846,4.73343777321536));
#15796=CARTESIAN_POINT('Ctrl Pts',(3.51713374916598,-2.55499065594226,4.7297331768631));
#15797=CARTESIAN_POINT('Ctrl Pts',(3.46793492640908,-2.51596437079605,4.72602858051083));
#15798=CARTESIAN_POINT('Ctrl Pts',(3.4463882536521,-2.46520103526108,4.72232398415856));
#15799=CARTESIAN_POINT('Ctrl Pts',(3.43771819866623,-2.44477463739825,4.72083331065937));
#15800=CARTESIAN_POINT('Ctrl Pts',(3.43352540224658,-2.42244785170318,4.71934263716017));
#15801=CARTESIAN_POINT('Ctrl Pts',(3.43362781745768,-2.40008425136911,4.71785196366098));
#15802=CARTESIAN_POINT('Ctrl Pts',(3.43357723227316,-2.39988235337877,4.73714803633902));
#15803=CARTESIAN_POINT('Ctrl Pts',(3.43381138552965,-2.4357936609347,4.73954357378302));
#15804=CARTESIAN_POINT('Ctrl Pts',(3.44521519749436,-2.4718405175289,4.74193911122702));
#15805=CARTESIAN_POINT('Ctrl Pts',(3.46665596946098,-2.50033503922361,4.74433464867103));
#15806=CARTESIAN_POINT('Ctrl Pts',(3.49981320764826,-2.54440060012484,4.74803924502329));
#15807=CARTESIAN_POINT('Ctrl Pts',(3.55697413840284,-2.57040452432951,4.75174384137556));
#15808=CARTESIAN_POINT('Ctrl Pts',(3.61197873764036,-2.56644596847307,4.75544843772783));
#15809=CARTESIAN_POINT('Ctrl Pts',(3.66698333687788,-2.56248741261664,4.7591530340801));
#15810=CARTESIAN_POINT('Ctrl Pts',(3.71983160459833,-2.52856637669909,4.76285763043237));
#15811=CARTESIAN_POINT('Ctrl Pts',(3.7463372314094,-2.48020701515346,4.76656222678464));
#15812=CARTESIAN_POINT('Ctrl Pts',(3.77284285822047,-2.43184765360783,4.7702668231369));
#15813=CARTESIAN_POINT('Ctrl Pts',(3.77300584412214,-2.36904996643411,4.77397141948917));
#15814=CARTESIAN_POINT('Ctrl Pts',(3.74675159769234,-2.32055367125447,4.77767601584144));
#15815=CARTESIAN_POINT('Ctrl Pts',(3.72049735126253,-2.27205737607482,4.78138061219371));
#15816=CARTESIAN_POINT('Ctrl Pts',(3.66782587250124,-2.23786247288924,4.78508520854598));
#15817=CARTESIAN_POINT('Ctrl Pts',(3.61284256233116,-2.23361845303891,4.78878980489824));
#15818=CARTESIAN_POINT('Ctrl Pts',(3.55785925216109,-2.22937443318857,4.79249440125051));
#15819=CARTESIAN_POINT('Ctrl Pts',(3.50056411058224,-2.25508129667347,4.79619899760278));
#15820=CARTESIAN_POINT('Ctrl Pts',(3.46717858402372,-2.29897415165191,4.79990359395505));
#15821=CARTESIAN_POINT('Ctrl Pts',(3.44541647189655,-2.32758538921762,4.80231840808304));
#15822=CARTESIAN_POINT('Ctrl Pts',(3.43381352935432,-2.36392383491678,4.80473322221103));
#15823=CARTESIAN_POINT('Ctrl Pts',(3.43357088161517,-2.40012064492246,4.80714803633902));
#15824=CARTESIAN_POINT('Origin',(3.6,-2.4,4.7));
#15825=CARTESIAN_POINT('',(3.43314189260959,-2.4000500574177,4.87714803633902));
#15826=CARTESIAN_POINT('',(3.43333250832843,-2.39985412494998,4.85785196366098));
#15827=CARTESIAN_POINT('',(3.4334,-2.4,4.7));
#15828=CARTESIAN_POINT('Ctrl Pts',(3.43333250832843,-2.39985412494998,4.85785196366098));
#15829=CARTESIAN_POINT('Ctrl Pts',(3.43323384369475,-2.3890884237173,4.85713112672072));
#15830=CARTESIAN_POINT('Ctrl Pts',(3.43418764919828,-2.37834013090661,4.85641028978047));
#15831=CARTESIAN_POINT('Ctrl Pts',(3.4362574396422,-2.36781122023692,4.85568945284021));
#15832=CARTESIAN_POINT('Ctrl Pts',(3.44689471098651,-2.31370000328629,4.85198485648794));
#15833=CARTESIAN_POINT('Ctrl Pts',(3.48700781310569,-2.26538319325753,4.84828026013567));
#15834=CARTESIAN_POINT('Ctrl Pts',(3.53823875735816,-2.24497325223528,4.8445756637834));
#15835=CARTESIAN_POINT('Ctrl Pts',(3.58946970161063,-2.22456331121304,4.84087106743114));
#15836=CARTESIAN_POINT('Ctrl Pts',(3.65181848799641,-2.23206023919731,4.83716647107887));
#15837=CARTESIAN_POINT('Ctrl Pts',(3.69675084088435,-2.26403302458561,4.8334618747266));
#15838=CARTESIAN_POINT('Ctrl Pts',(3.74168319377229,-2.2960058099739,4.82975727837434));
#15839=CARTESIAN_POINT('Ctrl Pts',(3.76919911316239,-2.35245445276622,4.82605268202207));
#15840=CARTESIAN_POINT('Ctrl Pts',(3.76670578251992,-2.40754491150309,4.8223480856698));
#15841=CARTESIAN_POINT('Ctrl Pts',(3.76421245187744,-2.46263537023996,4.81864348931753));
#15842=CARTESIAN_POINT('Ctrl Pts',(3.73170987120238,-2.51636764492139,4.81493889296526));
#15843=CARTESIAN_POINT('Ctrl Pts',(3.68407303084285,-2.54415085535669,4.81123429661299));
#15844=CARTESIAN_POINT('Ctrl Pts',(3.63643619048332,-2.57193406579199,4.80752970026073));
#15845=CARTESIAN_POINT('Ctrl Pts',(3.57366509043931,-2.57376821198116,4.80382510390846));
#15846=CARTESIAN_POINT('Ctrl Pts',(3.52448728058231,-2.54881388652042,4.80012050755619));
#15847=CARTESIAN_POINT('Ctrl Pts',(3.47530947072531,-2.52385956105968,4.79641591120392));
#15848=CARTESIAN_POINT('Ctrl Pts',(3.43972495105532,-2.47211676394902,4.79271131485165));
#15849=CARTESIAN_POINT('Ctrl Pts',(3.43401917877726,-2.41726587968776,4.78900671849938));
#15850=CARTESIAN_POINT('Ctrl Pts',(3.43342633252912,-2.41156671411356,4.78862180021992));
#15851=CARTESIAN_POINT('Ctrl Pts',(3.43315605159773,-2.40583399421718,4.78823688194045));
#15852=CARTESIAN_POINT('Ctrl Pts',(3.43319592655187,-2.40009747379871,4.78785196366098));
#15853=CARTESIAN_POINT('Ctrl Pts',(3.43357088161517,-2.40012064492246,4.80714803633902));
#15854=CARTESIAN_POINT('Ctrl Pts',(3.43344128044335,-2.4194538108087,4.8084378185633));
#15855=CARTESIAN_POINT('Ctrl Pts',(3.43655249964156,-2.4387465714195,4.80972760078758));
#15856=CARTESIAN_POINT('Ctrl Pts',(3.44308755405667,-2.45679995496896,4.81101738301185));
#15857=CARTESIAN_POINT('Ctrl Pts',(3.46185796218633,-2.50865405683559,4.81472197936412));
#15858=CARTESIAN_POINT('Ctrl Pts',(3.50887468998386,-2.55028341409687,4.81842657571639));
#15859=CARTESIAN_POINT('Ctrl Pts',(3.56262026536972,-2.56263611534763,4.82213117206866));
#15860=CARTESIAN_POINT('Ctrl Pts',(3.61636584075558,-2.5749888165984,4.82583576842092));
#15861=CARTESIAN_POINT('Ctrl Pts',(3.67684026372979,-2.55806486183865,4.82954036477319));
#15862=CARTESIAN_POINT('Ctrl Pts',(3.71636707170489,-2.51960959492959,4.83324496112546));
#15863=CARTESIAN_POINT('Ctrl Pts',(3.75589387967999,-2.48115432802054,4.83694955747773));
#15864=CARTESIAN_POINT('Ctrl Pts',(3.77447307265599,-2.42116774896216,4.84065415383));
#15865=CARTESIAN_POINT('Ctrl Pts',(3.76360177761623,-2.36710305580748,4.84435875018227));
#15866=CARTESIAN_POINT('Ctrl Pts',(3.75273048257646,-2.3130383626528,4.84806334653453));
#15867=CARTESIAN_POINT('Ctrl Pts',(3.71240869952093,-2.26489555540181,4.8517679428868));
#15868=CARTESIAN_POINT('Ctrl Pts',(3.66108992110507,-2.24470746278141,4.85547253923907));
#15869=CARTESIAN_POINT('Ctrl Pts',(3.60977114268922,-2.224519370161,4.85917713559134));
#15870=CARTESIAN_POINT('Ctrl Pts',(3.54745536891304,-2.23228599217118,4.86288173194361));
#15871=CARTESIAN_POINT('Ctrl Pts',(3.50266176699964,-2.26445289020885,4.86658632829587));
#15872=CARTESIAN_POINT('Ctrl Pts',(3.4600933015382,-2.29502188733407,4.87010689764359));
#15873=CARTESIAN_POINT('Ctrl Pts',(3.43334940736011,-2.34762718854044,4.87362746699131));
#15874=CARTESIAN_POINT('Ctrl Pts',(3.43314189260959,-2.4000500574177,4.87714803633902));
#15875=CARTESIAN_POINT('Origin',(3.6,-2.4,4.7));
#15876=CARTESIAN_POINT('',(3.43342339329134,-2.39984780956037,4.94714803633902));
#15877=CARTESIAN_POINT('',(3.43366987537036,-2.39999366746476,4.92785196366098));
#15878=CARTESIAN_POINT('',(3.4334,-2.4,4.7));
#15879=CARTESIAN_POINT('Ctrl Pts',(3.43366987537036,-2.39999366746476,4.92785196366098));
#15880=CARTESIAN_POINT('Ctrl Pts',(3.43366057869757,-2.37257318362641,4.926025371501));
#15881=CARTESIAN_POINT('Ctrl Pts',(3.44006468998231,-2.34515678783965,4.92419877934102));
#15882=CARTESIAN_POINT('Ctrl Pts',(3.45290605548974,-2.32118937188857,4.92237218718104));
#15883=CARTESIAN_POINT('Ctrl Pts',(3.47895022498703,-2.27257994300186,4.91866759082877));
#15884=CARTESIAN_POINT('Ctrl Pts',(3.53147325377826,-2.23815747156893,4.9149629944765));
#15885=CARTESIAN_POINT('Ctrl Pts',(3.58643767991325,-2.23367559683213,4.91125839812423));
#15886=CARTESIAN_POINT('Ctrl Pts',(3.64140210604824,-2.22919372209532,4.90755380177196));
#15887=CARTESIAN_POINT('Ctrl Pts',(3.69880792952698,-2.25465244405464,4.9038492054197));
#15888=CARTESIAN_POINT('Ctrl Pts',(3.7323830497203,-2.29840043424344,4.90014460906743));
#15889=CARTESIAN_POINT('Ctrl Pts',(3.76595816991362,-2.34214842443224,4.89644001271516));
#15890=CARTESIAN_POINT('Ctrl Pts',(3.77570258682152,-2.40418568285053,4.89273541636289));
#15891=CARTESIAN_POINT('Ctrl Pts',(3.75715671279198,-2.45612050640859,4.88903082001062));
#15892=CARTESIAN_POINT('Ctrl Pts',(3.73861083876244,-2.50805532996664,4.88532622365835));
#15893=CARTESIAN_POINT('Ctrl Pts',(3.69177467379546,-2.54988771866446,4.88162162730609));
#15894=CARTESIAN_POINT('Ctrl Pts',(3.63808305436706,-2.56247284260842,4.87791703095382));
#15895=CARTESIAN_POINT('Ctrl Pts',(3.58439143493865,-2.57505796655237,4.87421243460155));
#15896=CARTESIAN_POINT('Ctrl Pts',(3.52384436104883,-2.55839582574246,4.87050783824928));
#15897=CARTESIAN_POINT('Ctrl Pts',(3.48415154438863,-2.52011194340126,4.86680324189701));
#15898=CARTESIAN_POINT('Ctrl Pts',(3.45218211937245,-2.4892773035642,4.863819482485));
#15899=CARTESIAN_POINT('Ctrl Pts',(3.4337409107187,-2.4444165781012,4.86083572307299));
#15900=CARTESIAN_POINT('Ctrl Pts',(3.43333250832843,-2.39985412494998,4.85785196366098));
#15901=CARTESIAN_POINT('Ctrl Pts',(3.43314189260959,-2.4000500574177,4.87714803633902));
#15902=CARTESIAN_POINT('Ctrl Pts',(3.43313104541013,-2.4027903026953,4.87733206334358));
#15903=CARTESIAN_POINT('Ctrl Pts',(3.43319270505025,-2.40553004950279,4.87751609034813));
#15904=CARTESIAN_POINT('Ctrl Pts',(3.43332840145004,-2.40826612443654,4.87770011735268));
#15905=CARTESIAN_POINT('Ctrl Pts',(3.43606006786446,-2.46334528656136,4.88140471370495));
#15906=CARTESIAN_POINT('Ctrl Pts',(3.46879483074392,-2.51693643674581,4.88510931005721));
#15907=CARTESIAN_POINT('Ctrl Pts',(3.51655144023777,-2.54451328122398,4.88881390640948));
#15908=CARTESIAN_POINT('Ctrl Pts',(3.56430804973163,-2.57209012570216,4.89251850276175));
#15909=CARTESIAN_POINT('Ctrl Pts',(3.62708650583988,-2.57365266447405,4.89622309911402));
#15910=CARTESIAN_POINT('Ctrl Pts',(3.67615589214678,-2.54848579281353,4.89992769546629));
#15911=CARTESIAN_POINT('Ctrl Pts',(3.72522527845368,-2.52331892115301,4.90363229181856));
#15912=CARTESIAN_POINT('Ctrl Pts',(3.76058559495924,-2.47142263906009,4.90733688817082));
#15913=CARTESIAN_POINT('Ctrl Pts',(3.76605399230753,-2.41654757430046,4.91104148452309));
#15914=CARTESIAN_POINT('Ctrl Pts',(3.77152238965583,-2.36167250954082,4.91474608087536));
#15915=CARTESIAN_POINT('Ctrl Pts',(3.74709886784687,-2.30381866211447,4.91845067722763));
#15916=CARTESIAN_POINT('Ctrl Pts',(3.70396099012833,-2.26946317336186,4.9221552735799));
#15917=CARTESIAN_POINT('Ctrl Pts',(3.6608231124098,-2.23510768460924,4.92585986993216));
#15918=CARTESIAN_POINT('Ctrl Pts',(3.5989708787817,-2.22425055453036,4.92956446628443));
#15919=CARTESIAN_POINT('Ctrl Pts',(3.54671131468788,-2.24186061024559,4.9332690626367));
#15920=CARTESIAN_POINT('Ctrl Pts',(3.49445175059407,-2.25947066596082,4.93697365898896));
#15921=CARTESIAN_POINT('Ctrl Pts',(3.45178485603454,-2.30554790747016,4.94067825534124));
#15922=CARTESIAN_POINT('Ctrl Pts',(3.43823737724635,-2.35900482396987,4.94438285169351));
#15923=CARTESIAN_POINT('Ctrl Pts',(3.43486667440692,-2.37230526038685,4.94530457990868));
#15924=CARTESIAN_POINT('Ctrl Pts',(3.43329860172231,-2.38606253373953,4.94622630812385));
#15925=CARTESIAN_POINT('Ctrl Pts',(3.43342339329134,-2.39984780956037,4.94714803633902));
#15926=CARTESIAN_POINT('Origin',(3.6,-2.4,4.7));
#15927=CARTESIAN_POINT('',(3.43365998837939,-2.40004261214837,5.01714803633902));
#15928=CARTESIAN_POINT('',(3.4333557533513,-2.40014916294441,4.99785196366098));
#15929=CARTESIAN_POINT('',(3.4334,-2.4,4.7));
#15930=CARTESIAN_POINT('Ctrl Pts',(3.4333557533513,-2.40014916294441,4.99785196366098));
#15931=CARTESIAN_POINT('Ctrl Pts',(3.43376006878861,-2.35633883086337,4.99491961628128));
#15932=CARTESIAN_POINT('Ctrl Pts',(3.45150379646176,-2.31223873171809,4.99198726890157));
#15933=CARTESIAN_POINT('Ctrl Pts',(3.48249984549986,-2.28150334481789,4.98905492152186));
#15934=CARTESIAN_POINT('Ctrl Pts',(3.5216588656746,-2.24267363351424,4.98535032516959));
#15935=CARTESIAN_POINT('Ctrl Pts',(3.58196947066853,-2.22517489033693,4.98164572881732));
#15936=CARTESIAN_POINT('Ctrl Pts',(3.63583017024712,-2.23701551447795,4.97794113246505));
#15937=CARTESIAN_POINT('Ctrl Pts',(3.68969086982571,-2.24885613861896,4.97423653611278));
#15938=CARTESIAN_POINT('Ctrl Pts',(3.73710166398897,-2.29003613007831,4.97053193976052));
#15939=CARTESIAN_POINT('Ctrl Pts',(3.75636473388799,-2.34170923218213,4.96682734340825));
#15940=CARTESIAN_POINT('Ctrl Pts',(3.775627803787,-2.39338233428594,4.96312274705599));
#15941=CARTESIAN_POINT('Ctrl Pts',(3.76674314942177,-2.45554854703422,4.95941815070372));
#15942=CARTESIAN_POINT('Ctrl Pts',(3.73377688327324,-2.49975715069431,4.95571355435145));
#15943=CARTESIAN_POINT('Ctrl Pts',(3.7008106171247,-2.54396575435439,4.95200895799918));
#15944=CARTESIAN_POINT('Ctrl Pts',(3.64376273919286,-2.57021674892629,4.94830436164691));
#15945=CARTESIAN_POINT('Ctrl Pts',(3.58874153428106,-2.56649621787192,4.94459976529464));
#15946=CARTESIAN_POINT('Ctrl Pts',(3.53372032936927,-2.56277568681755,4.94089516894238));
#15947=CARTESIAN_POINT('Ctrl Pts',(3.48072579747752,-2.52908363013692,4.93719057259011));
#15948=CARTESIAN_POINT('Ctrl Pts',(3.45401118663332,-2.48083940862635,4.93348597623784));
#15949=CARTESIAN_POINT('Ctrl Pts',(3.4404685098097,-2.45638253353524,4.93160797204555));
#15950=CARTESIAN_POINT('Ctrl Pts',(3.43367943371122,-2.42818593979086,4.92972996785327));
#15951=CARTESIAN_POINT('Ctrl Pts',(3.43366987537036,-2.39999366746476,4.92785196366098));
#15952=CARTESIAN_POINT('Ctrl Pts',(3.43342339329134,-2.39984780956037,4.94714803633902));
#15953=CARTESIAN_POINT('Ctrl Pts',(3.43380016214308,-2.44146810957007,4.94993090447612));
#15954=CARTESIAN_POINT('Ctrl Pts',(3.44960819947038,-2.48334366548894,4.95271377261321));
#15955=CARTESIAN_POINT('Ctrl Pts',(3.47782660292827,-2.51367238728015,4.95549664075031));
#15956=CARTESIAN_POINT('Ctrl Pts',(3.51539137041525,-2.55404644260063,4.95920123710258));
#15957=CARTESIAN_POINT('Ctrl Pts',(3.57494896840608,-2.57395796175148,4.96290583345484));
#15958=CARTESIAN_POINT('Ctrl Pts',(3.62924252448225,-2.56429432528282,4.96661042980711));
#15959=CARTESIAN_POINT('Ctrl Pts',(3.68353608055842,-2.55463068881416,4.97031502615938));
#15960=CARTESIAN_POINT('Ctrl Pts',(3.73256559471993,-2.51539189672599,4.97401962251165));
#15961=CARTESIAN_POINT('Ctrl Pts',(3.75389243176138,-2.46453580432507,4.97772421886392));
#15962=CARTESIAN_POINT('Ctrl Pts',(3.77521926880282,-2.41367971192415,4.98142881521619));
#15963=CARTESIAN_POINT('Ctrl Pts',(3.7688434287242,-2.35120631921049,4.98513341156845));
#15964=CARTESIAN_POINT('Ctrl Pts',(3.73768285095733,-2.30570692939164,4.98883800792072));
#15965=CARTESIAN_POINT('Ctrl Pts',(3.70652227319045,-2.26020753957279,4.99254260427299));
#15966=CARTESIAN_POINT('Ctrl Pts',(3.65057695773533,-2.23168215264876,4.99624720062526));
#15967=CARTESIAN_POINT('Ctrl Pts',(3.59545059530862,-2.23318557212546,4.99995179697752));
#15968=CARTESIAN_POINT('Ctrl Pts',(3.5403242328819,-2.23468899160217,5.00365639332979));
#15969=CARTESIAN_POINT('Ctrl Pts',(3.48601682348359,-2.2662212174796,5.00736098968206));
#15970=CARTESIAN_POINT('Ctrl Pts',(3.4573824612349,-2.31335135092863,5.01106558603433));
#15971=CARTESIAN_POINT('Ctrl Pts',(3.44171120056098,-2.3391451367466,5.01309306946923));
#15972=CARTESIAN_POINT('Ctrl Pts',(3.43372965513495,-2.36961088327844,5.01512055290413));
#15973=CARTESIAN_POINT('Ctrl Pts',(3.43365998837939,-2.40004261214837,5.01714803633902));
#15974=CARTESIAN_POINT('Origin',(3.6,-2.4,4.7));
#15975=CARTESIAN_POINT('',(3.43326718206005,-2.40013003210005,5.08714803633902));
#15976=CARTESIAN_POINT('',(3.43317939237559,-2.39991359865598,5.06785196366098));
#15977=CARTESIAN_POINT('',(3.4334,-2.4,4.7));
#15978=CARTESIAN_POINT('Ctrl Pts',(3.43317939237559,-2.39991359865598,5.06785196366098));
#15979=CARTESIAN_POINT('Ctrl Pts',(3.43314802801357,-2.39494457971841,5.06751845741381));
#15980=CARTESIAN_POINT('Ctrl Pts',(3.43335080279482,-2.38997815623028,5.06718495116665));
#15981=CARTESIAN_POINT('Ctrl Pts',(3.43379605546717,-2.38503356765244,5.06685144491949));
#15982=CARTESIAN_POINT('Ctrl Pts',(3.43874193411214,-2.33010894490636,5.06314684856722));
#15983=CARTESIAN_POINT('Ctrl Pts',(3.47360673801625,-2.27787849376484,5.05944225221495));
#15984=CARTESIAN_POINT('Ctrl Pts',(3.52243437581894,-2.25224575672994,5.05573765586269));
#15985=CARTESIAN_POINT('Ctrl Pts',(3.57126201362163,-2.22661301969504,5.05203305951042));
#15986=CARTESIAN_POINT('Ctrl Pts',(3.63405248532289,-2.22757799676674,5.04832846315815));
#15987=CARTESIAN_POINT('Ctrl Pts',(3.68206938357278,-2.25469907052132,5.04462386680588));
#15988=CARTESIAN_POINT('Ctrl Pts',(3.73008628182266,-2.28182014427589,5.04091927045361));
#15989=CARTESIAN_POINT('Ctrl Pts',(3.76332960662116,-2.33509731471334,5.03721467410135));
#15990=CARTESIAN_POINT('Ctrl Pts',(3.7665853578407,-2.39014797778335,5.03351007774908));
#15991=CARTESIAN_POINT('Ctrl Pts',(3.76984110906023,-2.44519864085336,5.02980548139681));
#15992=CARTESIAN_POINT('Ctrl Pts',(3.7431092867008,-2.50202279655593,5.02610088504454));
#15993=CARTESIAN_POINT('Ctrl Pts',(3.69862386285843,-2.53461455026518,5.02239628869228));
#15994=CARTESIAN_POINT('Ctrl Pts',(3.65413843901607,-2.56720630397444,5.01869169234001));
#15995=CARTESIAN_POINT('Ctrl Pts',(3.59189941369078,-2.57556565569037,5.01498709598774));
#15996=CARTESIAN_POINT('Ctrl Pts',(3.54039082873623,-2.55586689947754,5.01128249963547));
#15997=CARTESIAN_POINT('Ctrl Pts',(3.48888224378167,-2.53616814326471,5.0075779032832));
#15998=CARTESIAN_POINT('Ctrl Pts',(3.44810409919785,-2.48841127912311,5.00387330693093));
#15999=CARTESIAN_POINT('Ctrl Pts',(3.43671874458371,-2.43445250733732,5.00016871057866));
#16000=CARTESIAN_POINT('Ctrl Pts',(3.43434538792972,-2.42320442465572,4.9993964616061));
#16001=CARTESIAN_POINT('Ctrl Pts',(3.43324927477267,-2.41168684233781,4.99862421263354));
#16002=CARTESIAN_POINT('Ctrl Pts',(3.4333557533513,-2.40014916294441,4.99785196366098));
#16003=CARTESIAN_POINT('Ctrl Pts',(3.43365998837939,-2.40004261214837,5.01714803633902));
#16004=CARTESIAN_POINT('Ctrl Pts',(3.43360236077384,-2.42521541736454,5.01882514925639));
#16005=CARTESIAN_POINT('Ctrl Pts',(3.43895837597341,-2.45036494625428,5.02050226217376));
#16006=CARTESIAN_POINT('Ctrl Pts',(3.44985377805168,-2.47282762403026,5.02217937509113));
#16007=CARTESIAN_POINT('Ctrl Pts',(3.47392077221621,-2.52244572266223,5.0258839714434));
#16008=CARTESIAN_POINT('Ctrl Pts',(3.52501607564434,-2.55895387890556,5.02958856779567));
#16009=CARTESIAN_POINT('Ctrl Pts',(3.57975563405926,-2.56564394064586,5.03329316414793));
#16010=CARTESIAN_POINT('Ctrl Pts',(3.63449519247418,-2.57233400238615,5.0369977605002));
#16011=CARTESIAN_POINT('Ctrl Pts',(3.69287900587587,-2.54920596962341,5.04070235685248));
#16012=CARTESIAN_POINT('Ctrl Pts',(3.72818738886538,-2.5068444924534,5.04440695320474));
#16013=CARTESIAN_POINT('Ctrl Pts',(3.76349577185488,-2.4644830152834,5.04811154955701));
#16014=CARTESIAN_POINT('Ctrl Pts',(3.77572872443219,-2.40288809370614,5.05181614590928));
#16015=CARTESIAN_POINT('Ctrl Pts',(3.75928777076399,-2.35024904339754,5.05552074226154));
#16016=CARTESIAN_POINT('Ctrl Pts',(3.74284681709578,-2.29760999308894,5.05922533861381));
#16017=CARTESIAN_POINT('Ctrl Pts',(3.69773195718207,-2.25392681404901,5.06292993496608));
#16018=CARTESIAN_POINT('Ctrl Pts',(3.6445902539118,-2.239191259641,5.06663453131835));
#16019=CARTESIAN_POINT('Ctrl Pts',(3.59144855064154,-2.22445570523299,5.07033912767062));
#16020=CARTESIAN_POINT('Ctrl Pts',(3.53028000401472,-2.2386677754569,5.07404372402289));
#16021=CARTESIAN_POINT('Ctrl Pts',(3.48907876340423,-2.27532343849,5.07774832037515));
#16022=CARTESIAN_POINT('Ctrl Pts',(3.45423196569032,-2.3063257203596,5.08088155902977));
#16023=CARTESIAN_POINT('Ctrl Pts',(3.43366833898609,-2.35338253026132,5.0840147976844));
#16024=CARTESIAN_POINT('Ctrl Pts',(3.43326718206005,-2.40013003210005,5.08714803633902));
#16025=CARTESIAN_POINT('Origin',(3.6,-2.4,4.7));
#16026=CARTESIAN_POINT('',(3.43325215766083,-2.39987843114813,5.15714803633902));
#16027=CARTESIAN_POINT('',(3.43361559198215,-2.39990578567643,5.13785196366098));
#16028=CARTESIAN_POINT('',(3.4334,-2.4,4.7));
#16029=CARTESIAN_POINT('',(3.72690708798524,-2.29206413469515,5.2));
#16030=CARTESIAN_POINT('Ctrl Pts',(3.43325215766083,-2.39987843114813,5.15714803633902));
#16031=CARTESIAN_POINT('Ctrl Pts',(3.43364568926707,-2.44715561674071,5.16031823516921));
#16032=CARTESIAN_POINT('Ctrl Pts',(3.45475450700198,-2.49473162154361,5.1634884339994));
#16033=CARTESIAN_POINT('Ctrl Pts',(3.49032381647516,-2.52575978121339,5.16665863282959));
#16034=CARTESIAN_POINT('Ctrl Pts',(3.53188901196771,-2.56201832942672,5.17036322918186));
#16035=CARTESIAN_POINT('Ctrl Pts',(3.59320078561411,-2.575679906312,5.17406782553413));
#16036=CARTESIAN_POINT('Ctrl Pts',(3.64619137793262,-2.5603849196725,5.17777242188639));
#16037=CARTESIAN_POINT('Ctrl Pts',(3.69918197025112,-2.545089933033,5.18147701823866));
#16038=CARTESIAN_POINT('Ctrl Pts',(3.74385138124173,-2.50083838286872,5.18518161459093));
#16039=CARTESIAN_POINT('Ctrl Pts',(3.75975547145412,-2.44813183978448,5.1888862109432));
#16040=CARTESIAN_POINT('Ctrl Pts',(3.7756595616665,-2.39542529670025,5.19259080729546));
#16041=CARTESIAN_POINT('Ctrl Pts',(3.76279833110066,-2.33426376069605,5.19629540364773));
#16042=CARTESIAN_POINT('Ctrl Pts',(3.72690708798524,-2.29206413469515,5.2));
#16043=CARTESIAN_POINT('',(3.47285247305911,-2.29187966783456,5.2));
#16044=CARTESIAN_POINT('Origin',(3.6,-2.4,5.2));
#16045=CARTESIAN_POINT('Ctrl Pts',(3.47285232078578,-2.29187955100914,5.2));
#16046=CARTESIAN_POINT('Ctrl Pts',(3.50793811899511,-2.25072740472549,5.19636770818144));
#16047=CARTESIAN_POINT('Ctrl Pts',(3.5649358740211,-2.22812243199181,5.19273541636289));
#16048=CARTESIAN_POINT('Ctrl Pts',(3.61867624862122,-2.23418211249055,5.18910312454433));
#16049=CARTESIAN_POINT('Ctrl Pts',(3.67348638108252,-2.24036241721079,5.18539852819207));
#16050=CARTESIAN_POINT('Ctrl Pts',(3.72490815931237,-2.27635993281072,5.1816939318398));
#16051=CARTESIAN_POINT('Ctrl Pts',(3.74944162123119,-2.32574103985171,5.17798933548753));
#16052=CARTESIAN_POINT('Ctrl Pts',(3.77397508315002,-2.37512214689269,5.17428473913527));
#16053=CARTESIAN_POINT('Ctrl Pts',(3.77162022875783,-2.43788684537472,5.17058014278299));
#16054=CARTESIAN_POINT('Ctrl Pts',(3.74343805414309,-2.48529019582313,5.16687554643072));
#16055=CARTESIAN_POINT('Ctrl Pts',(3.71525587952836,-2.53269354627153,5.16317095007846));
#16056=CARTESIAN_POINT('Ctrl Pts',(3.66124638469108,-2.5647355486863,5.15946635372619));
#16057=CARTESIAN_POINT('Ctrl Pts',(3.60613566942556,-2.56676214228893,5.15576175737392));
#16058=CARTESIAN_POINT('Ctrl Pts',(3.55102495416005,-2.56878873589157,5.15205716102166));
#16059=CARTESIAN_POINT('Ctrl Pts',(3.49481301846629,-2.54079992068208,5.14835256466939));
#16060=CARTESIAN_POINT('Ctrl Pts',(3.46322140367409,-2.49559987057215,5.14464796831712));
#16061=CARTESIAN_POINT('Ctrl Pts',(3.44390335110665,-2.46796035452279,5.14238263343174));
#16062=CARTESIAN_POINT('Ctrl Pts',(3.43379142096037,-2.43388514918463,5.14011729854636));
#16063=CARTESIAN_POINT('Ctrl Pts',(3.43361559198215,-2.39990578567643,5.13785196366098));
#16064=CARTESIAN_POINT('Origin',(3.6,-2.4,5.35459252805377));
#16065=CARTESIAN_POINT('',(3.39427732444531,-2.39988044480691,4.34540747194623));
#16066=CARTESIAN_POINT('',(3.39483887958286,-2.40008013132228,4.33959252805377));
#16067=CARTESIAN_POINT('',(3.394525,-2.39999999999999,5.35459252805377));
#16068=CARTESIAN_POINT('',(3.78826275096636,-2.48232321801033,4.3));
#16069=CARTESIAN_POINT('Ctrl Pts',(3.39483887958286,-2.40008013132228,4.33959252805377));
#16070=CARTESIAN_POINT('Ctrl Pts',(3.39495668787724,-2.361520075325,4.33750880775932));
#16071=CARTESIAN_POINT('Ctrl Pts',(3.4239416532562,-2.25423614055743,4.3317204911126));
#16072=CARTESIAN_POINT('Ctrl Pts',(3.59702530195382,-2.15700945407857,4.32222757811361));
#16073=CARTESIAN_POINT('Ctrl Pts',(3.80250230755732,-2.26611609660926,4.31111378905681));
#16074=CARTESIAN_POINT('Ctrl Pts',(3.81563717950601,-2.41972137435598,4.30370459635227));
#16075=CARTESIAN_POINT('Ctrl Pts',(3.78826275096636,-2.48232321801033,4.3));
#16076=CARTESIAN_POINT('',(3.72235839003881,-2.56553532314028,4.3));
#16077=CARTESIAN_POINT('Origin',(3.6,-2.4,4.3));
#16078=CARTESIAN_POINT('Ctrl Pts',(3.39427732444531,-2.39988044480691,4.34540747194623));
#16079=CARTESIAN_POINT('Ctrl Pts',(3.39422705601106,-2.39271640856816,4.34501772883951));
#16080=CARTESIAN_POINT('Ctrl Pts',(3.39781628789546,-2.31750701228878,4.34092338938053));
#16081=CARTESIAN_POINT('Ctrl Pts',(3.49037003077072,-2.18326698967564,4.33312445356928));
#16082=CARTESIAN_POINT('Ctrl Pts',(3.72265543153543,-2.19039239422561,4.32201066451247));
#16083=CARTESIAN_POINT('Ctrl Pts',(3.84179827282652,-2.38799091139141,4.31096917998938));
#16084=CARTESIAN_POINT('Ctrl Pts',(3.77594285680537,-2.52582029152411,4.30363229181855));
#16085=CARTESIAN_POINT('Ctrl Pts',(3.72235852099786,-2.56553552032367,4.3));
#16086=CARTESIAN_POINT('Origin',(3.6,-2.4,5.35459252805377));
#16087=CARTESIAN_POINT('',(3.39480735688311,-2.3998973457609,4.41540747194623));
#16088=CARTESIAN_POINT('',(3.39433274578554,-2.4001497810388,4.40959252805377));
#16089=CARTESIAN_POINT('',(3.394525,-2.39999999999999,5.35459252805377));
#16090=CARTESIAN_POINT('Ctrl Pts',(3.39433274578554,-2.4001497810388,4.40959252805377));
#16091=CARTESIAN_POINT('Ctrl Pts',(3.39481384891428,-2.34148051031483,4.40640305253959));
#16092=CARTESIAN_POINT('Ctrl Pts',(3.45186170282621,-2.21384965704481,4.39950898067315));
#16093=CARTESIAN_POINT('Ctrl Pts',(3.66843098386609,-2.16697244123634,4.38891031245443));
#16094=CARTESIAN_POINT('Ctrl Pts',(3.83289206448147,-2.33111753521892,4.37779652339763));
#16095=CARTESIAN_POINT('Ctrl Pts',(3.7841810615649,-2.55829573402952,4.36668273434082));
#16096=CARTESIAN_POINT('Ctrl Pts',(3.56689372435994,-2.6406156849541,4.35556894528403));
#16097=CARTESIAN_POINT('Ctrl Pts',(3.4149557748622,-2.52850415334516,4.34653887652167));
#16098=CARTESIAN_POINT('Ctrl Pts',(3.39474723933523,-2.4300750743674,4.34121340411158));
#16099=CARTESIAN_POINT('Ctrl Pts',(3.39483887958286,-2.40008013132228,4.33959252805377));
#16100=CARTESIAN_POINT('Ctrl Pts',(3.39480735688311,-2.3998973457609,4.41540747194623));
#16101=CARTESIAN_POINT('Ctrl Pts',(3.39468219270667,-2.3722256242847,4.41391197361979));
#16102=CARTESIAN_POINT('Ctrl Pts',(3.4127838411683,-2.27616341542302,4.40871187894107));
#16103=CARTESIAN_POINT('Ctrl Pts',(3.55878722400007,-2.16065655916503,4.3998071879101));
#16104=CARTESIAN_POINT('Ctrl Pts',(3.77873474447839,-2.23556893008468,4.38869339885329));
#16105=CARTESIAN_POINT('Ctrl Pts',(3.83508286096032,-2.4609855401145,4.37757960979649));
#16106=CARTESIAN_POINT('Ctrl Pts',(3.67625990251943,-2.63058416437082,4.36646582073969));
#16107=CARTESIAN_POINT('Ctrl Pts',(3.45564722516575,-2.59057499098668,4.3557417747896));
#16108=CARTESIAN_POINT('Ctrl Pts',(3.39470486884463,-2.46081219284274,4.34872232519178));
#16109=CARTESIAN_POINT('Ctrl Pts',(3.39427732444531,-2.39988044480691,4.34540747194623));
#16110=CARTESIAN_POINT('Origin',(3.6,-2.4,5.35459252805377));
#16111=CARTESIAN_POINT('',(3.39465010821578,-2.400176527643,4.48540747194623));
#16112=CARTESIAN_POINT('',(3.39437120606287,-2.39983660975581,4.47959252805377));
#16113=CARTESIAN_POINT('',(3.394525,-2.39999999999999,5.35459252805377));
#16114=CARTESIAN_POINT('Ctrl Pts',(3.39437120606287,-2.39983660975581,4.47959252805376));
#16115=CARTESIAN_POINT('Ctrl Pts',(3.39427673427304,-2.3889667776849,4.47900189367213));
#16116=CARTESIAN_POINT('Ctrl Pts',(3.40000383699504,-2.31001856010007,4.47470666293823));
#16117=CARTESIAN_POINT('Ctrl Pts',(3.50226148839652,-2.17766948860297,4.46670683585206));
#16118=CARTESIAN_POINT('Ctrl Pts',(3.73378446004359,-2.19730463405286,4.45559304679526));
#16119=CARTESIAN_POINT('Ctrl Pts',(3.84285302402677,-2.40246926900864,4.44447925773845));
#16120=CARTESIAN_POINT('Ctrl Pts',(3.72963540924699,-2.60537350906572,4.43336546868165));
#16121=CARTESIAN_POINT('Ctrl Pts',(3.49776113780875,-2.62029753773771,4.42225167962485));
#16122=CARTESIAN_POINT('Ctrl Pts',(3.39915518843152,-2.48716469789757,4.41432736608222));
#16123=CARTESIAN_POINT('Ctrl Pts',(3.3942550445316,-2.40962524613366,4.41010764889186));
#16124=CARTESIAN_POINT('Ctrl Pts',(3.39433274578554,-2.4001497810388,4.40959252805377));
#16125=CARTESIAN_POINT('Ctrl Pts',(3.39465010821578,-2.400176527643,4.48540747194623));
#16126=CARTESIAN_POINT('Ctrl Pts',(3.3950436881435,-2.35213729673001,4.48280621840006));
#16127=CARTESIAN_POINT('Ctrl Pts',(3.43581223913156,-2.23508079066125,4.47650036850162));
#16128=CARTESIAN_POINT('Ctrl Pts',(3.63081864021225,-2.15909778094929,4.46648992225093));
#16129=CARTESIAN_POINT('Ctrl Pts',(3.81910984016012,-2.29524053287965,4.45537613319411));
#16130=CARTESIAN_POINT('Ctrl Pts',(3.80684729577664,-2.52727079162485,4.44426234413733));
#16131=CARTESIAN_POINT('Ctrl Pts',(3.60525512132335,-2.64280869447754,4.4331485550805));
#16132=CARTESIAN_POINT('Ctrl Pts',(3.42662678112532,-2.55045981030713,4.42353026435015));
#16133=CARTESIAN_POINT('Ctrl Pts',(3.39499224504393,-2.44077304866432,4.41761656997206));
#16134=CARTESIAN_POINT('Ctrl Pts',(3.39480735688311,-2.3998973457609,4.41540747194623));
#16135=CARTESIAN_POINT('Origin',(3.6,-2.4,5.35459252805377));
#16136=CARTESIAN_POINT('',(3.39418406677318,-2.39999917227821,4.55540747194623));
#16137=CARTESIAN_POINT('',(3.39484823116951,-2.39995310238382,4.54959252805377));
#16138=CARTESIAN_POINT('',(3.394525,-2.39999999999999,5.35459252805377));
#16139=CARTESIAN_POINT('Ctrl Pts',(3.39484823116951,-2.39995310238382,4.54959252805377));
#16140=CARTESIAN_POINT('Ctrl Pts',(3.3947841219125,-2.36854855723416,4.54789613845241));
#16141=CARTESIAN_POINT('Ctrl Pts',(3.41632348134282,-2.26864576454574,4.54249515249878));
#16142=CARTESIAN_POINT('Ctrl Pts',(3.57178888017207,-2.15877849637109,4.53338957019289));
#16143=CARTESIAN_POINT('Ctrl Pts',(3.78736362800739,-2.2454731342224,4.52227578113608));
#16144=CARTESIAN_POINT('Ctrl Pts',(3.83144232268012,-2.47360796667095,4.51116199207928));
#16145=CARTESIAN_POINT('Ctrl Pts',(3.66367923386702,-2.6343685886554,4.50004820302247));
#16146=CARTESIAN_POINT('Ctrl Pts',(3.44964305628728,-2.58346600654441,4.48952504834731));
#16147=CARTESIAN_POINT('Ctrl Pts',(3.39486928333363,-2.45714489513262,4.4827064900244));
#16148=CARTESIAN_POINT('Ctrl Pts',(3.39437120606287,-2.39983660975581,4.47959252805376));
#16149=CARTESIAN_POINT('Ctrl Pts',(3.39418406845602,-2.39999917228229,4.55540747194623));
#16150=CARTESIAN_POINT('Ctrl Pts',(3.39418406581063,-2.39995488126817,4.55540505953261));
#16151=CARTESIAN_POINT('Ctrl Pts',(3.39420413582033,-2.33189558582108,4.55169805076672));
#16152=CARTESIAN_POINT('Ctrl Pts',(3.46841583417461,-2.19586946879708,4.54428644564855));
#16153=CARTESIAN_POINT('Ctrl Pts',(3.70013762796088,-2.17873969637961,4.53317265659175));
#16154=CARTESIAN_POINT('Ctrl Pts',(3.84020231541317,-2.36413198929513,4.52205886753494));
#16155=CARTESIAN_POINT('Ctrl Pts',(3.7604070991348,-2.58235467884591,4.51094507847814));
#16156=CARTESIAN_POINT('Ctrl Pts',(3.53378944658573,-2.63366606347461,4.49983128942134));
#16157=CARTESIAN_POINT('Ctrl Pts',(3.40663179333208,-2.50914981953724,4.4913187539107));
#16158=CARTESIAN_POINT('Ctrl Pts',(3.39448316809474,-2.42055275737136,4.48651081475233));
#16159=CARTESIAN_POINT('Ctrl Pts',(3.39465010821578,-2.400176527643,4.48540747194623));
#16160=CARTESIAN_POINT('Origin',(3.6,-2.4,5.35459252805377));
#16161=CARTESIAN_POINT('',(3.39465252302706,-2.39982399270837,4.62540747194623));
#16162=CARTESIAN_POINT('',(3.39454319301877,-2.40018789160095,4.61959252805377));
#16163=CARTESIAN_POINT('',(3.394525,-2.39999999999999,5.35459252805377));
#16164=CARTESIAN_POINT('Ctrl Pts',(3.39454319301877,-2.40018789160095,4.61959252805377));
#16165=CARTESIAN_POINT('Ctrl Pts',(3.39501369486734,-2.34850703974388,4.61679038323268));
#16166=CARTESIAN_POINT('Ctrl Pts',(3.44097935155591,-2.22775547868952,4.61028364205933));
#16167=CARTESIAN_POINT('Ctrl Pts',(3.64379902793915,-2.16111650041238,4.60007230453371));
#16168=CARTESIAN_POINT('Ctrl Pts',(3.82445363439269,-2.30724091831967,4.58895851547691));
#16169=CARTESIAN_POINT('Ctrl Pts',(3.79966328381548,-2.53826877567792,4.57784472642011));
#16170=CARTESIAN_POINT('Ctrl Pts',(3.59211886521387,-2.64273765452468,4.5667309373633));
#16171=CARTESIAN_POINT('Ctrl Pts',(3.42236627541046,-2.54299330864641,4.55731353790785));
#16172=CARTESIAN_POINT('Ctrl Pts',(3.39492412449178,-2.43713018689806,4.55160073480468));
#16173=CARTESIAN_POINT('Ctrl Pts',(3.39484823116951,-2.39995310238382,4.54959252805377));
#16174=CARTESIAN_POINT('Ctrl Pts',(3.39465252302706,-2.39982399270837,4.62540747194623));
#16175=CARTESIAN_POINT('Ctrl Pts',(3.39448549072207,-2.37935805029673,4.62429930431288));
#16176=CARTESIAN_POINT('Ctrl Pts',(3.40670160391397,-2.29066952405396,4.61948654032727));
#16177=CARTESIAN_POINT('Ctrl Pts',(3.53409308711521,-2.16624811163355,4.61096917998937));
#16178=CARTESIAN_POINT('Ctrl Pts',(3.76064388390312,-2.21785387995996,4.59985539093258));
#16179=CARTESIAN_POINT('Ctrl Pts',(3.8401555119317,-2.4361800576391,4.58874160187577));
#16180=CARTESIAN_POINT('Ctrl Pts',(3.69985007633495,-2.62139021824623,4.57762781281896));
#16181=CARTESIAN_POINT('Ctrl Pts',(3.4682010273,-2.60396318498582,4.56651643617578));
#16182=CARTESIAN_POINT('Ctrl Pts',(3.39418812817678,-2.46796988817124,4.55910965588488));
#16183=CARTESIAN_POINT('Ctrl Pts',(3.39418406845602,-2.39999917228229,4.55540747194623));
#16184=CARTESIAN_POINT('Origin',(3.6,-2.4,5.35459252805377));
#16185=CARTESIAN_POINT('',(3.39480597714356,-2.40010391086475,4.69540747194623));
#16186=CARTESIAN_POINT('',(3.39421139045774,-2.39993212258527,4.68959252805377));
#16187=CARTESIAN_POINT('',(3.394525,-2.39999999999999,5.35459252805377));
#16188=CARTESIAN_POINT('Ctrl Pts',(3.39421139045774,-2.39993212258527,4.68959252805377));
#16189=CARTESIAN_POINT('Ctrl Pts',(3.39419531835948,-2.39619821368606,4.68938922436523));
#16190=CARTESIAN_POINT('Ctrl Pts',(3.3959796089401,-2.32444075084805,4.68548132432442));
#16191=CARTESIAN_POINT('Ctrl Pts',(3.47964553863801,-2.18905336016944,4.67786882793135));
#16192=CARTESIAN_POINT('Ctrl Pts',(3.71195459122784,-2.18447772567898,4.66675503887453));
#16193=CARTESIAN_POINT('Ctrl Pts',(3.84179033681535,-2.37717207306315,4.65564124981774));
#16194=CARTESIAN_POINT('Ctrl Pts',(3.75031264502696,-2.59076108085938,4.64452746076093));
#16195=CARTESIAN_POINT('Ctrl Pts',(3.52125208458385,-2.6297443079663,4.63341367170413));
#16196=CARTESIAN_POINT('Ctrl Pts',(3.40385053605922,-2.50163131684181,4.6251020274684));
#16197=CARTESIAN_POINT('Ctrl Pts',(3.39439166440737,-2.4168320934068,4.62049497958495));
#16198=CARTESIAN_POINT('Ctrl Pts',(3.39454319301877,-2.40018789160095,4.61959252805377));
#16199=CARTESIAN_POINT('Ctrl Pts',(3.39480597714356,-2.40010391086475,4.69540747194623));
#16200=CARTESIAN_POINT('Ctrl Pts',(3.39499357523214,-2.35913959871511,4.69319354909316));
#16201=CARTESIAN_POINT('Ctrl Pts',(3.42673278397032,-2.24936123585863,4.68727502988782));
#16202=CARTESIAN_POINT('Ctrl Pts',(3.60557055480924,-2.15719836203143,4.6776519143302));
#16203=CARTESIAN_POINT('Ctrl Pts',(3.8070124874506,-2.27299804520947,4.6665381252734));
#16204=CARTESIAN_POINT('Ctrl Pts',(3.81897354264718,-2.50504405790744,4.65542433621659));
#16205=CARTESIAN_POINT('Ctrl Pts',(3.63050563092984,-2.64094205312202,4.64431054715979));
#16206=CARTESIAN_POINT('Ctrl Pts',(3.4356920506335,-2.56474249848871,4.63430492573633));
#16207=CARTESIAN_POINT('Ctrl Pts',(3.39504387850492,-2.44777554718273,4.62800390066515));
#16208=CARTESIAN_POINT('Ctrl Pts',(3.39465252302706,-2.39982399270837,4.62540747194623));
#16209=CARTESIAN_POINT('Origin',(3.6,-2.4,5.35459252805377));
#16210=CARTESIAN_POINT('',(3.39427330737243,-2.40012021866021,4.76540747194624));
#16211=CARTESIAN_POINT('',(3.39474358824326,-2.39985490132356,4.75959252805377));
#16212=CARTESIAN_POINT('',(3.394525,-2.39999999999999,5.35459252805377));
#16213=CARTESIAN_POINT('Ctrl Pts',(3.39474358824326,-2.39985490132356,4.75959252805377));
#16214=CARTESIAN_POINT('Ctrl Pts',(3.39458577609892,-2.37565177668507,4.75828346914551));
#16215=CARTESIAN_POINT('Ctrl Pts',(3.40973684003147,-2.28314575562072,4.75326981388497));
#16216=CARTESIAN_POINT('Ctrl Pts',(3.546828337511,-2.16302646659663,4.74455156227216));
#16217=CARTESIAN_POINT('Ctrl Pts',(3.77025746015408,-2.22680624004484,4.73343777321537));
#16218=CARTESIAN_POINT('Ctrl Pts',(3.83784799866721,-2.44911222613084,4.72232398415856));
#16219=CARTESIAN_POINT('Ctrl Pts',(3.68773356662048,-2.62646523466876,4.71121019510175));
#16220=CARTESIAN_POINT('Ctrl Pts',(3.46153062411222,-2.59707961114918,4.7002997097335));
#16221=CARTESIAN_POINT('Ctrl Pts',(3.3944881838605,-2.46423743809455,4.6930938207175));
#16222=CARTESIAN_POINT('Ctrl Pts',(3.39421139045774,-2.39993212258527,4.68959252805377));
#16223=CARTESIAN_POINT('Ctrl Pts',(3.39427330737243,-2.40012021866021,4.76540747194624));
#16224=CARTESIAN_POINT('Ctrl Pts',(3.39469744970711,-2.3391019374956,4.76208779387343));
#16225=CARTESIAN_POINT('Ctrl Pts',(3.45579878082125,-2.20925256261312,4.75506351944836));
#16226=CARTESIAN_POINT('Ctrl Pts',(3.67655777933124,-2.16951665373617,4.74433464867103));
#16227=CARTESIAN_POINT('Ctrl Pts',(3.83516271561975,-2.33931916560024,4.73322085961422));
#16228=CARTESIAN_POINT('Ctrl Pts',(3.77852055137491,-2.56466353335787,4.72210707055742));
#16229=CARTESIAN_POINT('Ctrl Pts',(3.55847650189588,-2.63928950162157,4.71099328150062));
#16230=CARTESIAN_POINT('Ctrl Pts',(3.41270209403565,-2.52365597038275,4.70209341529688));
#16231=CARTESIAN_POINT('Ctrl Pts',(3.3946796640253,-2.4276859083356,4.69689814544542));
#16232=CARTESIAN_POINT('Ctrl Pts',(3.39480597714356,-2.40010391086475,4.69540747194623));
#16233=CARTESIAN_POINT('Origin',(3.6,-2.4,5.35459252805377));
#16234=CARTESIAN_POINT('',(3.39444175959654,-2.39982008597895,4.83540747194623));
#16235=CARTESIAN_POINT('',(3.39473575570154,-2.40014879661129,4.82959252805377));
#16236=CARTESIAN_POINT('',(3.394525,-2.39999999999999,5.35459252805377));
#16237=CARTESIAN_POINT('Ctrl Pts',(3.39473575570154,-2.40014879661129,4.82959252805377));
#16238=CARTESIAN_POINT('Ctrl Pts',(3.39503502367394,-2.35550570215801,4.82717771392578));
#16239=CARTESIAN_POINT('Ctrl Pts',(3.43129921618784,-2.24193240937533,4.82105830344552));
#16240=CARTESIAN_POINT('Ctrl Pts',(3.61869057055051,-2.15785470519124,4.81123429661299));
#16241=CARTESIAN_POINT('Ctrl Pts',(3.81357662274397,-2.28437687323548,4.80012050755619));
#16242=CARTESIAN_POINT('Ctrl Pts',(3.81297357001622,-2.51673020046272,4.78900671849938));
#16243=CARTESIAN_POINT('Ctrl Pts',(3.61743339336808,-2.64223905139592,4.77789292944258));
#16244=CARTESIAN_POINT('Ctrl Pts',(3.43084783163214,-2.55735665460818,4.76808819929404));
#16245=CARTESIAN_POINT('Ctrl Pts',(3.39503237960207,-2.44414587323265,4.76198806549777));
#16246=CARTESIAN_POINT('Ctrl Pts',(3.39474358824326,-2.39985490132356,4.75959252805377));
#16247=CARTESIAN_POINT('Ctrl Pts',(3.39444175959654,-2.39982008597895,4.83540747194623));
#16248=CARTESIAN_POINT('Ctrl Pts',(3.39432007222796,-2.3865422800919,4.83468663500598));
#16249=CARTESIAN_POINT('Ctrl Pts',(3.40154215697383,-2.30515767781734,4.83026120171345));
#16250=CARTESIAN_POINT('Ctrl Pts',(3.51011506636152,-2.17438004258061,4.82213117206865));
#16251=CARTESIAN_POINT('Ctrl Pts',(3.74080744720095,-2.20211890112026,4.81101738301186));
#16252=CARTESIAN_POINT('Ctrl Pts',(3.84261717475225,-2.41098057358878,4.79990359395505));
#16253=CARTESIAN_POINT('Ctrl Pts',(3.72235665078693,-2.60979160252334,4.78878980489825));
#16254=CARTESIAN_POINT('Ctrl Pts',(3.49010169673754,-2.61657799846968,4.77767601584144));
#16255=CARTESIAN_POINT('Ctrl Pts',(3.3977657533099,-2.4823139974067,4.76988190485744));
#16256=CARTESIAN_POINT('Ctrl Pts',(3.39422412786341,-2.40719531789781,4.7657923902257));
#16257=CARTESIAN_POINT('Ctrl Pts',(3.39427330737243,-2.40012021866021,4.76540747194624));
#16258=CARTESIAN_POINT('Origin',(3.6,-2.4,5.35459252805377));
#16259=CARTESIAN_POINT('',(3.39485784898994,-2.39999218980985,4.90540747194623));
#16260=CARTESIAN_POINT('',(3.39420666496973,-2.4000617379826,4.89959252805377));
#16261=CARTESIAN_POINT('',(3.394525,-2.39999999999999,5.35459252805377));
#16262=CARTESIAN_POINT('Ctrl Pts',(3.39420666496973,-2.4000617379826,4.89959252805377));
#16263=CARTESIAN_POINT('Ctrl Pts',(3.39446260190468,-2.33540634192885,4.89607195870605));
#16264=CARTESIAN_POINT('Ctrl Pts',(3.46215556821269,-2.20225412189412,4.88884679300607));
#16265=CARTESIAN_POINT('Ctrl Pts',(3.68890791813162,-2.17399322284688,4.87791703095382));
#16266=CARTESIAN_POINT('Ctrl Pts',(3.83809972557463,-2.3521230545377,4.86680324189701));
#16267=CARTESIAN_POINT('Ctrl Pts',(3.76935615396461,-2.57407519737118,4.85568945284021));
#16268=CARTESIAN_POINT('Ctrl Pts',(3.54559897400137,-2.63669433790405,4.8445756637834));
#16269=CARTESIAN_POINT('Ctrl Pts',(3.4094345739418,-2.51613221625325,4.83587668885459));
#16270=CARTESIAN_POINT('Ctrl Pts',(3.39457591295976,-2.42399322794668,4.83088231027805));
#16271=CARTESIAN_POINT('Ctrl Pts',(3.39473575570154,-2.40014879661129,4.82959252805377));
#16272=CARTESIAN_POINT('Ctrl Pts',(3.39485784898994,-2.39999218980985,4.90540747194623));
#16273=CARTESIAN_POINT('Ctrl Pts',(3.3948463830005,-2.36617331876133,4.90358087978625));
#16274=CARTESIAN_POINT('Ctrl Pts',(3.41876410056102,-2.26378009325356,4.898049691274));
#16275=CARTESIAN_POINT('Ctrl Pts',(3.5802619217345,-2.1579378700657,4.88881390640948));
#16276=CARTESIAN_POINT('Ctrl Pts',(3.7926651914697,-2.25213590538246,4.87770011735268));
#16277=CARTESIAN_POINT('Ctrl Pts',(3.8287198264784,-2.48167562339262,4.86658632829587));
#16278=CARTESIAN_POINT('Ctrl Pts',(3.65542461045338,-2.63645671704841,4.85547253923907));
#16279=CARTESIAN_POINT('Ctrl Pts',(3.44592887677019,-2.57880492333736,4.84507958712252));
#16280=CARTESIAN_POINT('Ctrl Pts',(3.39494545996352,-2.45478089066832,4.83839123135824));
#16281=CARTESIAN_POINT('Ctrl Pts',(3.39444175959654,-2.39982008597895,4.83540747194623));
#16282=CARTESIAN_POINT('Origin',(3.6,-2.4,5.35459252805377));
#16283=CARTESIAN_POINT('',(3.39447042869063,-2.40018396912367,4.97540747194623));
#16284=CARTESIAN_POINT('',(3.39455385196002,-2.39981229693528,4.96959252805377));
#16285=CARTESIAN_POINT('',(3.394525,-2.39999999999999,5.35459252805377));
#16286=CARTESIAN_POINT('Ctrl Pts',(3.39455385196002,-2.39981229693529,4.96959252805377));
#16287=CARTESIAN_POINT('Ctrl Pts',(3.39439994110979,-2.38281031884833,4.9686707998386));
#16288=CARTESIAN_POINT('Ctrl Pts',(3.40410690463755,-2.29764758883809,4.96404447527116));
#16289=CARTESIAN_POINT('Ctrl Pts',(3.52244569995759,-2.16985002334435,4.95571355435144));
#16290=CARTESIAN_POINT('Ctrl Pts',(3.75130082069111,-2.21002173048044,4.94459976529465));
#16291=CARTESIAN_POINT('Ctrl Pts',(3.84166858438312,-2.42408270226789,4.93348597623783));
#16292=CARTESIAN_POINT('Ctrl Pts',(3.71083435207858,-2.61610050352316,4.92237218718104));
#16293=CARTESIAN_POINT('Ctrl Pts',(3.47855218037073,-2.61031906317225,4.91125839812423));
#16294=CARTESIAN_POINT('Ctrl Pts',(3.3958002253152,-2.47484313295797,4.90366517841514));
#16295=CARTESIAN_POINT('Ctrl Pts',(3.39419328664854,-2.40344140123838,4.89977655505832));
#16296=CARTESIAN_POINT('Ctrl Pts',(3.39420666496973,-2.4000617379826,4.89959252805377));
#16297=CARTESIAN_POINT('Ctrl Pts',(3.39447042869063,-2.40018396912367,4.97540747194623));
#16298=CARTESIAN_POINT('Ctrl Pts',(3.39496908844141,-2.34615078794508,4.97247512456653));
#16299=CARTESIAN_POINT('Ctrl Pts',(3.44450059908404,-2.22304562253723,4.96583818083456));
#16300=CARTESIAN_POINT('Ctrl Pts',(3.65214584962031,-2.16279865748873,4.9554966407503));
#16301=CARTESIAN_POINT('Ctrl Pts',(3.82756721091734,-2.31516586178242,4.94438285169351));
#16302=CARTESIAN_POINT('Ctrl Pts',(3.79469372311971,-2.54518271468373,4.9332690626367));
#16303=CARTESIAN_POINT('Ctrl Pts',(3.58361486265069,-2.64231218244471,4.9221552735799));
#16304=CARTESIAN_POINT('Ctrl Pts',(3.41976019754822,-2.53813915804107,4.91286807668307));
#16305=CARTESIAN_POINT('Ctrl Pts',(3.39486963770596,-2.43476294104758,4.90728547613852));
#16306=CARTESIAN_POINT('Ctrl Pts',(3.39485784898994,-2.39999218980985,4.90540747194623));
#16307=CARTESIAN_POINT('Origin',(3.6,-2.4,5.35459252805377));
#16308=CARTESIAN_POINT('',(3.39425291505627,-2.39989343747799,5.04540747194623));
#16309=CARTESIAN_POINT('',(3.39484565493551,-2.40005255540929,5.03959252805377));
#16310=CARTESIAN_POINT('',(3.394525,-2.39999999999999,5.35459252805377));
#16311=CARTESIAN_POINT('Ctrl Pts',(3.39484565493551,-2.40005255540928,5.03959252805377));
#16312=CARTESIAN_POINT('Ctrl Pts',(3.39493157796431,-2.36251978536397,5.03756504461887));
#16313=CARTESIAN_POINT('Ctrl Pts',(3.42276239101834,-2.25628891765328,5.03183296483171));
#16314=CARTESIAN_POINT('Ctrl Pts',(3.59337897177386,-2.15722470850713,5.02239628869227));
#16315=CARTESIAN_POINT('Ctrl Pts',(3.8003783179889,-2.26276949623011,5.01128249963547));
#16316=CARTESIAN_POINT('Ctrl Pts',(3.82396911763155,-2.49392292422242,5.00016871057867));
#16317=CARTESIAN_POINT('Ctrl Pts',(3.64255844375993,-2.63910763258347,4.98905492152186));
#16318=CARTESIAN_POINT('Ctrl Pts',(3.44046962807591,-2.57154454308001,4.97886286068022));
#16319=CARTESIAN_POINT('Ctrl Pts',(3.39501853731303,-2.45114441665013,4.97237539619086));
#16320=CARTESIAN_POINT('Ctrl Pts',(3.39455385196002,-2.39981229693529,4.96959252805377));
#16321=CARTESIAN_POINT('Ctrl Pts',(3.39425291505627,-2.39989343747799,5.04540747194623));
#16322=CARTESIAN_POINT('Ctrl Pts',(3.39421423202935,-2.39376493107826,5.04507396569907));
#16323=CARTESIAN_POINT('Ctrl Pts',(3.39724233967252,-2.31959956972988,5.04103586309963));
#16324=CARTESIAN_POINT('Ctrl Pts',(3.48711398605093,-2.18496417501817,5.03329316414794));
#16325=CARTESIAN_POINT('Ctrl Pts',(3.71944061581356,-2.18853461914439,5.02217937509113));
#16326=CARTESIAN_POINT('Ctrl Pts',(3.84244191526684,-2.38566174871763,5.01106558603433));
#16327=CARTESIAN_POINT('Ctrl Pts',(3.74353337026135,-2.59591283022398,4.99995179697752));
#16328=CARTESIAN_POINT('Ctrl Pts',(3.51324710863985,-2.62684268245385,4.98883800792072));
#16329=CARTESIAN_POINT('Ctrl Pts',(3.40217618139952,-2.49676321865199,4.98065656624362));
#16330=CARTESIAN_POINT('Ctrl Pts',(3.3943391040451,-2.41441388913183,4.97617972091879));
#16331=CARTESIAN_POINT('Ctrl Pts',(3.39447042869063,-2.40018396912367,4.97540747194623));
#16332=CARTESIAN_POINT('Origin',(3.6,-2.4,5.35459252805377));
#16333=CARTESIAN_POINT('',(3.39479089893477,-2.39988380139174,5.11540747194623));
#16334=CARTESIAN_POINT('',(3.39436118987868,-2.40016037422423,5.10959252805377));
#16335=CARTESIAN_POINT('',(3.394525,-2.39999999999999,5.35459252805377));
#16336=CARTESIAN_POINT('Ctrl Pts',(3.39436118987868,-2.40016037422423,5.10959252805377));
#16337=CARTESIAN_POINT('Ctrl Pts',(3.39485595410064,-2.34250465429438,5.10645928939914));
#16338=CARTESIAN_POINT('Ctrl Pts',(3.45020483509149,-2.21584694899168,5.09962145439226));
#16339=CARTESIAN_POINT('Ctrl Pts',(3.66489494634582,-2.16596525152154,5.08907902303309));
#16340=CARTESIAN_POINT('Ctrl Pts',(3.83182128201397,-2.32759432498908,5.07796523397629));
#16341=CARTESIAN_POINT('Ctrl Pts',(3.78655899034249,-2.55549738341204,5.06685144491949));
#16342=CARTESIAN_POINT('Ctrl Pts',(3.57053712854092,-2.64107179875281,5.05573765586268));
#16343=CARTESIAN_POINT('Ctrl Pts',(3.4159720352905,-2.53063333972521,5.04665135024078));
#16344=CARTESIAN_POINT('Ctrl Pts',(3.39477458031215,-2.43109926700468,5.04126964097114));
#16345=CARTESIAN_POINT('Ctrl Pts',(3.39484565493551,-2.40005255540928,5.03959252805377));
#16346=CARTESIAN_POINT('Ctrl Pts',(3.39479089893477,-2.39988380139174,5.11540747194623));
#16347=CARTESIAN_POINT('Ctrl Pts',(3.39465312034679,-2.37325776527266,5.11396821047934));
#16348=CARTESIAN_POINT('Ctrl Pts',(3.41183995517004,-2.27826800227929,5.10882435266019));
#16349=CARTESIAN_POINT('Ctrl Pts',(3.55516853033383,-2.16130913937078,5.09997589848876));
#16350=CARTESIAN_POINT('Ctrl Pts',(3.77622352465696,-2.23288041708187,5.08886210943196));
#16351=CARTESIAN_POINT('Ctrl Pts',(3.83598040928192,-2.457419700552,5.07774832037515));
#16352=CARTESIAN_POINT('Ctrl Pts',(3.67974110927284,-2.62940130358481,5.06663453131835));
#16353=CARTESIAN_POINT('Ctrl Pts',(3.45739290427932,-2.59254974530072,5.05585424850871));
#16354=CARTESIAN_POINT('Ctrl Pts',(3.39464392413157,-2.46184054479285,5.04877856205133));
#16355=CARTESIAN_POINT('Ctrl Pts',(3.39425291505627,-2.39989343747799,5.04540747194623));
#16356=CARTESIAN_POINT('Origin',(3.6,-2.4,5.35459252805377));
#16357=CARTESIAN_POINT('',(3.39473290683218,-2.40022967700174,5.18540747194623));
#16358=CARTESIAN_POINT('',(3.39434265963601,-2.39985006386652,5.17959252805377));
#16359=CARTESIAN_POINT('',(3.394525,-2.39999999999999,5.35459252805377));
#16360=CARTESIAN_POINT('',(3.54698297828114,-2.59851743256717,5.2));
#16361=CARTESIAN_POINT('Ctrl Pts',(3.54698297828114,-2.59851743256717,5.2));
#16362=CARTESIAN_POINT('Ctrl Pts',(3.48097120902544,-2.58088801151799,5.19629540364773));
#16363=CARTESIAN_POINT('Ctrl Pts',(3.40750558819668,-2.51127201784738,5.19143122762981));
#16364=CARTESIAN_POINT('Ctrl Pts',(3.39457125535004,-2.42165321144002,5.18656705161189));
#16365=CARTESIAN_POINT('Ctrl Pts',(3.39473290683218,-2.40022967700174,5.18540747194623));
#16366=CARTESIAN_POINT('',(3.65313154707148,-2.59887322485902,5.2));
#16367=CARTESIAN_POINT('Origin',(3.6,-2.4,5.2));
#16368=CARTESIAN_POINT('Ctrl Pts',(3.65313161981587,-2.59887345085171,5.2));
#16369=CARTESIAN_POINT('Ctrl Pts',(3.58867174169549,-2.61600530781671,5.19636770818145));
#16370=CARTESIAN_POINT('Ctrl Pts',(3.45069167513782,-2.58406709125274,5.1895652175327));
#16371=CARTESIAN_POINT('Ctrl Pts',(3.3948280192206,-2.45815906572508,5.18276272688396));
#16372=CARTESIAN_POINT('Ctrl Pts',(3.39434265963601,-2.39985006386652,5.17959252805377));
#16373=CARTESIAN_POINT('Origin',(3.6,2.4,4.7));
#16374=CARTESIAN_POINT('',(3.43324411482341,2.39987855685961,4.38714803633902));
#16375=CARTESIAN_POINT('',(3.43319917606922,2.4000969362753,4.36785196366098));
#16376=CARTESIAN_POINT('',(3.4334,2.4,4.7));
#16377=CARTESIAN_POINT('',(3.43648706727485,2.36807695453719,4.3));
#16378=CARTESIAN_POINT('Ctrl Pts',(3.43319917606922,2.4000969362753,4.36785196366098));
#16379=CARTESIAN_POINT('Ctrl Pts',(3.43315841823699,2.40590556741068,4.36746222055426));
#16380=CARTESIAN_POINT('Ctrl Pts',(3.43343543893775,2.41171030674387,4.36707247744754));
#16381=CARTESIAN_POINT('Ctrl Pts',(3.43404307301465,2.41748025740019,4.36668273434083));
#16382=CARTESIAN_POINT('Ctrl Pts',(3.43981877230484,2.47232494300381,4.36297813798856));
#16383=CARTESIAN_POINT('Ctrl Pts',(3.475465166407,2.52402649519299,4.35927354163629));
#16384=CARTESIAN_POINT('Ctrl Pts',(3.52467802575654,2.54891438715568,4.35556894528402));
#16385=CARTESIAN_POINT('Ctrl Pts',(3.57389088510608,2.57380227911837,4.35186434893175));
#16386=CARTESIAN_POINT('Ctrl Pts',(3.636670209703,2.57187651085455,4.34815975257948));
#16387=CARTESIAN_POINT('Ctrl Pts',(3.68426556342447,2.54403648109996,4.34445515622722));
#16388=CARTESIAN_POINT('Ctrl Pts',(3.73186091714595,2.51619645134536,4.34075055987495));
#16389=CARTESIAN_POINT('Ctrl Pts',(3.76427229999197,2.46244216009999,4.33704596352268));
#16390=CARTESIAN_POINT('Ctrl Pts',(3.76670490932883,2.40733835348838,4.33334136717041));
#16391=CARTESIAN_POINT('Ctrl Pts',(3.76913751866569,2.35223454687676,4.32963677081814));
#16392=CARTESIAN_POINT('Ctrl Pts',(3.74159135449339,2.29578122489891,4.32593217446588));
#16393=CARTESIAN_POINT('Ctrl Pts',(3.69659413605431,2.26388777656513,4.32222757811361));
#16394=CARTESIAN_POINT('Ctrl Pts',(3.65159691761524,2.23199432823136,4.31852298176134));
#16395=CARTESIAN_POINT('Ctrl Pts',(3.5891486449094,2.22466075354166,4.31481838540907));
#16396=CARTESIAN_POINT('Ctrl Pts',(3.53802497534865,2.24508842505152,4.3111137890568));
#16397=CARTESIAN_POINT('Ctrl Pts',(3.4869013057879,2.26551609656139,4.30740919270454));
#16398=CARTESIAN_POINT('Ctrl Pts',(3.44710223937223,2.31370501427082,4.30370459635227));
#16399=CARTESIAN_POINT('Ctrl Pts',(3.43648706727485,2.36807695453719,4.3));
#16400=CARTESIAN_POINT('',(3.5947433343941,2.5668198697629,4.3));
#16401=CARTESIAN_POINT('Origin',(3.6,2.4,4.3));
#16402=CARTESIAN_POINT('',(3.43365448824955,2.39993503013922,4.31714803633902));
#16403=CARTESIAN_POINT('Ctrl Pts',(3.59474333802771,2.56682006235004,4.3));
#16404=CARTESIAN_POINT('Ctrl Pts',(3.54069368762274,2.56504680898901,4.30363229181856));
#16405=CARTESIAN_POINT('Ctrl Pts',(3.48748281235487,2.53457817870515,4.30726458363711));
#16406=CARTESIAN_POINT('Ctrl Pts',(3.45871386452964,2.48878411340601,4.31089687545566));
#16407=CARTESIAN_POINT('Ctrl Pts',(3.44221011333674,2.46251364065879,4.31298059575012));
#16408=CARTESIAN_POINT('Ctrl Pts',(3.43375000591375,2.43119968923457,4.31506431604457));
#16409=CARTESIAN_POINT('Ctrl Pts',(3.43365448824955,2.39993503013922,4.31714803633902));
#16410=CARTESIAN_POINT('',(3.4334,2.4,4.2));
#16411=CARTESIAN_POINT('',(3.4334,2.4,4.7));
#16412=CARTESIAN_POINT('Origin',(3.6,2.4,4.2));
#16413=CARTESIAN_POINT('Ctrl Pts',(3.43365448824955,2.39993503013922,4.31714803633902));
#16414=CARTESIAN_POINT('Ctrl Pts',(3.4335801873487,2.37561500142982,4.31876891239684));
#16415=CARTESIAN_POINT('Ctrl Pts',(3.43856722533918,2.35132479907035,4.32038978845465));
#16416=CARTESIAN_POINT('Ctrl Pts',(3.44876666696164,2.32946151839122,4.32201066451247));
#16417=CARTESIAN_POINT('Ctrl Pts',(3.47207802013238,2.27949185571287,4.32571526086474));
#16418=CARTESIAN_POINT('Ctrl Pts',(3.52261765366037,2.24219981905568,4.32941985721701));
#16419=CARTESIAN_POINT('Ctrl Pts',(3.57725038766107,2.23467802743392,4.33312445356927));
#16420=CARTESIAN_POINT('Ctrl Pts',(3.63188312166177,2.22715623581217,4.33682904992154));
#16421=CARTESIAN_POINT('Ctrl Pts',(3.69060895613519,2.24940468922586,4.34053364627381));
#16422=CARTESIAN_POINT('Ctrl Pts',(3.72655438764877,2.29122842499976,4.34423824262608));
#16423=CARTESIAN_POINT('Ctrl Pts',(3.76249981916235,2.33305216077365,4.34794283897835));
#16424=CARTESIAN_POINT('Ctrl Pts',(3.77566484771609,2.39445117890775,4.35164743533062));
#16425=CARTESIAN_POINT('Ctrl Pts',(3.76002307153489,2.44733227776831,4.35535203168288));
#16426=CARTESIAN_POINT('Ctrl Pts',(3.7443812953537,2.50021337662887,4.35905662803515));
#16427=CARTESIAN_POINT('Ctrl Pts',(3.69993271443756,2.5445765562159,4.36276122438742));
#16428=CARTESIAN_POINT('Ctrl Pts',(3.64702014888419,2.56011555645441,4.36646582073968));
#16429=CARTESIAN_POINT('Ctrl Pts',(3.59410758333083,2.57565455669293,4.37017041709195));
#16430=CARTESIAN_POINT('Ctrl Pts',(3.53273103314024,2.56236937758293,4.37387501344422));
#16431=CARTESIAN_POINT('Ctrl Pts',(3.49097948747713,2.52634165427837,4.37757960979649));
#16432=CARTESIAN_POINT('Ctrl Pts',(3.45503345721934,2.49532355395523,4.38076908531067));
#16433=CARTESIAN_POINT('Ctrl Pts',(3.43363419524109,2.44744785138174,4.38395856082484));
#16434=CARTESIAN_POINT('Ctrl Pts',(3.43324411482341,2.39987855685961,4.38714803633902));
#16435=CARTESIAN_POINT('Origin',(3.6,2.4,4.7));
#16436=CARTESIAN_POINT('',(3.43327529856389,2.40013247750357,4.45714803633902));
#16437=CARTESIAN_POINT('',(3.43362892985438,2.40008323250784,4.43785196366098));
#16438=CARTESIAN_POINT('',(3.4334,2.4,4.7));
#16439=CARTESIAN_POINT('Ctrl Pts',(3.43362892985438,2.40008323250784,4.43785196366098));
#16440=CARTESIAN_POINT('Ctrl Pts',(3.43352744619908,2.42251958229607,4.43635646533454));
#16441=CARTESIAN_POINT('Ctrl Pts',(3.43774838281902,2.44491933756368,4.43486096700809));
#16442=CARTESIAN_POINT('Ctrl Pts',(3.44647310901037,2.4654005396039,4.43336546868165));
#16443=CARTESIAN_POINT('Ctrl Pts',(3.46808569676891,2.5161358597488,4.42966087232938));
#16444=CARTESIAN_POINT('Ctrl Pts',(3.51733510120548,2.55509827110394,4.42595627597712));
#16445=CARTESIAN_POINT('Ctrl Pts',(3.57168220127168,2.56445626518835,4.42225167962485));
#16446=CARTESIAN_POINT('Ctrl Pts',(3.62602930133789,2.57381425927275,4.41854708327258));
#16447=CARTESIAN_POINT('Ctrl Pts',(3.68547409703373,2.55356783608644,4.41484248692031));
#16448=CARTESIAN_POINT('Ctrl Pts',(3.7228110439026,2.51298316629394,4.41113789056804));
#16449=CARTESIAN_POINT('Ctrl Pts',(3.76014799077148,2.47239849650144,4.40743329421577));
#16450=CARTESIAN_POINT('Ctrl Pts',(3.77537708881339,2.41147558010275,4.4037286978635));
#16451=CARTESIAN_POINT('Ctrl Pts',(3.76152924886074,2.35809557405986,4.40002410151124));
#16452=CARTESIAN_POINT('Ctrl Pts',(3.74768140890809,2.30471556801697,4.39631950515897));
#16453=CARTESIAN_POINT('Ctrl Pts',(3.70475663096088,2.25887847232986,4.3926149088067));
#16454=CARTESIAN_POINT('Ctrl Pts',(3.65239849394634,2.24156301733926,4.38891031245443));
#16455=CARTESIAN_POINT('Ctrl Pts',(3.6000403569318,2.22424756234866,4.38520571610217));
#16456=CARTESIAN_POINT('Ctrl Pts',(3.53824886084993,2.23545374805455,4.3815011197499));
#16457=CARTESIAN_POINT('Ctrl Pts',(3.49530561504809,2.27005075041653,4.37779652339763));
#16458=CARTESIAN_POINT('Ctrl Pts',(3.45688022556308,2.30100796536268,4.37448167015208));
#16459=CARTESIAN_POINT('Ctrl Pts',(3.43354583064794,2.35069321510765,4.37116681690653));
#16460=CARTESIAN_POINT('Ctrl Pts',(3.43319917606922,2.4000969362753,4.36785196366098));
#16461=CARTESIAN_POINT('Ctrl Pts',(3.43324411482341,2.39987855685961,4.38714803633902));
#16462=CARTESIAN_POINT('Ctrl Pts',(3.43318111432356,2.39219580941329,4.38766315717711));
#16463=CARTESIAN_POINT('Ctrl Pts',(3.4336661242569,2.38452105441581,4.3881782780152));
#16464=CARTESIAN_POINT('Ctrl Pts',(3.43472636939645,2.37692660019285,4.38869339885329));
#16465=CARTESIAN_POINT('Ctrl Pts',(3.44235133811452,2.32230953691099,4.39239799520556));
#16466=CARTESIAN_POINT('Ctrl Pts',(3.47972781668628,2.27184567784637,4.39610259155783));
#16467=CARTESIAN_POINT('Ctrl Pts',(3.52975016370933,2.24863049260891,4.3998071879101));
#16468=CARTESIAN_POINT('Ctrl Pts',(3.57977251073239,2.22541530737146,4.40351178426237));
#16469=CARTESIAN_POINT('Ctrl Pts',(3.64244072620675,2.22944879596115,4.40721638061463));
#16470=CARTESIAN_POINT('Ctrl Pts',(3.6890743879353,2.25888481053352,4.4109209769669));
#16471=CARTESIAN_POINT('Ctrl Pts',(3.73570804966386,2.28832082510588,4.41462557331917));
#16472=CARTESIAN_POINT('Ctrl Pts',(3.76630715764661,2.34315936566092,4.41833016967144));
#16473=CARTESIAN_POINT('Ctrl Pts',(3.76686783565003,2.39830336248822,4.4220347660237));
#16474=CARTESIAN_POINT('Ctrl Pts',(3.76742851365345,2.45344735931552,4.42573936237597));
#16475=CARTESIAN_POINT('Ctrl Pts',(3.73795076167754,2.5088968124151,4.42944395872824));
#16476=CARTESIAN_POINT('Ctrl Pts',(3.69192525052887,2.53927491555576,4.43314855508051));
#16477=CARTESIAN_POINT('Ctrl Pts',(3.6458997393802,2.56965301869642,4.43685315143278));
#16478=CARTESIAN_POINT('Ctrl Pts',(3.58332646905877,2.57495977187817,4.44055774778505));
#16479=CARTESIAN_POINT('Ctrl Pts',(3.5328424463163,2.55276653418389,4.44426234413732));
#16480=CARTESIAN_POINT('Ctrl Pts',(3.48235842357382,2.53057329648961,4.44796694048958));
#16481=CARTESIAN_POINT('Ctrl Pts',(3.4439636484103,2.4808800679193,4.45167153684185));
#16482=CARTESIAN_POINT('Ctrl Pts',(3.43522971000183,2.42642922394017,4.45537613319412));
#16483=CARTESIAN_POINT('Ctrl Pts',(3.43383723324577,2.41774797030146,4.45596676757575));
#16484=CARTESIAN_POINT('Ctrl Pts',(3.43319870043454,2.40894578361697,4.45655740195739));
#16485=CARTESIAN_POINT('Ctrl Pts',(3.43327529856389,2.40013247750357,4.45714803633902));
#16486=CARTESIAN_POINT('Origin',(3.6,2.4,4.7));
#16487=CARTESIAN_POINT('',(3.43366207255012,2.4000380247868,4.52714803633902));
#16488=CARTESIAN_POINT('',(3.43350143198867,2.39985687063426,4.50785196366098));
#16489=CARTESIAN_POINT('',(3.4334,2.4,4.7));
#16490=CARTESIAN_POINT('Ctrl Pts',(3.43350143198867,2.39985687063426,4.50785196366098));
#16491=CARTESIAN_POINT('Ctrl Pts',(3.43382054827219,2.43880728393095,4.50525071011481));
#16492=CARTESIAN_POINT('Ctrl Pts',(3.44745633991989,2.47795898515992,4.50264945656865));
#16493=CARTESIAN_POINT('Ctrl Pts',(3.47241574712106,2.50756395301054,4.50004820302248));
#16494=CARTESIAN_POINT('Ctrl Pts',(3.50796188948324,2.54972610827987,4.49634360667021));
#16495=CARTESIAN_POINT('Ctrl Pts',(3.56647488720154,2.57252532742787,4.49263901031794));
#16496=CARTESIAN_POINT('Ctrl Pts',(3.62117593737884,2.56552741635789,4.48893441396567));
#16497=CARTESIAN_POINT('Ctrl Pts',(3.67587698755613,2.55852950528791,4.4852298176134));
#16498=CARTESIAN_POINT('Ctrl Pts',(3.72676609019243,2.52173446399995,4.48152522126113));
#16499=CARTESIAN_POINT('Ctrl Pts',(3.75055355430056,2.47198175613265,4.47782062490887));
#16500=CARTESIAN_POINT('Ctrl Pts',(3.77434101840868,2.42222904826535,4.4741160285566));
#16501=CARTESIAN_POINT('Ctrl Pts',(3.77102684398863,2.3595186738187,4.47041143220433));
#16502=CARTESIAN_POINT('Ctrl Pts',(3.74212779097605,2.31255038253853,4.46670683585206));
#16503=CARTESIAN_POINT('Ctrl Pts',(3.71322873796346,2.26558209125837,4.4630022394998));
#16504=CARTESIAN_POINT('Ctrl Pts',(3.65874480635833,2.23435588314469,4.45929764314753));
#16505=CARTESIAN_POINT('Ctrl Pts',(3.60361085794536,2.23316262684763,4.45559304679526));
#16506=CARTESIAN_POINT('Ctrl Pts',(3.54847690953239,2.23196937055057,4.45188845044299));
#16507=CARTESIAN_POINT('Ctrl Pts',(3.49269294431159,2.26080906607012,4.44818385409072));
#16508=CARTESIAN_POINT('Ctrl Pts',(3.46178884724144,2.30648302829723,4.44447925773845));
#16509=CARTESIAN_POINT('Ctrl Pts',(3.44336034023669,2.33371899416048,4.44227015971263));
#16510=CARTESIAN_POINT('Ctrl Pts',(3.43377883797438,2.36694103826561,4.44006106168681));
#16511=CARTESIAN_POINT('Ctrl Pts',(3.43362892985438,2.40008323250784,4.43785196366098));
#16512=CARTESIAN_POINT('Ctrl Pts',(3.43327529856389,2.40013247750357,4.45714803633902));
#16513=CARTESIAN_POINT('Ctrl Pts',(3.43367914173529,2.35366667577227,4.46026199830965));
#16514=CARTESIAN_POINT('Ctrl Pts',(3.45396107839716,2.3068917935147,4.46337596028029));
#16515=CARTESIAN_POINT('Ctrl Pts',(3.48843309004669,2.27590093912579,4.46648992225093));
#16516=CARTESIAN_POINT('Ctrl Pts',(3.52944351015346,2.23903195767851,4.47019451860319));
#16517=CARTESIAN_POINT('Ctrl Pts',(3.59053745202041,2.22450245417194,4.47389911495546));
#16518=CARTESIAN_POINT('Ctrl Pts',(3.64375492737657,2.23896193518984,4.47760371130773));
#16519=CARTESIAN_POINT('Ctrl Pts',(3.69697240273272,2.25342141620775,4.48130830765999));
#16520=CARTESIAN_POINT('Ctrl Pts',(3.74231341157808,2.29686988175014,4.48501290401227));
#16521=CARTESIAN_POINT('Ctrl Pts',(3.75902738378866,2.34942289673192,4.48871750036453));
#16522=CARTESIAN_POINT('Ctrl Pts',(3.77574135599923,2.40197591171369,4.4924220967168));
#16523=CARTESIAN_POINT('Ctrl Pts',(3.76382829157503,2.46363347613485,4.49612669306907));
#16524=CARTESIAN_POINT('Ctrl Pts',(3.7287402721637,2.50617765524692,4.49983128942134));
#16525=CARTESIAN_POINT('Ctrl Pts',(3.69365225275236,2.54872183435899,4.5035358857736));
#16526=CARTESIAN_POINT('Ctrl Pts',(3.63538927835389,2.57215262816197,4.50724048212587));
#16527=CARTESIAN_POINT('Ctrl Pts',(3.58061572949426,2.56574680139426,4.51094507847814));
#16528=CARTESIAN_POINT('Ctrl Pts',(3.52584218063463,2.55934097462656,4.51464967483041));
#16529=CARTESIAN_POINT('Ctrl Pts',(3.47455805731385,2.52309852728818,4.51835427118268));
#16530=CARTESIAN_POINT('Ctrl Pts',(3.45023382941089,2.47360602072044,4.52205886753494));
#16531=CARTESIAN_POINT('Ctrl Pts',(3.43909540477512,2.45094266808951,4.5237552571363));
#16532=CARTESIAN_POINT('Ctrl Pts',(3.43361009249165,2.42550096367579,4.52545164673766));
#16533=CARTESIAN_POINT('Ctrl Pts',(3.43366207255012,2.4000380247868,4.52714803633902));
#16534=CARTESIAN_POINT('Origin',(3.6,2.4,4.7));
#16535=CARTESIAN_POINT('',(3.43341474631901,2.39984765669014,4.59714803633902));
#16536=CARTESIAN_POINT('',(3.43312356359968,2.40000067112034,4.57785196366098));
#16537=CARTESIAN_POINT('',(3.4334,2.4,4.7));
#16538=CARTESIAN_POINT('Ctrl Pts',(3.43312356496403,2.40000067111703,4.57785196366098));
#16539=CARTESIAN_POINT('Ctrl Pts',(3.43312026903532,2.45518344011976,4.57414495489509));
#16540=CARTESIAN_POINT('Ctrl Pts',(3.46320502523792,2.51036311996034,4.5704379461292));
#16541=CARTESIAN_POINT('Ctrl Pts',(3.50958660620738,2.54026105638185,4.5667309373633));
#16542=CARTESIAN_POINT('Ctrl Pts',(3.55593800339121,2.57013953609479,4.56302634101103));
#16543=CARTESIAN_POINT('Ctrl Pts',(3.6185650095987,2.57476916693782,4.55932174465876));
#16544=CARTESIAN_POINT('Ctrl Pts',(3.66880602035543,2.55203117207009,4.55561714830649));
#16545=CARTESIAN_POINT('Ctrl Pts',(3.71904703111215,2.52929317720236,4.55191255195423));
#16546=CARTESIAN_POINT('Ctrl Pts',(3.7569020464181,2.47918755662387,4.54820795560196));
#16547=CARTESIAN_POINT('Ctrl Pts',(3.76504650379449,2.42464543177811,4.54450335924969));
#16548=CARTESIAN_POINT('Ctrl Pts',(3.77319096117088,2.37010330693235,4.54079876289743));
#16549=CARTESIAN_POINT('Ctrl Pts',(3.75162486061771,2.31112467781931,4.53709416654516));
#16550=CARTESIAN_POINT('Ctrl Pts',(3.71021805048437,2.27470144834891,4.53338957019289));
#16551=CARTESIAN_POINT('Ctrl Pts',(3.66881124035102,2.23827821887852,4.52968497384062));
#16552=CARTESIAN_POINT('Ctrl Pts',(3.60756372063751,2.22441038905077,4.52598037748835));
#16553=CARTESIAN_POINT('Ctrl Pts',(3.55450576575121,2.23944465009304,4.52227578113609));
#16554=CARTESIAN_POINT('Ctrl Pts',(3.50144781086492,2.25447891113532,4.51857118478382));
#16555=CARTESIAN_POINT('Ctrl Pts',(3.45657942080584,2.29841526304761,4.51486658843155));
#16556=CARTESIAN_POINT('Ctrl Pts',(3.44043486927933,2.35114598469909,4.51116199207928));
#16557=CARTESIAN_POINT('Ctrl Pts',(3.43562652497117,2.36685081644385,4.51005864927318));
#16558=CARTESIAN_POINT('Ctrl Pts',(3.43336607622673,2.38333573667221,4.50895530646708));
#16559=CARTESIAN_POINT('Ctrl Pts',(3.43350143198867,2.39985687063426,4.50785196366098));
#16560=CARTESIAN_POINT('Ctrl Pts',(3.43366207255012,2.4000380247868,4.52714803633902));
#16561=CARTESIAN_POINT('Ctrl Pts',(3.43372360717887,2.36989468640869,4.52915624308993));
#16562=CARTESIAN_POINT('Ctrl Pts',(3.44154516635149,2.33972158979514,4.53116444984084));
#16563=CARTESIAN_POINT('Ctrl Pts',(3.45693460375181,2.31409281443648,4.53317265659175));
#16564=CARTESIAN_POINT('Ctrl Pts',(3.48532393848085,2.26681468051736,4.53687725294402));
#16565=CARTESIAN_POINT('Ctrl Pts',(3.53946694042407,2.23500097847622,4.54058184929629));
#16566=CARTESIAN_POINT('Ctrl Pts',(3.59458475774056,2.23321142940033,4.54428644564855));
#16567=CARTESIAN_POINT('Ctrl Pts',(3.64970257505705,2.23142188032444,4.54799104200082));
#16568=CARTESIAN_POINT('Ctrl Pts',(3.7057952077468,2.25965648421381,4.55169563835309));
#16569=CARTESIAN_POINT('Ctrl Pts',(3.73719154438744,2.30499351452124,4.55540023470536));
#16570=CARTESIAN_POINT('Ctrl Pts',(3.76858788102808,2.35033054482868,4.55910483105763));
#16571=CARTESIAN_POINT('Ctrl Pts',(3.77528792161962,2.41277000155418,4.56280942740989));
#16572=CARTESIAN_POINT('Ctrl Pts',(3.75422535459604,2.4637361132596,4.56651402376216));
#16573=CARTESIAN_POINT('Ctrl Pts',(3.73316278757246,2.51470222496502,4.57021862011443));
#16574=CARTESIAN_POINT('Ctrl Pts',(3.68433761293377,2.55419499165036,4.5739232164667));
#16575=CARTESIAN_POINT('Ctrl Pts',(3.63009494870967,2.56414032470881,4.57762781281897));
#16576=CARTESIAN_POINT('Ctrl Pts',(3.57585228448556,2.57408565776726,4.58133240917124));
#16577=CARTESIAN_POINT('Ctrl Pts',(3.51619213067606,2.55448355719882,4.5850370055235));
#16578=CARTESIAN_POINT('Ctrl Pts',(3.47841829496877,2.51430503547713,4.58874160187577));
#16579=CARTESIAN_POINT('Ctrl Pts',(3.44984628656769,2.48391413027303,4.59154374669685));
#16580=CARTESIAN_POINT('Ctrl Pts',(3.43379623122065,2.44175071136891,4.59434589151794));
#16581=CARTESIAN_POINT('Ctrl Pts',(3.43341474631901,2.39984765669014,4.59714803633902));
#16582=CARTESIAN_POINT('Origin',(3.6,2.4,4.7));
#16583=CARTESIAN_POINT('',(3.43314571939013,2.4000550352968,4.66714803633902));
#16584=CARTESIAN_POINT('',(3.43350338992805,2.40014270746267,4.64785196366098));
#16585=CARTESIAN_POINT('',(3.4334,2.4,4.7));
#16586=CARTESIAN_POINT('Ctrl Pts',(3.43350338992805,2.40014270746267,4.64785196366098));
#16587=CARTESIAN_POINT('Ctrl Pts',(3.43336795942281,2.41673658085083,4.64674379602763));
#16588=CARTESIAN_POINT('Ctrl Pts',(3.43564861639563,2.43329406542932,4.64563562839428));
#16589=CARTESIAN_POINT('Ctrl Pts',(3.44049847652216,2.44906128539828,4.64452746076093));
#16590=CARTESIAN_POINT('Ctrl Pts',(3.45671152371201,2.5017709872742,4.64082286440866));
#16591=CARTESIAN_POINT('Ctrl Pts',(3.5016369588364,2.54564900761994,4.63711826805639));
#16592=CARTESIAN_POINT('Ctrl Pts',(3.55471440176584,2.56061432161925,4.63341367170412));
#16593=CARTESIAN_POINT('Ctrl Pts',(3.60779184469527,2.57557963561855,4.62970907535186));
#16594=CARTESIAN_POINT('Ctrl Pts',(3.66902129542974,2.56163224327142,4.62600447899959));
#16595=CARTESIAN_POINT('Ctrl Pts',(3.71038074864658,2.52515524777208,4.62229988264732));
#16596=CARTESIAN_POINT('Ctrl Pts',(3.75174020186341,2.48867825227274,4.61859528629505));
#16597=CARTESIAN_POINT('Ctrl Pts',(3.77322965756262,2.42967165362121,4.61489068994278));
#16598=CARTESIAN_POINT('Ctrl Pts',(3.76501434448883,2.37514015628156,4.61118609359052));
#16599=CARTESIAN_POINT('Ctrl Pts',(3.75679903141505,2.32060865894192,4.60748149723825));
#16600=CARTESIAN_POINT('Ctrl Pts',(3.71887894956827,2.27055226291416,4.60377690088598));
#16601=CARTESIAN_POINT('Ctrl Pts',(3.6686084394294,2.24787956167738,4.60007230453371));
#16602=CARTESIAN_POINT('Ctrl Pts',(3.61833792929053,2.22520686044059,4.59636770818145));
#16603=CARTESIAN_POINT('Ctrl Pts',(3.55571699085956,2.22991785399477,4.59266311182918));
#16604=CARTESIAN_POINT('Ctrl Pts',(3.50940445168984,2.2598565294309,4.58895851547691));
#16605=CARTESIAN_POINT('Ctrl Pts',(3.46312207100161,2.28977570895933,4.58525633153827));
#16606=CARTESIAN_POINT('Ctrl Pts',(3.43312685660295,2.34488972480058,4.58155414759962));
#16607=CARTESIAN_POINT('Ctrl Pts',(3.43312356496403,2.40000067111703,4.57785196366098));
#16608=CARTESIAN_POINT('Ctrl Pts',(3.43341474631901,2.39984765669014,4.59714803633902));
#16609=CARTESIAN_POINT('Ctrl Pts',(3.43329188627587,2.38635246701557,4.59805048787021));
#16610=CARTESIAN_POINT('Ctrl Pts',(3.43479418574107,2.37288428257405,4.59895293940139));
#16611=CARTESIAN_POINT('Ctrl Pts',(3.43802675467359,2.35984505096448,4.59985539093258));
#16612=CARTESIAN_POINT('Ctrl Pts',(3.45129656769075,2.30631853104845,4.60355998728484));
#16613=CARTESIAN_POINT('Ctrl Pts',(3.49372371133013,2.26002043409134,4.60726458363711));
#16614=CARTESIAN_POINT('Ctrl Pts',(3.54589116272705,2.24213934669288,4.61096917998938));
#16615=CARTESIAN_POINT('Ctrl Pts',(3.59805861412397,2.22425825929442,4.61467377634164));
#16616=CARTESIAN_POINT('Ctrl Pts',(3.65996637327845,2.23479418145462,4.61837837269391));
#16617=CARTESIAN_POINT('Ctrl Pts',(3.70328200317247,2.26892528865449,4.62208296904618));
#16618=CARTESIAN_POINT('Ctrl Pts',(3.7465976330665,2.30305639585435,4.62578756539845));
#16619=CARTESIAN_POINT('Ctrl Pts',(3.77132113370008,2.3607826880939,4.62949216175072));
#16620=CARTESIAN_POINT('Ctrl Pts',(3.76613765481651,2.41568540039916,4.63319675810299));
#16621=CARTESIAN_POINT('Ctrl Pts',(3.76095417593294,2.47058811270442,4.63690135445526));
#16622=CARTESIAN_POINT('Ctrl Pts',(3.72586371753223,2.5226672450754,4.64060595080753));
#16623=CARTESIAN_POINT('Ctrl Pts',(3.67692562687786,2.54808848727385,4.64431054715979));
#16624=CARTESIAN_POINT('Ctrl Pts',(3.6279875362235,2.5735097294723,4.64801514351206));
#16625=CARTESIAN_POINT('Ctrl Pts',(3.56520181331549,2.57227308149821,4.65171973986433));
#16626=CARTESIAN_POINT('Ctrl Pts',(3.51730270026196,2.54494450230916,4.65542433621659));
#16627=CARTESIAN_POINT('Ctrl Pts',(3.46940358720842,2.51761592312011,4.65912893256886));
#16628=CARTESIAN_POINT('Ctrl Pts',(3.43639108400936,2.46419541271609,4.66283352892113));
#16629=CARTESIAN_POINT('Ctrl Pts',(3.43337354994745,2.40913117059842,4.6665381252734));
#16630=CARTESIAN_POINT('Ctrl Pts',(3.43320795139183,2.40610931275893,4.66674142896194));
#16631=CARTESIAN_POINT('Ctrl Pts',(3.43313268806444,2.40308250452664,4.66694473265048));
#16632=CARTESIAN_POINT('Ctrl Pts',(3.43314571939013,2.4000550352968,4.66714803633902));
#16633=CARTESIAN_POINT('Origin',(3.6,2.4,4.7));
#16634=CARTESIAN_POINT('',(3.43357722762007,2.40011764662452,4.73714803633902));
#16635=CARTESIAN_POINT('',(3.43362781118013,2.39991574862771,4.71785196366098));
#16636=CARTESIAN_POINT('',(3.4334,2.4,4.7));
#16637=CARTESIAN_POINT('Ctrl Pts',(3.43362781118013,2.39991574862771,4.71785196366098));
#16638=CARTESIAN_POINT('Ctrl Pts',(3.4337799165104,2.43312978761853,4.71563804080791));
#16639=CARTESIAN_POINT('Ctrl Pts',(3.44340626416077,2.46642503117871,4.71342411795483));
#16640=CARTESIAN_POINT('Ctrl Pts',(3.46191047388993,2.49369647002616,4.71121019510175));
#16641=CARTESIAN_POINT('Ctrl Pts',(3.49287389602047,2.5393302520412,4.70750559874949));
#16642=CARTESIAN_POINT('Ctrl Pts',(3.54869526280824,2.56809742778931,4.70380100239722));
#16643=CARTESIAN_POINT('Ctrl Pts',(3.60382760921412,2.56683253616837,4.70009640604495));
#16644=CARTESIAN_POINT('Ctrl Pts',(3.65895995562,2.56556764454744,4.69639180969268));
#16645=CARTESIAN_POINT('Ctrl Pts',(3.71340328164399,2.53427068555747,4.69268721334041));
#16646=CARTESIAN_POINT('Ctrl Pts',(3.74224129041658,2.48726488994604,4.68898261698815));
#16647=CARTESIAN_POINT('Ctrl Pts',(3.77107929918916,2.44025909433461,4.68527802063588));
#16648=CARTESIAN_POINT('Ctrl Pts',(3.77431199071034,2.37754446210172,4.68157342428361));
#16649=CARTESIAN_POINT('Ctrl Pts',(3.75045990537481,2.32782270030492,4.67786882793134));
#16650=CARTESIAN_POINT('Ctrl Pts',(3.72660782003928,2.27810093850813,4.67416423157907));
#16651=CARTESIAN_POINT('Ctrl Pts',(3.67567095784705,2.24137204714742,4.6704596352268));
#16652=CARTESIAN_POINT('Ctrl Pts',(3.62096086261208,2.23444521162098,4.66675503887454));
#16653=CARTESIAN_POINT('Ctrl Pts',(3.56625076737711,2.22751837609454,4.66305044252227));
#16654=CARTESIAN_POINT('Ctrl Pts',(3.5077674390994,2.25039359640236,4.65934584617));
#16655=CARTESIAN_POINT('Ctrl Pts',(3.4722761045882,2.29260189825932,4.65564124981774));
#16656=CARTESIAN_POINT('Ctrl Pts',(3.44740140531328,2.32218429717603,4.65304482109882));
#16657=CARTESIAN_POINT('Ctrl Pts',(3.43382070261849,2.36126338259659,4.6504483923799));
#16658=CARTESIAN_POINT('Ctrl Pts',(3.43350338992805,2.40014270746267,4.64785196366098));
#16659=CARTESIAN_POINT('Ctrl Pts',(3.43314571939013,2.4000550352968,4.66714803633902));
#16660=CARTESIAN_POINT('Ctrl Pts',(3.43337014465933,2.34791601174949,4.67064932900275));
#16661=CARTESIAN_POINT('Ctrl Pts',(3.45978247246013,2.29558093851357,4.67415062166648));
#16662=CARTESIAN_POINT('Ctrl Pts',(3.50195947903851,2.26495997488444,4.67765191433021));
#16663=CARTESIAN_POINT('Ctrl Pts',(3.54658550711625,2.23256099511944,4.68135651068247));
#16664=CARTESIAN_POINT('Ctrl Pts',(3.60886012819649,2.22447100942077,4.68506110703474));
#16665=CARTESIAN_POINT('Ctrl Pts',(3.66028300882075,2.24439244561677,4.68876570338701));
#16666=CARTESIAN_POINT('Ctrl Pts',(3.71170588944501,2.26431388181277,4.69247029973928));
#16667=CARTESIAN_POINT('Ctrl Pts',(3.75227702961328,2.31224673990343,4.69617489609154));
#16668=CARTESIAN_POINT('Ctrl Pts',(3.76342881697354,2.36625427558577,4.69987949244381));
#16669=CARTESIAN_POINT('Ctrl Pts',(3.7745806043338,2.42026181126811,4.70358408879608));
#16670=CARTESIAN_POINT('Ctrl Pts',(3.75631303888606,2.48034402454213,4.70728868514835));
#16671=CARTESIAN_POINT('Ctrl Pts',(3.71698637554161,2.51900394981365,4.71099328150062));
#16672=CARTESIAN_POINT('Ctrl Pts',(3.67765971219715,2.55766387508518,4.71469787785288));
#16673=CARTESIAN_POINT('Ctrl Pts',(3.617273950956,2.57490151235421,4.71840247420515));
#16674=CARTESIAN_POINT('Ctrl Pts',(3.5634649778607,2.56282795918052,4.72210707055742));
#16675=CARTESIAN_POINT('Ctrl Pts',(3.50965600476541,2.55075440600683,4.72581166690969));
#16676=CARTESIAN_POINT('Ctrl Pts',(3.46242381981598,2.50936966239043,4.72951626326196));
#16677=CARTESIAN_POINT('Ctrl Pts',(3.44338450027923,2.45761369091481,4.73322085961423));
#16678=CARTESIAN_POINT('Ctrl Pts',(3.43665675223952,2.43932516253718,4.73452991852249));
#16679=CARTESIAN_POINT('Ctrl Pts',(3.43344927286167,2.41974164310833,4.73583897743076));
#16680=CARTESIAN_POINT('Ctrl Pts',(3.43357722762007,2.40011764662452,4.73714803633902));
#16681=CARTESIAN_POINT('Origin',(3.6,2.4,4.7));
#16682=CARTESIAN_POINT('',(3.4335708769619,2.39987935507417,4.80714803633902));
#16683=CARTESIAN_POINT('',(3.43319592025803,2.39990252619761,4.78785196366098));
#16684=CARTESIAN_POINT('',(3.4334,2.4,4.7));
#16685=CARTESIAN_POINT('Ctrl Pts',(3.43319592025803,2.39990252619761,4.78785196366098));
#16686=CARTESIAN_POINT('Ctrl Pts',(3.43353981667182,2.44937640878962,4.78453228558818));
#16687=CARTESIAN_POINT('Ctrl Pts',(3.45695303934336,2.49913297337583,4.78121260751538));
#16688=CARTESIAN_POINT('Ctrl Pts',(3.495475201044,2.5300857875399,4.77789292944258));
#16689=CARTESIAN_POINT('Ctrl Pts',(3.5384640260409,2.56462759548935,4.77418833309031));
#16690=CARTESIAN_POINT('Ctrl Pts',(3.60026870000874,2.57575223778946,4.77048373673805));
#16691=CARTESIAN_POINT('Ctrl Pts',(3.6526039634498,2.55836845881058,4.76677914038578));
#16692=CARTESIAN_POINT('Ctrl Pts',(3.70493922689085,2.54098467983171,4.76307454403351));
#16693=CARTESIAN_POINT('Ctrl Pts',(3.74780507980512,2.49509247957384,4.75936994768124));
#16694=CARTESIAN_POINT('Ctrl Pts',(3.76158372154047,2.44169468371147,4.75566535132897));
#16695=CARTESIAN_POINT('Ctrl Pts',(3.77536236327582,2.38829688784909,4.7519607549767));
#16696=CARTESIAN_POINT('Ctrl Pts',(3.76005379383226,2.32739349638222,4.74825615862444));
#16697=CARTESIAN_POINT('Ctrl Pts',(3.72266406682112,2.28685729176137,4.74455156227217));
#16698=CARTESIAN_POINT('Ctrl Pts',(3.68527433980998,2.24632108714052,4.7408469659199));
#16699=CARTESIAN_POINT('Ctrl Pts',(3.62580345523126,2.22615206936571,4.73714236956763));
#16700=CARTESIAN_POINT('Ctrl Pts',(3.57146860063526,2.23558070378767,4.73343777321536));
#16701=CARTESIAN_POINT('Ctrl Pts',(3.51713374603927,2.24500933820964,4.72973317686309));
#16702=CARTESIAN_POINT('Ctrl Pts',(3.467934921426,2.28403562482839,4.72602858051083));
#16703=CARTESIAN_POINT('Ctrl Pts',(3.44638824785603,2.33479896227876,4.72232398415856));
#16704=CARTESIAN_POINT('Ctrl Pts',(3.43771819254303,2.35522536091232,4.72083331065937));
#16705=CARTESIAN_POINT('Ctrl Pts',(3.43352539596517,2.37755214744982,4.71934263716017));
#16706=CARTESIAN_POINT('Ctrl Pts',(3.43362781118013,2.39991574862771,4.71785196366098));
#16707=CARTESIAN_POINT('Ctrl Pts',(3.43357722762007,2.40011764662452,4.73714803633902));
#16708=CARTESIAN_POINT('Ctrl Pts',(3.4338113808831,2.36420633806453,4.73954357378302));
#16709=CARTESIAN_POINT('Ctrl Pts',(3.44521519316665,2.32815948046248,4.74193911122703));
#16710=CARTESIAN_POINT('Ctrl Pts',(3.46665596573275,2.29966495797107,4.74433464867103));
#16711=CARTESIAN_POINT('Ctrl Pts',(3.49981320484709,2.25559939583779,4.7480392450233));
#16712=CARTESIAN_POINT('Ctrl Pts',(3.55697413719987,2.22959547090607,4.75174384137556));
#16713=CARTESIAN_POINT('Ctrl Pts',(3.61197873797528,2.23355402687319,4.75544843772783));
#16714=CARTESIAN_POINT('Ctrl Pts',(3.6669833387507,2.2375125828403,4.7591530340801));
#16715=CARTESIAN_POINT('Ctrl Pts',(3.71983160794876,2.27143361970626,4.76285763043237));
#16716=CARTESIAN_POINT('Ctrl Pts',(3.74633723550091,2.31979298260399,4.76656222678464));
#16717=CARTESIAN_POINT('Ctrl Pts',(3.77284286305306,2.36815234550172,4.7702668231369));
#16718=CARTESIAN_POINT('Ctrl Pts',(3.77300584895929,2.43095003443123,4.77397141948917));
#16719=CARTESIAN_POINT('Ctrl Pts',(3.74675160179543,2.47944633096681,4.77767601584144));
#16720=CARTESIAN_POINT('Ctrl Pts',(3.72049735463157,2.52794262750239,4.78138061219371));
#16721=CARTESIAN_POINT('Ctrl Pts',(3.66782587439761,2.56213753164403,4.78508520854598));
#16722=CARTESIAN_POINT('Ctrl Pts',(3.61284256269023,2.56638155161303,4.78878980489825));
#16723=CARTESIAN_POINT('Ctrl Pts',(3.55785925098286,2.57062557158203,4.79249440125052));
#16724=CARTESIAN_POINT('Ctrl Pts',(3.50056410780207,2.54491870737838,4.79619899760278));
#16725=CARTESIAN_POINT('Ctrl Pts',(3.4671785803101,2.50102585117272,4.79990359395505));
#16726=CARTESIAN_POINT('Ctrl Pts',(3.44541646757448,2.47241461280706,4.80231840808304));
#16727=CARTESIAN_POINT('Ctrl Pts',(3.43381352470784,2.43607616609189,4.80473322221103));
#16728=CARTESIAN_POINT('Ctrl Pts',(3.4335708769619,2.39987935507417,4.80714803633902));
#16729=CARTESIAN_POINT('Origin',(3.6,2.4,4.7));
#16730=CARTESIAN_POINT('',(3.43314188794433,2.3999499425809,4.87714803633902));
#16731=CARTESIAN_POINT('',(3.43333250203974,2.40014587505553,4.85785196366098));
#16732=CARTESIAN_POINT('',(3.4334,2.4,4.7));
#16733=CARTESIAN_POINT('Ctrl Pts',(3.43333250203974,2.40014587505553,4.85785196366098));
#16734=CARTESIAN_POINT('Ctrl Pts',(3.43323383740233,2.41091157669441,4.85713112672073));
#16735=CARTESIAN_POINT('Ctrl Pts',(3.43418764294185,2.42165986991066,4.85641028978047));
#16736=CARTESIAN_POINT('Ctrl Pts',(3.43625743346387,2.43218878097762,4.85568945284021));
#16737=CARTESIAN_POINT('Ctrl Pts',(3.44689470520955,2.48629999996998,4.85198485648794));
#16738=CARTESIAN_POINT('Ctrl Pts',(3.48700780884227,2.53461681182183,4.84828026013567));
#16739=CARTESIAN_POINT('Ctrl Pts',(3.53823875502779,2.55502675361418,4.8445756637834));
#16740=CARTESIAN_POINT('Ctrl Pts',(3.58946970121331,2.57543669540653,4.84087106743113));
#16741=CARTESIAN_POINT('Ctrl Pts',(3.65181848995162,2.56793976713939,4.83716647107887));
#16742=CARTESIAN_POINT('Ctrl Pts',(3.69675084453495,2.5359669805447,4.8334618747266));
#16743=CARTESIAN_POINT('Ctrl Pts',(3.74168319911827,2.50399419395,4.82975727837433));
#16744=CARTESIAN_POINT('Ctrl Pts',(3.7691991195466,2.44754554902777,4.82605268202206));
#16745=CARTESIAN_POINT('Ctrl Pts',(3.76670578881005,2.39245508821223,4.8223480856698));
#16746=CARTESIAN_POINT('Ctrl Pts',(3.7642124580735,2.33736462739668,4.81864348931753));
#16747=CARTESIAN_POINT('Ctrl Pts',(3.73170987617206,2.28363235068783,4.81493889296526));
#16748=CARTESIAN_POINT('Ctrl Pts',(3.68407303401509,2.25584913920422,4.811234296613));
#16749=CARTESIAN_POINT('Ctrl Pts',(3.63643619185813,2.2280659277206,4.80752970026073));
#16750=CARTESIAN_POINT('Ctrl Pts',(3.57366508944564,2.22623178146222,4.80382510390846));
#16751=CARTESIAN_POINT('Ctrl Pts',(3.52448727773306,2.25118610786454,4.80012050755619));
#16752=CARTESIAN_POINT('Ctrl Pts',(3.47530946602049,2.27614043426686,4.79641591120392));
#16753=CARTESIAN_POINT('Ctrl Pts',(3.43972494500783,2.32788323332987,4.79271131485165));
#16754=CARTESIAN_POINT('Ctrl Pts',(3.43401917251448,2.38273411966077,4.78900671849938));
#16755=CARTESIAN_POINT('Ctrl Pts',(3.43342632624397,2.38843328545001,4.78862180021992));
#16756=CARTESIAN_POINT('Ctrl Pts',(3.43315604530238,2.39416600556269,4.78823688194045));
#16757=CARTESIAN_POINT('Ctrl Pts',(3.43319592025803,2.39990252619761,4.78785196366098));
#16758=CARTESIAN_POINT('Ctrl Pts',(3.4335708769619,2.39987935507417,4.80714803633902));
#16759=CARTESIAN_POINT('Ctrl Pts',(3.43344127578645,2.38054618864739,4.8084378185633));
#16760=CARTESIAN_POINT('Ctrl Pts',(3.43655249507166,2.36125342749717,4.80972760078758));
#16761=CARTESIAN_POINT('Ctrl Pts',(3.44308754966948,2.34320004344294,4.81101738301185));
#16762=CARTESIAN_POINT('Ctrl Pts',(3.46185795832395,2.2913459401265,4.81472197936412));
#16763=CARTESIAN_POINT('Ctrl Pts',(3.50887468743604,2.24971658170129,4.81842657571639));
#16764=CARTESIAN_POINT('Ctrl Pts',(3.5626202643246,2.23736388010515,4.82213117206866));
#16765=CARTESIAN_POINT('Ctrl Pts',(3.61636584121316,2.22501117850901,4.82583576842092));
#16766=CARTESIAN_POINT('Ctrl Pts',(3.6768402658782,2.24193513374194,4.82954036477319));
#16767=CARTESIAN_POINT('Ctrl Pts',(3.71636707495845,2.28039040172619,4.83324496112546));
#16768=CARTESIAN_POINT('Ctrl Pts',(3.7558938840387,2.31884566971043,4.83694955747773));
#16769=CARTESIAN_POINT('Ctrl Pts',(3.77447307753417,2.378832250446,4.84065415383));
#16770=CARTESIAN_POINT('Ctrl Pts',(3.76360178219044,2.4328969451123,4.84435875018227));
#16771=CARTESIAN_POINT('Ctrl Pts',(3.75273048684672,2.4869616397786,4.84806334653454));
#16772=CARTESIAN_POINT('Ctrl Pts',(3.71240870266382,2.53510444837563,4.8517679428868));
#16773=CARTESIAN_POINT('Ctrl Pts',(3.66108992281312,2.55529254156049,4.85547253923907));
#16774=CARTESIAN_POINT('Ctrl Pts',(3.60977114296242,2.57548063474534,4.85917713559134));
#16775=CARTESIAN_POINT('Ctrl Pts',(3.54745536744392,2.56771401251802,4.86288173194361));
#16776=CARTESIAN_POINT('Ctrl Pts',(3.50266176427811,2.53554711358097,4.86658632829587));
#16777=CARTESIAN_POINT('Ctrl Pts',(3.46009329762648,2.50497811560107,4.87010689764359));
#16778=CARTESIAN_POINT('Ctrl Pts',(3.43334940270065,2.45237281292388,4.87362746699131));
#16779=CARTESIAN_POINT('Ctrl Pts',(3.43314188794433,2.3999499425809,4.87714803633902));
#16780=CARTESIAN_POINT('Origin',(3.6,2.4,4.7));
#16781=CARTESIAN_POINT('',(3.43342338863395,2.40015219044389,4.94714803633902));
#16782=CARTESIAN_POINT('',(3.4336698690944,2.40000633253548,4.92785196366098));
#16783=CARTESIAN_POINT('',(3.4334,2.4,4.7));
#16784=CARTESIAN_POINT('Ctrl Pts',(3.4336698690944,2.40000633253548,4.92785196366098));
#16785=CARTESIAN_POINT('Ctrl Pts',(3.43366057242126,2.42742681740845,4.926025371501));
#16786=CARTESIAN_POINT('Ctrl Pts',(3.44006468394764,2.45484321422969,4.92419877934102));
#16787=CARTESIAN_POINT('Ctrl Pts',(3.4529060499396,2.47881063108511,4.92237218718104));
#16788=CARTESIAN_POINT('Ctrl Pts',(3.47895022041959,2.52742006180595,4.91866759082877));
#16789=CARTESIAN_POINT('Ctrl Pts',(3.53147325119262,2.5618425345377,4.9149629944765));
#16790=CARTESIAN_POINT('Ctrl Pts',(3.58643767940152,2.56632440944362,4.91125839812423));
#16791=CARTESIAN_POINT('Ctrl Pts',(3.64140210761043,2.57080628434953,4.90755380177196));
#16792=CARTESIAN_POINT('Ctrl Pts',(3.6988079332552,2.54534756142961,4.90384920541969));
#16793=CARTESIAN_POINT('Ctrl Pts',(3.73238305471537,2.50159956959011,4.90014460906743));
#16794=CARTESIAN_POINT('Ctrl Pts',(3.76595817617555,2.45785157775061,4.89644001271516));
#16795=CARTESIAN_POINT('Ctrl Pts',(3.77570259345112,2.39581431699153,4.89273541636289));
#16796=CARTESIAN_POINT('Ctrl Pts',(3.75715671872181,2.34387949147388,4.88903082001062));
#16797=CARTESIAN_POINT('Ctrl Pts',(3.7386108439925,2.29194466595622,4.88532622365836));
#16798=CARTESIAN_POINT('Ctrl Pts',(3.6917746772583,2.25011227567998,4.88162162730609));
#16799=CARTESIAN_POINT('Ctrl Pts',(3.638083055804,2.23752715126117,4.87791703095382));
#16800=CARTESIAN_POINT('Ctrl Pts',(3.58439143434971,2.22494202684235,4.87421243460155));
#16801=CARTESIAN_POINT('Ctrl Pts',(3.52384435817533,2.24160416828095,4.87050783824928));
#16802=CARTESIAN_POINT('Ctrl Pts',(3.48415154001745,2.27988805206668,4.86680324189701));
#16803=CARTESIAN_POINT('Ctrl Pts',(3.45218211379499,2.3107226930672,4.863819482485));
#16804=CARTESIAN_POINT('Ctrl Pts',(3.43374090444541,2.35558342022287,4.86083572307299));
#16805=CARTESIAN_POINT('Ctrl Pts',(3.43333250203974,2.40014587505553,4.85785196366098));
#16806=CARTESIAN_POINT('Ctrl Pts',(3.43314188794433,2.3999499425809,4.87714803633902));
#16807=CARTESIAN_POINT('Ctrl Pts',(3.43313104074456,2.39720969722669,4.87733206334358));
#16808=CARTESIAN_POINT('Ctrl Pts',(3.43319270038641,2.39446995034259,4.87751609034813));
#16809=CARTESIAN_POINT('Ctrl Pts',(3.43332839678999,2.39173387533235,4.87770011735268));
#16810=CARTESIAN_POINT('Ctrl Pts',(3.43606006328079,2.33665471166754,4.88140471370495));
#16811=CARTESIAN_POINT('Ctrl Pts',(3.4687948270755,2.28306355998471,4.88510931005722));
#16812=CARTESIAN_POINT('Ctrl Pts',(3.5165514379046,2.2554867147355,4.88881390640948));
#16813=CARTESIAN_POINT('Ctrl Pts',(3.5643080487337,2.2279098694863,4.89251850276175));
#16814=CARTESIAN_POINT('Ctrl Pts',(3.6270865065972,2.22634733067072,4.89622309911402));
#16815=CARTESIAN_POINT('Ctrl Pts',(3.67615589427605,2.25151420303488,4.89992769546629));
#16816=CARTESIAN_POINT('Ctrl Pts',(3.72522528195491,2.27668107539905,4.90363229181856));
#16817=CARTESIAN_POINT('Ctrl Pts',(3.76058559944912,2.32857735894297,4.90733688817082));
#16818=CARTESIAN_POINT('Ctrl Pts',(3.76605399695032,2.38345242523688,4.91104148452309));
#16819=CARTESIAN_POINT('Ctrl Pts',(3.77152239445151,2.43832749153079,4.91474608087536));
#16820=CARTESIAN_POINT('Ctrl Pts',(3.74709887195967,2.4961813405747,4.91845067722763));
#16821=CARTESIAN_POINT('Ctrl Pts',(3.70396099303503,2.53053683028788,4.9221552735799));
#16822=CARTESIAN_POINT('Ctrl Pts',(3.66082311411038,2.56489232000106,4.92585986993216));
#16823=CARTESIAN_POINT('Ctrl Pts',(3.59897087875293,2.57574945038351,4.92956446628443));
#16824=CARTESIAN_POINT('Ctrl Pts',(3.54671131319796,2.55813939417591,4.9332690626367));
#16825=CARTESIAN_POINT('Ctrl Pts',(3.494451747643,2.5405293379683,4.93697365898897));
#16826=CARTESIAN_POINT('Ctrl Pts',(3.45178485189053,2.49445209517064,4.94067825534124));
#16827=CARTESIAN_POINT('Ctrl Pts',(3.43823737272355,2.44099517717631,4.94438285169351));
#16828=CARTESIAN_POINT('Ctrl Pts',(3.43486666978988,2.42769474038747,4.94530457990868));
#16829=CARTESIAN_POINT('Ctrl Pts',(3.43329859706143,2.41393746665015,4.94622630812385));
#16830=CARTESIAN_POINT('Ctrl Pts',(3.43342338863395,2.40015219044389,4.94714803633902));
#16831=CARTESIAN_POINT('Origin',(3.6,2.4,4.7));
#16832=CARTESIAN_POINT('',(3.43365998372879,2.39995738785189,5.01714803633902));
#16833=CARTESIAN_POINT('',(3.43335574706359,2.39985083704977,4.99785196366098));
#16834=CARTESIAN_POINT('',(3.4334,2.4,4.7));
#16835=CARTESIAN_POINT('Ctrl Pts',(3.43335574706359,2.39985083704977,4.99785196366098));
#16836=CARTESIAN_POINT('Ctrl Pts',(3.43376006251615,2.44366117078388,4.99491961628127));
#16837=CARTESIAN_POINT('Ctrl Pts',(3.45150379085869,2.48776127159334,4.99198726890157));
#16838=CARTESIAN_POINT('Ctrl Pts',(3.48249984106631,2.5184966596533,4.98905492152186));
#16839=CARTESIAN_POINT('Ctrl Pts',(3.52165886271855,2.55732637242214,4.98535032516959));
#16840=CARTESIAN_POINT('Ctrl Pts',(3.58196946998821,2.57482511625956,4.98164572881732));
#16841=CARTESIAN_POINT('Ctrl Pts',(3.63583017159909,2.56298449167174,4.97794113246505));
#16842=CARTESIAN_POINT('Ctrl Pts',(3.68969087320997,2.55114386708391,4.97423653611278));
#16843=CARTESIAN_POINT('Ctrl Pts',(3.73710166916209,2.50996387407084,4.97053193976052));
#16844=CARTESIAN_POINT('Ctrl Pts',(3.75636473978792,2.45829077001732,4.96682734340825));
#16845=CARTESIAN_POINT('Ctrl Pts',(3.77562781041376,2.4066176659638,4.96312274705598));
#16846=CARTESIAN_POINT('Ctrl Pts',(3.76674315571332,2.34445145086982,4.95941815070371));
#16847=CARTESIAN_POINT('Ctrl Pts',(3.73377688832091,2.30024284554165,4.95571355435145));
#16848=CARTESIAN_POINT('Ctrl Pts',(3.70081062092849,2.25603424021347,4.95200895799918));
#16849=CARTESIAN_POINT('Ctrl Pts',(3.64376274084411,2.2297832446511,4.94830436164691));
#16850=CARTESIAN_POINT('Ctrl Pts',(3.58874153385625,2.23350377584586,4.94459976529464));
#16851=CARTESIAN_POINT('Ctrl Pts',(3.5337203268684,2.23722430704061,4.94089516894238));
#16852=CARTESIAN_POINT('Ctrl Pts',(3.48072579297707,2.2709163649925,4.93719057259011));
#16853=CARTESIAN_POINT('Ctrl Pts',(3.45401118112487,2.31916058832341,4.93348597623784));
#16854=CARTESIAN_POINT('Ctrl Pts',(3.44046850379027,2.34361746433734,4.93160797204555));
#16855=CARTESIAN_POINT('Ctrl Pts',(3.43367942743562,2.37181405914562,4.92972996785326));
#16856=CARTESIAN_POINT('Ctrl Pts',(3.4336698690944,2.40000633253548,4.92785196366098));
#16857=CARTESIAN_POINT('Ctrl Pts',(3.43342338863395,2.40015219044389,4.94714803633902));
#16858=CARTESIAN_POINT('Ctrl Pts',(3.43380015749623,2.35853188927053,4.94993090447612));
#16859=CARTESIAN_POINT('Ctrl Pts',(3.44960819526551,2.31665633218087,4.95271377261321));
#16860=CARTESIAN_POINT('Ctrl Pts',(3.47782659951237,2.28632760954166,4.95549664075031));
#16861=CARTESIAN_POINT('Ctrl Pts',(3.51539136804964,2.24595355309232,4.95920123710258));
#16862=CARTESIAN_POINT('Ctrl Pts',(3.57494896770565,2.22604203338462,4.96290583345485));
#16863=CARTESIAN_POINT('Ctrl Pts',(3.62924252529985,2.23570567012353,4.96661042980711));
#16864=CARTESIAN_POINT('Ctrl Pts',(3.68353608289404,2.24536930686244,4.97031502615938));
#16865=CARTESIAN_POINT('Ctrl Pts',(3.73256559842641,2.28460810004796,4.97401962251165));
#16866=CARTESIAN_POINT('Ctrl Pts',(3.75389243606413,2.33546419387067,4.97772421886392));
#16867=CARTESIAN_POINT('Ctrl Pts',(3.77521927370186,2.38632028769338,4.98142881521618));
#16868=CARTESIAN_POINT('Ctrl Pts',(3.76884343344493,2.44879368215328,4.98513341156845));
#16869=CARTESIAN_POINT('Ctrl Pts',(3.73768285480685,2.49429307324449,4.98883800792072));
#16870=CARTESIAN_POINT('Ctrl Pts',(3.70652227616876,2.5397924643357,4.99254260427299));
#16871=CARTESIAN_POINT('Ctrl Pts',(3.65057695914952,2.5683178520582,4.99624720062526));
#16872=CARTESIAN_POINT('Ctrl Pts',(3.59545059518146,2.56681443253905,4.99995179697753));
#16873=CARTESIAN_POINT('Ctrl Pts',(3.54032423121339,2.5653110130199,5.00365639332979));
#16874=CARTESIAN_POINT('Ctrl Pts',(3.4860168202965,2.5337787862591,5.00736098968206));
#16875=CARTESIAN_POINT('Ctrl Pts',(3.45738245724731,2.48664865149311,5.01106558603433));
#16876=CARTESIAN_POINT('Ctrl Pts',(3.44171119613527,2.4608548649544,5.01309306946923));
#16877=CARTESIAN_POINT('Ctrl Pts',(3.43372965048622,2.43038911757193,5.01512055290412));
#16878=CARTESIAN_POINT('Ctrl Pts',(3.43365998372879,2.39995738785189,5.01714803633902));
#16879=CARTESIAN_POINT('Origin',(3.6,2.4,4.7));
#16880=CARTESIAN_POINT('',(3.43326717741735,2.39986996798437,5.08714803633902));
#16881=CARTESIAN_POINT('',(3.43317938608394,2.40008640134203,5.06785196366098));
#16882=CARTESIAN_POINT('',(3.4334,2.4,4.7));
#16883=CARTESIAN_POINT('Ctrl Pts',(3.43317938608394,2.40008640134203,5.06785196366098));
#16884=CARTESIAN_POINT('Ctrl Pts',(3.43314802172115,2.40505542046622,5.06751845741382));
#16885=CARTESIAN_POINT('Ctrl Pts',(3.4333507965104,2.41002184414099,5.06718495116665));
#16886=CARTESIAN_POINT('Ctrl Pts',(3.43379604919982,2.41496643290483,5.06685144491949));
#16887=CARTESIAN_POINT('Ctrl Pts',(3.4387419280344,2.46989105771691,5.06314684856722));
#16888=CARTESIAN_POINT('Ctrl Pts',(3.47360673324676,2.52212151084356,5.05944225221496));
#16889=CARTESIAN_POINT('Ctrl Pts',(3.52243437289015,2.54775424884904,5.05573765586269));
#16890=CARTESIAN_POINT('Ctrl Pts',(3.57126201253354,2.57338698685451,5.05203305951042));
#16891=CARTESIAN_POINT('Ctrl Pts',(3.63405248660798,2.57242200973882,5.04832846315815));
#16892=CARTESIAN_POINT('Ctrl Pts',(3.68206938667054,2.54530093495911,5.04462386680588));
#16893=CARTESIAN_POINT('Ctrl Pts',(3.7300862867331,2.51817986017941,5.04091927045361));
#16894=CARTESIAN_POINT('Ctrl Pts',(3.7633296127838,2.4649026877357,5.03721467410135));
#16895=CARTESIAN_POINT('Ctrl Pts',(3.76658536412569,2.40985202258946,5.03351007774908));
#16896=CARTESIAN_POINT('Ctrl Pts',(3.76984111546757,2.35480135744323,5.02980548139681));
#16897=CARTESIAN_POINT('Ctrl Pts',(3.74310929210064,2.29797719959448,5.02610088504454));
#16898=CARTESIAN_POINT('Ctrl Pts',(3.69862386658003,2.26538544465498,5.02239628869227));
#16899=CARTESIAN_POINT('Ctrl Pts',(3.65413844105941,2.23279368971548,5.01869169234));
#16900=CARTESIAN_POINT('Ctrl Pts',(3.59189941338511,2.22443433768522,5.01498709598774));
#16901=CARTESIAN_POINT('Ctrl Pts',(3.54039082648689,2.24413309464159,5.01128249963547));
#16902=CARTESIAN_POINT('Ctrl Pts',(3.48888223958867,2.26383185159795,5.0075779032832));
#16903=CARTESIAN_POINT('Ctrl Pts',(3.44810409346653,2.31158871754094,5.00387330693093));
#16904=CARTESIAN_POINT('Ctrl Pts',(3.43671873842288,2.36554749136257,5.00016871057866));
#16905=CARTESIAN_POINT('Ctrl Pts',(3.43434538167935,2.37679557446855,4.9993964616061));
#16906=CARTESIAN_POINT('Ctrl Pts',(3.43324926848095,2.38831315722103,4.99862421263354));
#16907=CARTESIAN_POINT('Ctrl Pts',(3.43335574706359,2.39985083704977,4.99785196366098));
#16908=CARTESIAN_POINT('Ctrl Pts',(3.43365998372879,2.39995738785189,5.01714803633902));
#16909=CARTESIAN_POINT('Ctrl Pts',(3.43360235612169,2.37478458193251,5.01882514925639));
#16910=CARTESIAN_POINT('Ctrl Pts',(3.43895837147105,2.34963505233992,5.02050226217376));
#16911=CARTESIAN_POINT('Ctrl Pts',(3.44985377385385,2.32717237393524,5.02217937509113));
#16912=CARTESIAN_POINT('Ctrl Pts',(3.47392076869108,2.2775542739145,5.0258839714434));
#16913=CARTESIAN_POINT('Ctrl Pts',(3.52501607354704,2.24104611664418,5.02958856779567));
#16914=CARTESIAN_POINT('Ctrl Pts',(3.57975563349286,2.23435605471958,5.03329316414794));
#16915=CARTESIAN_POINT('Ctrl Pts',(3.63449519343869,2.22766599279499,5.03699776050021));
#16916=CARTESIAN_POINT('Ctrl Pts',(3.69287900847437,2.25079402621613,5.04070235685247));
#16917=CARTESIAN_POINT('Ctrl Pts',(3.72818739245021,2.2931555045654,5.04440695320474));
#16918=CARTESIAN_POINT('Ctrl Pts',(3.76349577642604,2.33551698291468,5.04811154955701));
#16919=CARTESIAN_POINT('Ctrl Pts',(3.77572872934203,2.39711190619209,5.05181614590928));
#16920=CARTESIAN_POINT('Ctrl Pts',(3.75928777521595,2.44975095798197,5.05552074226155));
#16921=CARTESIAN_POINT('Ctrl Pts',(3.74284682108988,2.50239000977184,5.05922533861381));
#16922=CARTESIAN_POINT('Ctrl Pts',(3.69773195992176,2.54607319007419,5.06292993496608));
#16923=CARTESIAN_POINT('Ctrl Pts',(3.64459025516192,2.56080874487665,5.06663453131835));
#16924=CARTESIAN_POINT('Ctrl Pts',(3.59144855040209,2.57554429967911,5.07033912767062));
#16925=CARTESIAN_POINT('Ctrl Pts',(3.53028000205055,2.5613322289817,5.07404372402289));
#16926=CARTESIAN_POINT('Ctrl Pts',(3.48907876029587,2.52467656495583,5.07774832037516));
#16927=CARTESIAN_POINT('Ctrl Pts',(3.45423196161424,2.49367428224656,5.08088155902978));
#16928=CARTESIAN_POINT('Ctrl Pts',(3.43366833435756,2.44661747113372,5.0840147976844));
#16929=CARTESIAN_POINT('Ctrl Pts',(3.43326717741735,2.39986996798437,5.08714803633902));
#16930=CARTESIAN_POINT('Origin',(3.6,2.4,4.7));
#16931=CARTESIAN_POINT('',(3.43325215340634,2.40012157034435,5.15714803633902));
#16932=CARTESIAN_POINT('',(3.43361558566414,2.40009421455432,5.13785196366098));
#16933=CARTESIAN_POINT('',(3.4334,2.4,4.7));
#16934=CARTESIAN_POINT('',(3.72690708798524,2.50793586530485,5.2));
#16935=CARTESIAN_POINT('Ctrl Pts',(3.43325215340634,2.40012157034435,5.15714803633902));
#16936=CARTESIAN_POINT('Ctrl Pts',(3.43364568326786,2.35284438105766,5.16031823516921));
#16937=CARTESIAN_POINT('Ctrl Pts',(3.45475449837728,2.3052683699281,5.1634884339994));
#16938=CARTESIAN_POINT('Ctrl Pts',(3.49032381108024,2.27424021130156,5.16665863282959));
#16939=CARTESIAN_POINT('Ctrl Pts',(3.53188901034701,2.23798166430732,5.17036322918186));
#16940=CARTESIAN_POINT('Ctrl Pts',(3.59320079576331,2.22432009870508,5.17406782553412));
#16941=CARTESIAN_POINT('Ctrl Pts',(3.64619138280368,2.2396150803554,5.17777242188639));
#16942=CARTESIAN_POINT('Ctrl Pts',(3.69918196984405,2.25491006200572,5.18147701823866));
#16943=CARTESIAN_POINT('Ctrl Pts',(3.74385135850849,2.2991615909086,5.18518161459093));
#16944=CARTESIAN_POINT('Ctrl Pts',(3.75975544882264,2.35186813523316,5.1888862109432));
#16945=CARTESIAN_POINT('Ctrl Pts',(3.7756595391368,2.40457467955771,5.19259080729547));
#16946=CARTESIAN_POINT('Ctrl Pts',(3.76279833110066,2.46573623930395,5.19629540364773));
#16947=CARTESIAN_POINT('Ctrl Pts',(3.72690708798524,2.50793586530485,5.2));
#16948=CARTESIAN_POINT('',(3.47285246768952,2.50812032770478,5.2));
#16949=CARTESIAN_POINT('Origin',(3.6,2.4,5.2));
#16950=CARTESIAN_POINT('Ctrl Pts',(3.47285231527688,2.50812044463164,5.2));
#16951=CARTESIAN_POINT('Ctrl Pts',(3.50793811173714,2.54927258268021,5.19636770818145));
#16952=CARTESIAN_POINT('Ctrl Pts',(3.56493587106976,2.57187757629771,5.19273541636289));
#16953=CARTESIAN_POINT('Ctrl Pts',(3.6186762488644,2.56581789998251,5.18910312454433));
#16954=CARTESIAN_POINT('Ctrl Pts',(3.67348638458382,2.55963759952907,5.18539852819207));
#16955=CARTESIAN_POINT('Ctrl Pts',(3.72490816491496,2.52364007082416,5.1816939318398));
#16956=CARTESIAN_POINT('Ctrl Pts',(3.74944162746499,2.4742589593754,5.17798933548753));
#16957=CARTESIAN_POINT('Ctrl Pts',(3.77397509001502,2.42487784792664,5.17428473913527));
#16958=CARTESIAN_POINT('Ctrl Pts',(3.77162023478396,2.36211315373403,5.17058014278299));
#16959=CARTESIAN_POINT('Ctrl Pts',(3.74343805908691,2.31470980295916,5.16687554643072));
#16960=CARTESIAN_POINT('Ctrl Pts',(3.71525588338986,2.2673064521843,5.16317095007846));
#16961=CARTESIAN_POINT('Ctrl Pts',(3.66124638722683,2.23526444482719,5.15946635372619));
#16962=CARTESIAN_POINT('Ctrl Pts',(3.60613566997566,2.23323785031625,5.15576175737392));
#16963=CARTESIAN_POINT('Ctrl Pts',(3.55102495272448,2.23121125580531,5.15205716102166));
#16964=CARTESIAN_POINT('Ctrl Pts',(3.49481301438516,2.25920007414054,5.14835256466939));
#16965=CARTESIAN_POINT('Ctrl Pts',(3.46322139831185,2.30440012642267,5.14464796831712));
#16966=CARTESIAN_POINT('Ctrl Pts',(3.44390334496103,2.33203964380033,5.14238263343174));
#16967=CARTESIAN_POINT('Ctrl Pts',(3.43379141454156,2.36611485011022,5.14011729854636));
#16968=CARTESIAN_POINT('Ctrl Pts',(3.43361558566414,2.40009421455432,5.13785196366098));
#16969=CARTESIAN_POINT('Origin',(3.6,2.4,5.35459252805377));
#16970=CARTESIAN_POINT('',(3.39427731514299,2.4001195557093,4.34540747194623));
#16971=CARTESIAN_POINT('',(3.39483887138702,2.39991986985508,4.33959252805377));
#16972=CARTESIAN_POINT('',(3.394525,2.40000000000001,5.35459252805377));
#16973=CARTESIAN_POINT('',(3.78826275096636,2.31767678198967,4.3));
#16974=CARTESIAN_POINT('Ctrl Pts',(3.39483887138702,2.39991986985508,4.33959252805377));
#16975=CARTESIAN_POINT('Ctrl Pts',(3.39495667746176,2.43847992884438,4.33750880775932));
#16976=CARTESIAN_POINT('Ctrl Pts',(3.42394163903792,2.54576387140554,4.3317204911126));
#16977=CARTESIAN_POINT('Ctrl Pts',(3.59702533363695,2.64299053446886,4.32222757811361));
#16978=CARTESIAN_POINT('Ctrl Pts',(3.80250223745458,2.5338839434383,4.3111137890568));
#16979=CARTESIAN_POINT('Ctrl Pts',(3.81563717950601,2.38027862564402,4.30370459635227));
#16980=CARTESIAN_POINT('Ctrl Pts',(3.78826275096636,2.31767678198967,4.3));
#16981=CARTESIAN_POINT('',(3.72235838409899,2.2344646706273,4.3));
#16982=CARTESIAN_POINT('Origin',(3.6,2.4,4.3));
#16983=CARTESIAN_POINT('Ctrl Pts',(3.394277315143,2.4001195557093,4.34540747194623));
#16984=CARTESIAN_POINT('Ctrl Pts',(3.39422704674216,2.40728359221916,4.34501772883951));
#16985=CARTESIAN_POINT('Ctrl Pts',(3.39781627947545,2.48249299124839,4.34092338938053));
#16986=CARTESIAN_POINT('Ctrl Pts',(3.49037003538787,2.61673301642169,4.33312445356927));
#16987=CARTESIAN_POINT('Ctrl Pts',(3.72265542052987,2.60960761604941,4.32201066451248));
#16988=CARTESIAN_POINT('Ctrl Pts',(3.84179830935629,2.41200908789601,4.31096917998937));
#16989=CARTESIAN_POINT('Ctrl Pts',(3.77594284069862,2.27417970060314,4.30363229181856));
#16990=CARTESIAN_POINT('Ctrl Pts',(3.72235851517117,2.23446447326397,4.3));
#16991=CARTESIAN_POINT('Origin',(3.6,2.4,5.35459252805377));
#16992=CARTESIAN_POINT('',(3.39480734911062,2.40010265425899,4.41540747194623));
#16993=CARTESIAN_POINT('',(3.39433274005607,2.39985021891194,4.40959252805377));
#16994=CARTESIAN_POINT('',(3.394525,2.40000000000001,5.35459252805377));
#16995=CARTESIAN_POINT('Ctrl Pts',(3.39433274005607,2.39985021891194,4.40959252805377));
#16996=CARTESIAN_POINT('Ctrl Pts',(3.39481384314024,2.45851949137253,4.40640305253959));
#16997=CARTESIAN_POINT('Ctrl Pts',(3.45186169840294,2.58615034863243,4.39950898067315));
#16998=CARTESIAN_POINT('Ctrl Pts',(3.66843098640644,2.63302756431036,4.38891031245443));
#16999=CARTESIAN_POINT('Ctrl Pts',(3.83289206978718,2.4688824684104,4.37779652339763));
#17000=CARTESIAN_POINT('Ctrl Pts',(3.78418106902943,2.24170425860662,4.36668273434082));
#17001=CARTESIAN_POINT('Ctrl Pts',(3.56689371899776,2.15938431325527,4.35556894528402));
#17002=CARTESIAN_POINT('Ctrl Pts',(3.41495577575702,2.27149583748734,4.34653887652167));
#17003=CARTESIAN_POINT('Ctrl Pts',(3.39474723286599,2.36992492448255,4.34121340411158));
#17004=CARTESIAN_POINT('Ctrl Pts',(3.39483887138702,2.39991986985508,4.33959252805377));
#17005=CARTESIAN_POINT('Ctrl Pts',(3.39480734911062,2.40010265425899,4.41540747194623));
#17006=CARTESIAN_POINT('Ctrl Pts',(3.3946821849205,2.42777437678442,4.41391197361979));
#17007=CARTESIAN_POINT('Ctrl Pts',(3.41278383405305,2.52383658927861,4.40871187894108));
#17008=CARTESIAN_POINT('Ctrl Pts',(3.55878722266986,2.63934344974957,4.3998071879101));
#17009=CARTESIAN_POINT('Ctrl Pts',(3.77873475080197,2.56443107632444,4.38869339885329));
#17010=CARTESIAN_POINT('Ctrl Pts',(3.8350828706128,2.33901445723046,4.37757960979649));
#17011=CARTESIAN_POINT('Ctrl Pts',(3.67625990394949,2.16941582752504,4.36646582073968));
#17012=CARTESIAN_POINT('Ctrl Pts',(3.45564722223464,2.20942500090864,4.3557417747896));
#17013=CARTESIAN_POINT('Ctrl Pts',(3.394704859258,2.33918780536763,4.34872232519178));
#17014=CARTESIAN_POINT('Ctrl Pts',(3.394277315143,2.4001195557093,4.34540747194623));
#17015=CARTESIAN_POINT('Origin',(3.6,2.4,5.35459252805377));
#17016=CARTESIAN_POINT('',(3.39465010046741,2.39982347235041,4.48540747194623));
#17017=CARTESIAN_POINT('',(3.39437120031462,2.40016339024638,4.47959252805377));
#17018=CARTESIAN_POINT('',(3.394525,2.40000000000001,5.35459252805377));
#17019=CARTESIAN_POINT('Ctrl Pts',(3.39437120031462,2.40016339024638,4.47959252805377));
#17020=CARTESIAN_POINT('Ctrl Pts',(3.39427672852213,2.41103322262123,4.47900189367213));
#17021=CARTESIAN_POINT('Ctrl Pts',(3.40000383140382,2.48998144241434,4.47470666293823));
#17022=CARTESIAN_POINT('Ctrl Pts',(3.5022614856576,2.62233051762717,4.46670683585207));
#17023=CARTESIAN_POINT('Ctrl Pts',(3.73378446379617,2.60269537158839,4.45559304679526));
#17024=CARTESIAN_POINT('Ctrl Pts',(3.84285303079348,2.39753073097072,4.44447925773845));
#17025=CARTESIAN_POINT('Ctrl Pts',(3.72963541291671,2.19462648510256,4.43336546868165));
#17026=CARTESIAN_POINT('Ctrl Pts',(3.49776113486282,2.17970245626759,4.42225167962485));
#17027=CARTESIAN_POINT('Ctrl Pts',(3.39915518291127,2.31283529949844,4.41432736608222));
#17028=CARTESIAN_POINT('Ctrl Pts',(3.39425503880932,2.39037475353659,4.41010764889186));
#17029=CARTESIAN_POINT('Ctrl Pts',(3.39433274005607,2.39985021891194,4.40959252805377));
#17030=CARTESIAN_POINT('Ctrl Pts',(3.39465010046741,2.39982347235041,4.48540747194623));
#17031=CARTESIAN_POINT('Ctrl Pts',(3.39504368040953,2.44786270507631,4.48280621840007));
#17032=CARTESIAN_POINT('Ctrl Pts',(3.43581223293462,2.56491921556266,4.47650036850162));
#17033=CARTESIAN_POINT('Ctrl Pts',(3.63081864137997,2.64090222813732,4.46648992225093));
#17034=CARTESIAN_POINT('Ctrl Pts',(3.81910984841827,2.50475947107891,4.45537613319412));
#17035=CARTESIAN_POINT('Ctrl Pts',(3.80684730359907,2.27272920356226,4.44426234413732));
#17036=CARTESIAN_POINT('Ctrl Pts',(3.60525512148808,2.15719129638054,4.43314855508051));
#17037=CARTESIAN_POINT('Ctrl Pts',(3.42662677463403,2.24954018398722,4.42353026435015));
#17038=CARTESIAN_POINT('Ctrl Pts',(3.39499223729164,2.35922694980568,4.41761656997206));
#17039=CARTESIAN_POINT('Ctrl Pts',(3.39480734911062,2.40010265425899,4.41540747194623));
#17040=CARTESIAN_POINT('Origin',(3.6,2.4,5.35459252805377));
#17041=CARTESIAN_POINT('',(3.39418405900746,2.40000082772182,4.55540747194623));
#17042=CARTESIAN_POINT('',(3.39484822543359,2.40004689761745,4.54959252805377));
#17043=CARTESIAN_POINT('',(3.394525,2.40000000000001,5.35459252805377));
#17044=CARTESIAN_POINT('Ctrl Pts',(3.39484822543359,2.40004689761745,4.54959252805377));
#17045=CARTESIAN_POINT('Ctrl Pts',(3.3947841161748,2.43145144364515,4.54789613845241));
#17046=CARTESIAN_POINT('Ctrl Pts',(3.41632347620735,2.53135423912678,4.54249515249878));
#17047=CARTESIAN_POINT('Ctrl Pts',(3.57178887938318,2.64122151037363,4.5333895701929));
#17048=CARTESIAN_POINT('Ctrl Pts',(3.78736363324621,2.55452687009752,4.52227578113608));
#17049=CARTESIAN_POINT('Ctrl Pts',(3.83144232915068,2.3263920312721,4.51116199207928));
#17050=CARTESIAN_POINT('Ctrl Pts',(3.66367923564831,2.1656314047897,4.50004820302247));
#17051=CARTESIAN_POINT('Ctrl Pts',(3.44964305208187,2.21653398832958,4.48952504834731));
#17052=CARTESIAN_POINT('Ctrl Pts',(3.39486927759939,2.34285510326715,4.4827064900244));
#17053=CARTESIAN_POINT('Ctrl Pts',(3.39437120031462,2.40016339024638,4.47959252805377));
#17054=CARTESIAN_POINT('Ctrl Pts',(3.39418406069018,2.40000082771773,4.55540747194623));
#17055=CARTESIAN_POINT('Ctrl Pts',(3.39418405804479,2.40004511873352,4.55540505953261));
#17056=CARTESIAN_POINT('Ctrl Pts',(3.39420412805525,2.46810441674863,4.55169805076671));
#17057=CARTESIAN_POINT('Ctrl Pts',(3.46841582920963,2.6041305389052,4.54428644564855));
#17058=CARTESIAN_POINT('Ctrl Pts',(3.70013763173937,2.6212603119689,4.53317265659175));
#17059=CARTESIAN_POINT('Ctrl Pts',(3.84020232447629,2.43586801205837,4.52205886753494));
#17060=CARTESIAN_POINT('Ctrl Pts',(3.76040710518764,2.21764531427324,4.51094507847815));
#17061=CARTESIAN_POINT('Ctrl Pts',(3.53378944408678,2.16633392770918,4.49983128942133));
#17062=CARTESIAN_POINT('Ctrl Pts',(3.40663178603677,2.29085017634376,4.4913187539107));
#17063=CARTESIAN_POINT('Ctrl Pts',(3.39448316034026,2.37944724185309,4.48651081475233));
#17064=CARTESIAN_POINT('Ctrl Pts',(3.39465010046741,2.39982347235041,4.48540747194623));
#17065=CARTESIAN_POINT('Origin',(3.6,2.4,5.35459252805377));
#17066=CARTESIAN_POINT('',(3.3946525152789,2.40017600729827,4.62540747194623));
#17067=CARTESIAN_POINT('',(3.39454318727431,2.3998121083938,4.61959252805377));
#17068=CARTESIAN_POINT('',(3.394525,2.40000000000001,5.35459252805377));
#17069=CARTESIAN_POINT('Ctrl Pts',(3.39454318727431,2.3998121083938,4.61959252805377));
#17070=CARTESIAN_POINT('Ctrl Pts',(3.39501368913604,2.45149296169584,4.61679038323269));
#17071=CARTESIAN_POINT('Ctrl Pts',(3.44097934710978,2.57224452612634,4.61028364205933));
#17072=CARTESIAN_POINT('Ctrl Pts',(3.64379902916374,2.63888350626668,4.60007230453372));
#17073=CARTESIAN_POINT('Ctrl Pts',(3.8244536406683,2.49275908427381,4.5889585154769));
#17074=CARTESIAN_POINT('Ctrl Pts',(3.79966328939795,2.26173122045618,4.57784472642011));
#17075=CARTESIAN_POINT('Ctrl Pts',(3.59211886499353,2.15726233868846,4.56673093736329));
#17076=CARTESIAN_POINT('Ctrl Pts',(3.42236627044389,2.25700668735564,4.55731353790786));
#17077=CARTESIAN_POINT('Ctrl Pts',(3.39492411875798,2.36286981206378,4.55160073480468));
#17078=CARTESIAN_POINT('Ctrl Pts',(3.39484822543359,2.40004689761745,4.54959252805377));
#17079=CARTESIAN_POINT('Ctrl Pts',(3.3946525152789,2.40017600729827,4.62540747194623));
#17080=CARTESIAN_POINT('Ctrl Pts',(3.3944854829676,2.42064195048213,4.62429930431288));
#17081=CARTESIAN_POINT('Ctrl Pts',(3.40670159662045,2.50933048007129,4.61948654032727));
#17082=CARTESIAN_POINT('Ctrl Pts',(3.53409308462842,2.63375189718637,4.61096917998938));
#17083=CARTESIAN_POINT('Ctrl Pts',(3.76064388996454,2.58214612691277,4.59985539093257));
#17084=CARTESIAN_POINT('Ctrl Pts',(3.84015552099323,2.36381994099575,4.58874160187577));
#17085=CARTESIAN_POINT('Ctrl Pts',(3.6998500801025,2.17860977340027,4.57762781281896));
#17086=CARTESIAN_POINT('Ctrl Pts',(3.46820102232696,2.19603680731826,4.56651643617579));
#17087=CARTESIAN_POINT('Ctrl Pts',(3.3941881204111,2.33203010926412,4.55910965588488));
#17088=CARTESIAN_POINT('Ctrl Pts',(3.39418406069018,2.40000082771773,4.55540747194623));
#17089=CARTESIAN_POINT('Origin',(3.6,2.4,5.35459252805377));
#17090=CARTESIAN_POINT('',(3.39480596940119,2.39989608913133,4.69540747194623));
#17091=CARTESIAN_POINT('',(3.394211384704,2.40006787741663,4.68959252805377));
#17092=CARTESIAN_POINT('',(3.394525,2.40000000000001,5.35459252805377));
#17093=CARTESIAN_POINT('Ctrl Pts',(3.394211384704,2.40006787741663,4.68959252805377));
#17094=CARTESIAN_POINT('Ctrl Pts',(3.39419531260529,2.40380178642024,4.68938922436523));
#17095=CARTESIAN_POINT('Ctrl Pts',(3.3959796032358,2.47555925126455,4.68548132432442));
#17096=CARTESIAN_POINT('Ctrl Pts',(3.47964553527297,2.61094664572852,4.67786882793135));
#17097=CARTESIAN_POINT('Ctrl Pts',(3.71195459435803,2.61552228034691,4.66675503887453));
#17098=CARTESIAN_POINT('Ctrl Pts',(3.84179034357568,2.42282792757511,4.65564124981774));
#17099=CARTESIAN_POINT('Ctrl Pts',(3.75031264922961,2.20923891380705,4.64452746076093));
#17100=CARTESIAN_POINT('Ctrl Pts',(3.5212520823821,2.17025568561017,4.63341367170412));
#17101=CARTESIAN_POINT('Ctrl Pts',(3.40385053057498,2.29836868031663,4.62510202746841));
#17102=CARTESIAN_POINT('Ctrl Pts',(3.39439165865867,2.38316790612259,4.62049497958496));
#17103=CARTESIAN_POINT('Ctrl Pts',(3.39454318727431,2.3998121083938,4.61959252805377));
#17104=CARTESIAN_POINT('Ctrl Pts',(3.39480596940119,2.39989608913133,4.69540747194623));
#17105=CARTESIAN_POINT('Ctrl Pts',(3.39499356749685,2.44086040282664,4.69319354909316));
#17106=CARTESIAN_POINT('Ctrl Pts',(3.42673277743261,2.55063876982526,4.68727502988781));
#17107=CARTESIAN_POINT('Ctrl Pts',(3.60557055501943,2.64280164712995,4.67765191433021));
#17108=CARTESIAN_POINT('Ctrl Pts',(3.80701249526159,2.52700195958257,4.6665381252734));
#17109=CARTESIAN_POINT('Ctrl Pts',(3.81897355090948,2.29495593812904,4.65542433621659));
#17110=CARTESIAN_POINT('Ctrl Pts',(3.63050563208088,2.15905793778677,4.6443105471598));
#17111=CARTESIAN_POINT('Ctrl Pts',(3.43569204443384,2.23525749529523,4.63430492573634));
#17112=CARTESIAN_POINT('Ctrl Pts',(3.39504387077152,2.35222445101461,4.62800390066515));
#17113=CARTESIAN_POINT('Ctrl Pts',(3.3946525152789,2.40017600729827,4.62540747194623));
#17114=CARTESIAN_POINT('Origin',(3.6,2.4,5.35459252805377));
#17115=CARTESIAN_POINT('',(3.39427329960995,2.39987978133526,4.76540747194623));
#17116=CARTESIAN_POINT('',(3.3947435825044,2.40014509868052,4.75959252805377));
#17117=CARTESIAN_POINT('',(3.394525,2.40000000000001,5.35459252805377));
#17118=CARTESIAN_POINT('Ctrl Pts',(3.3947435825044,2.40014509868052,4.75959252805377));
#17119=CARTESIAN_POINT('Ctrl Pts',(3.39458577035565,2.4243482239957,4.7582834691455));
#17120=CARTESIAN_POINT('Ctrl Pts',(3.40973683471182,2.51685424764646,4.75326981388497));
#17121=CARTESIAN_POINT('Ctrl Pts',(3.54682833602434,2.63697354002902,4.74455156227216));
#17122=CARTESIAN_POINT('Ctrl Pts',(3.77025746491439,2.57319376479756,4.73343777321537));
#17123=CARTESIAN_POINT('Ctrl Pts',(3.83784800531731,2.35088777249601,4.72232398415856));
#17124=CARTESIAN_POINT('Ctrl Pts',(3.68773356907346,2.1735347589994,4.71121019510175));
#17125=CARTESIAN_POINT('Ctrl Pts',(3.46153062024069,2.20292038334059,4.70029970973349));
#17126=CARTESIAN_POINT('Ctrl Pts',(3.3944881781145,2.3357625601094,4.6930938207175));
#17127=CARTESIAN_POINT('Ctrl Pts',(3.394211384704,2.40006787741663,4.68959252805377));
#17128=CARTESIAN_POINT('Ctrl Pts',(3.39427329960995,2.39987978133526,4.76540747194623));
#17129=CARTESIAN_POINT('Ctrl Pts',(3.39469744196064,2.4608980648022,4.76208779387343));
#17130=CARTESIAN_POINT('Ctrl Pts',(3.45579877538026,2.59074744458416,4.75506351944837));
#17131=CARTESIAN_POINT('Ctrl Pts',(3.67655778221991,2.63048335496042,4.74433464867103));
#17132=CARTESIAN_POINT('Ctrl Pts',(3.8351627244929,2.46068083668937,4.73322085961423));
#17133=CARTESIAN_POINT('Ctrl Pts',(3.77852055811084,2.23533646042905,4.72210707055742));
#17134=CARTESIAN_POINT('Ctrl Pts',(3.55847650032912,2.16071048934957,4.71099328150062));
#17135=CARTESIAN_POINT('Ctrl Pts',(3.41270208696854,2.27634402495147,4.70209341529689));
#17136=CARTESIAN_POINT('Ctrl Pts',(3.39467965627817,2.37231409061976,4.69689814544543));
#17137=CARTESIAN_POINT('Ctrl Pts',(3.39480596940119,2.39989608913133,4.69540747194623));
#17138=CARTESIAN_POINT('Origin',(3.6,2.4,5.35459252805377));
#17139=CARTESIAN_POINT('',(3.39444175184043,2.40017991402784,4.83540747194624));
#17140=CARTESIAN_POINT('',(3.39473574996246,2.39985120338455,4.82959252805377));
#17141=CARTESIAN_POINT('',(3.394525,2.40000000000001,5.35459252805377));
#17142=CARTESIAN_POINT('Ctrl Pts',(3.39473574996246,2.39985120338455,4.82959252805377));
#17143=CARTESIAN_POINT('Ctrl Pts',(3.39503501794323,2.44449429908603,4.82717771392578));
#17144=CARTESIAN_POINT('Ctrl Pts',(3.43129921147106,2.55806759504416,4.82105830344552));
#17145=CARTESIAN_POINT('Ctrl Pts',(3.61869057107309,2.64214530157901,4.811234296613));
#17146=CARTESIAN_POINT('Ctrl Pts',(3.81357662871545,2.51562312999728,4.80012050755618));
#17147=CARTESIAN_POINT('Ctrl Pts',(3.81297357597085,2.28326979627357,4.78900671849939));
#17148=CARTESIAN_POINT('Ctrl Pts',(3.61743339385551,2.1577609418312,4.77789292944258));
#17149=CARTESIAN_POINT('Ctrl Pts',(3.43084782690273,2.24264334099221,4.76808819929404));
#17150=CARTESIAN_POINT('Ctrl Pts',(3.39503237387128,2.35585412553307,4.76198806549777));
#17151=CARTESIAN_POINT('Ctrl Pts',(3.3947435825044,2.40014509868052,4.75959252805377));
#17152=CARTESIAN_POINT('Ctrl Pts',(3.39444175184043,2.40017991402784,4.83540747194624));
#17153=CARTESIAN_POINT('Ctrl Pts',(3.39432006446725,2.41345772041588,4.83468663500598));
#17154=CARTESIAN_POINT('Ctrl Pts',(3.40154214948563,2.49484232576125,4.83026120171345));
#17155=CARTESIAN_POINT('Ctrl Pts',(3.51011506296999,2.62561996593247,4.82213117206865));
#17156=CARTESIAN_POINT('Ctrl Pts',(3.74080745251389,2.59788110634618,4.81101738301186));
#17157=CARTESIAN_POINT('Ctrl Pts',(3.84261718390667,2.38901942599691,4.79990359395504));
#17158=CARTESIAN_POINT('Ctrl Pts',(3.72235665540369,2.19020838956081,4.78878980489825));
#17159=CARTESIAN_POINT('Ctrl Pts',(3.49010169259086,2.18342199335841,4.77767601584144));
#17160=CARTESIAN_POINT('Ctrl Pts',(3.3977657456792,2.31768599948744,4.76988190485744));
#17161=CARTESIAN_POINT('Ctrl Pts',(3.39422412009908,2.39280468183069,4.7657923902257));
#17162=CARTESIAN_POINT('Ctrl Pts',(3.39427329960995,2.39987978133526,4.76540747194623));
#17163=CARTESIAN_POINT('Origin',(3.6,2.4,5.35459252805377));
#17164=CARTESIAN_POINT('',(3.39485784124953,2.40000781019044,4.90540747194623));
#17165=CARTESIAN_POINT('',(3.39420665921585,2.39993826201568,4.89959252805377));
#17166=CARTESIAN_POINT('',(3.394525,2.40000000000001,5.35459252805377));
#17167=CARTESIAN_POINT('Ctrl Pts',(3.39420665921585,2.39993826201568,4.89959252805377));
#17168=CARTESIAN_POINT('Ctrl Pts',(3.39446259615796,2.46459365987715,4.89607195870605));
#17169=CARTESIAN_POINT('Ctrl Pts',(3.46215556435864,2.59774588363475,4.88884679300606));
#17170=CARTESIAN_POINT('Ctrl Pts',(3.68890792061744,2.62600678347214,4.87791703095382));
#17171=CARTESIAN_POINT('Ctrl Pts',(3.83809973223177,2.44787694680091,4.86680324189701));
#17172=CARTESIAN_POINT('Ctrl Pts',(3.76935615869971,2.22592479776177,4.85568945284022));
#17173=CARTESIAN_POINT('Ctrl Pts',(3.54559897248035,2.16330565547811,4.8445756637834));
#17174=CARTESIAN_POINT('Ctrl Pts',(3.40943456861369,2.28386778049975,4.83587668885459));
#17175=CARTESIAN_POINT('Ctrl Pts',(3.39457590721621,2.37600677138249,4.83088231027805));
#17176=CARTESIAN_POINT('Ctrl Pts',(3.39473574996246,2.39985120338455,4.82959252805377));
#17177=CARTESIAN_POINT('Ctrl Pts',(3.39485784124953,2.40000781019044,4.90540747194623));
#17178=CARTESIAN_POINT('Ctrl Pts',(3.39484637525965,2.43382668251502,4.90358087978625));
#17179=CARTESIAN_POINT('Ctrl Pts',(3.41876409372263,2.5362199118863,4.898049691274));
#17180=CARTESIAN_POINT('Ctrl Pts',(3.58026192098975,2.64206213906777,4.88881390640948));
#17181=CARTESIAN_POINT('Ctrl Pts',(3.79266519873933,2.54786410019675,4.87770011735268));
#17182=CARTESIAN_POINT('Ctrl Pts',(3.82871983510845,2.3183243735256,4.86658632829587));
#17183=CARTESIAN_POINT('Ctrl Pts',(3.65542461254465,2.16354327402962,4.85547253923907));
#17184=CARTESIAN_POINT('Ctrl Pts',(3.44592887095679,2.22119506991598,4.84507958712252));
#17185=CARTESIAN_POINT('Ctrl Pts',(3.39494545222641,2.34521910726469,4.83839123135825));
#17186=CARTESIAN_POINT('Ctrl Pts',(3.39444175184043,2.40017991402784,4.83540747194624));
#17187=CARTESIAN_POINT('Origin',(3.6,2.4,5.35459252805377));
#17188=CARTESIAN_POINT('',(3.39447042093573,2.39981603086916,4.97540747194623));
#17189=CARTESIAN_POINT('',(3.39455384621585,2.40018770306997,4.96959252805377));
#17190=CARTESIAN_POINT('',(3.394525,2.40000000000001,5.35459252805377));
#17191=CARTESIAN_POINT('Ctrl Pts',(3.39455384621585,2.40018770306997,4.96959252805377));
#17192=CARTESIAN_POINT('Ctrl Pts',(3.39439993536132,2.41718968163228,4.9686707998386));
#17193=CARTESIAN_POINT('Ctrl Pts',(3.40410689916048,2.50235241402357,4.96404447527116));
#17194=CARTESIAN_POINT('Ctrl Pts',(3.52244569778922,2.63014998309056,4.95571355435144));
#17195=CARTESIAN_POINT('Ctrl Pts',(3.7513008249214,2.58997827483123,4.94459976529465));
#17196=CARTESIAN_POINT('Ctrl Pts',(3.84166859114005,2.37591729705878,4.93348597623783));
#17197=CARTESIAN_POINT('Ctrl Pts',(3.71083435517744,2.18389949043478,4.92237218718104));
#17198=CARTESIAN_POINT('Ctrl Pts',(3.47855217697512,2.18968093094735,4.91125839812423));
#17199=CARTESIAN_POINT('Ctrl Pts',(3.39580021960588,2.32515686494945,4.90366517841514));
#17200=CARTESIAN_POINT('Ctrl Pts',(3.39419328089429,2.3965585986654,4.89977655505832));
#17201=CARTESIAN_POINT('Ctrl Pts',(3.39420665921585,2.39993826201568,4.89959252805377));
#17202=CARTESIAN_POINT('Ctrl Pts',(3.39447042093573,2.39981603086916,4.97540747194623));
#17203=CARTESIAN_POINT('Ctrl Pts',(3.39496908070531,2.45384921408654,4.97247512456653));
#17204=CARTESIAN_POINT('Ctrl Pts',(3.44450059321654,2.57695438413994,4.96583818083455));
#17205=CARTESIAN_POINT('Ctrl Pts',(3.652145851588,2.63720135146115,4.95549664075031));
#17206=CARTESIAN_POINT('Ctrl Pts',(3.82756721950384,2.48483414141864,4.9443828516935));
#17207=CARTESIAN_POINT('Ctrl Pts',(3.79469373046592,2.25481727983819,4.9332690626367));
#17208=CARTESIAN_POINT('Ctrl Pts',(3.58361486203243,2.15768780841241,4.9221552735799));
#17209=CARTESIAN_POINT('Ctrl Pts',(3.41976019074743,2.26186083674666,4.91286807668307));
#17210=CARTESIAN_POINT('Ctrl Pts',(3.39486962996599,2.36523705764074,4.90728547613852));
#17211=CARTESIAN_POINT('Ctrl Pts',(3.39485784124953,2.40000781019044,4.90540747194623));
#17212=CARTESIAN_POINT('Origin',(3.6,2.4,5.35459252805377));
#17213=CARTESIAN_POINT('',(3.3942529072965,2.40010656251954,5.04540747194623));
#17214=CARTESIAN_POINT('',(3.39484564919972,2.39994744459104,5.03959252805377));
#17215=CARTESIAN_POINT('',(3.394525,2.40000000000001,5.35459252805377));
#17216=CARTESIAN_POINT('Ctrl Pts',(3.39484564919972,2.39994744459104,5.03959252805377));
#17217=CARTESIAN_POINT('Ctrl Pts',(3.39493157223083,2.43748021568483,5.03756504461887));
#17218=CARTESIAN_POINT('Ctrl Pts',(3.42276238606253,2.54371108636155,5.03183296483171));
#17219=CARTESIAN_POINT('Ctrl Pts',(3.59337897158896,2.64277529828296,5.02239628869227));
#17220=CARTESIAN_POINT('Ctrl Pts',(3.80037832359127,2.53723050760561,5.01128249963547));
#17221=CARTESIAN_POINT('Ctrl Pts',(3.82396912389365,2.30607707315216,5.00016871057866));
#17222=CARTESIAN_POINT('Ctrl Pts',(3.64255844494981,2.16089236073089,4.98905492152186));
#17223=CARTESIAN_POINT('Ctrl Pts',(3.44046962361553,2.22845545212382,4.97886286068023));
#17224=CARTESIAN_POINT('Ctrl Pts',(3.39501853158186,2.34885558191993,4.97237539619086));
#17225=CARTESIAN_POINT('Ctrl Pts',(3.39455384621585,2.40018770306997,4.96959252805377));
#17226=CARTESIAN_POINT('Ctrl Pts',(3.3942529072965,2.40010656251954,5.04540747194623));
#17227=CARTESIAN_POINT('Ctrl Pts',(3.39421422426863,2.40623506914945,5.04507396569907));
#17228=CARTESIAN_POINT('Ctrl Pts',(3.39724233203131,2.4804004332851,5.04103586309963));
#17229=CARTESIAN_POINT('Ctrl Pts',(3.48711398178203,2.61503583311392,5.03329316414794));
#17230=CARTESIAN_POINT('Ctrl Pts',(3.71944062032543,2.61146538882495,5.02217937509113));
#17231=CARTESIAN_POINT('Ctrl Pts',(3.84244192441188,2.41433825182845,5.01106558603433));
#17232=CARTESIAN_POINT('Ctrl Pts',(3.74353337567863,2.20408716238119,4.99995179697753));
#17233=CARTESIAN_POINT('Ctrl Pts',(3.51324710536571,2.17315730898832,4.98883800792072));
#17234=CARTESIAN_POINT('Ctrl Pts',(3.40217617393534,2.30323677769677,4.98065656624362));
#17235=CARTESIAN_POINT('Ctrl Pts',(3.39433909628525,2.38558611032407,4.97617972091879));
#17236=CARTESIAN_POINT('Ctrl Pts',(3.39447042093573,2.39981603086916,4.97540747194623));
#17237=CARTESIAN_POINT('Origin',(3.6,2.4,5.35459252805377));
#17238=CARTESIAN_POINT('',(3.39479089114249,2.40011619889285,5.11540747194623));
#17239=CARTESIAN_POINT('',(3.39436118415265,2.39983962587988,5.10959252805377));
#17240=CARTESIAN_POINT('',(3.394525,2.40000000000001,5.35459252805377));
#17241=CARTESIAN_POINT('Ctrl Pts',(3.39436118415265,2.39983962587988,5.10959252805377));
#17242=CARTESIAN_POINT('Ctrl Pts',(3.39485594839208,2.45749534742618,5.10645928939915));
#17243=CARTESIAN_POINT('Ctrl Pts',(3.45020483086988,2.58415305598872,5.09962145439226));
#17244=CARTESIAN_POINT('Ctrl Pts',(3.66489494817768,2.63403475512075,5.08907902303309));
#17245=CARTESIAN_POINT('Ctrl Pts',(3.83182128848718,2.47240567698227,5.0779652339763));
#17246=CARTESIAN_POINT('Ctrl Pts',(3.78655899556261,2.24450261226871,5.06685144491949));
#17247=CARTESIAN_POINT('Ctrl Pts',(3.57053712771522,2.15892819449186,5.05573765586269));
#17248=CARTESIAN_POINT('Ctrl Pts',(3.41597203014558,2.26936665662614,5.04665135024078));
#17249=CARTESIAN_POINT('Ctrl Pts',(3.39477457457446,2.36890073212835,5.04126964097114));
#17250=CARTESIAN_POINT('Ctrl Pts',(3.39484564919972,2.39994744459104,5.03959252805377));
#17251=CARTESIAN_POINT('Ctrl Pts',(3.39479089114249,2.40011619889285,5.11540747194623));
#17252=CARTESIAN_POINT('Ctrl Pts',(3.39465311263348,2.42674223574529,5.11396821047934));
#17253=CARTESIAN_POINT('Ctrl Pts',(3.4118399484044,2.5217320012959,5.10882435266019));
#17254=CARTESIAN_POINT('Ctrl Pts',(3.55516852834243,2.63869087044012,5.09997589848876));
#17255=CARTESIAN_POINT('Ctrl Pts',(3.77622353148193,2.56711958879047,5.08886210943196));
#17256=CARTESIAN_POINT('Ctrl Pts',(3.8359804180852,2.34258029751366,5.07774832037515));
#17257=CARTESIAN_POINT('Ctrl Pts',(3.6797411123384,2.17059868763558,5.06663453131835));
#17258=CARTESIAN_POINT('Ctrl Pts',(3.45739289886954,2.2074502474941,5.05585424850871));
#17259=CARTESIAN_POINT('Ctrl Pts',(3.39464391638139,2.33815945287815,5.04877856205133));
#17260=CARTESIAN_POINT('Ctrl Pts',(3.3942529072965,2.40010656251954,5.04540747194623));
#17261=CARTESIAN_POINT('Origin',(3.6,2.4,5.35459252805377));
#17262=CARTESIAN_POINT('',(3.39473291096846,2.39977036782444,5.18540747194623));
#17263=CARTESIAN_POINT('',(3.39434265438876,2.4001499379742,5.17959252805377));
#17264=CARTESIAN_POINT('',(3.394525,2.40000000000001,5.35459252805377));
#17265=CARTESIAN_POINT('',(3.54698297828114,2.20148256743283,5.2));
#17266=CARTESIAN_POINT('Ctrl Pts',(3.54698297828114,2.20148256743283,5.2));
#17267=CARTESIAN_POINT('Ctrl Pts',(3.48097120902544,2.21911198848201,5.19629540364773));
#17268=CARTESIAN_POINT('Ctrl Pts',(3.40750559920538,2.28872805295596,5.19143122762981));
#17269=CARTESIAN_POINT('Ctrl Pts',(3.39457126112442,2.3783468402669,5.18656705161189));
#17270=CARTESIAN_POINT('Ctrl Pts',(3.39473291096846,2.39977036782444,5.18540747194623));
#17271=CARTESIAN_POINT('',(3.6531315533849,2.20112677566065,5.2));
#17272=CARTESIAN_POINT('Origin',(3.6,2.4,5.2));
#17273=CARTESIAN_POINT('Ctrl Pts',(3.65313162618093,2.20112654952031,5.2));
#17274=CARTESIAN_POINT('Ctrl Pts',(3.58867175365004,2.1839946978326,5.19636770818145));
#17275=CARTESIAN_POINT('Ctrl Pts',(3.45069166079049,2.21593288928867,5.1895652175327));
#17276=CARTESIAN_POINT('Ctrl Pts',(3.39482801182151,2.34184093155955,5.18276272688396));
#17277=CARTESIAN_POINT('Ctrl Pts',(3.39434265438876,2.4001499379742,5.17959252805377));
#17278=CARTESIAN_POINT('Origin',(-3.6,2.4,4.7));
#17279=CARTESIAN_POINT('',(-3.76675586981256,2.39987855699196,4.38714803633902));
#17280=CARTESIAN_POINT('',(-3.76680083090633,2.40009693666208,4.36785196366098));
#17281=CARTESIAN_POINT('',(-3.7666,2.4,4.7));
#17282=CARTESIAN_POINT('',(-3.76351293272515,2.3680769545372,4.3));
#17283=CARTESIAN_POINT('Ctrl Pts',(-3.76680083090633,2.40009693666208,4.36785196366098));
#17284=CARTESIAN_POINT('Ctrl Pts',(-3.76684158871352,2.40590556800081,4.36746222055426));
#17285=CARTESIAN_POINT('Ctrl Pts',(-3.76656456795221,2.41171030753034,4.36707247744754));
#17286=CARTESIAN_POINT('Ctrl Pts',(-3.76595693377405,2.41748025837345,4.36668273434082));
#17287=CARTESIAN_POINT('Ctrl Pts',(-3.76018123352143,2.47232494575256,4.36297813798855));
#17288=CARTESIAN_POINT('Ctrl Pts',(-3.72453483477909,2.52402649885475,4.35927354163629));
#17289=CARTESIAN_POINT('Ctrl Pts',(-3.67532197505843,2.54891439179576,4.35556894528402));
#17290=CARTESIAN_POINT('Ctrl Pts',(-3.62610911533777,2.57380228473677,4.35186434893175));
#17291=CARTESIAN_POINT('Ctrl Pts',(-3.56332979463879,2.5718765175166,4.34815975257948));
#17292=CARTESIAN_POINT('Ctrl Pts',(-3.51573443689162,2.5440364869014,4.34445515622722));
#17293=CARTESIAN_POINT('Ctrl Pts',(-3.46813907914445,2.5161964562862,4.34075055987495));
#17294=CARTESIAN_POINT('Ctrl Pts',(-3.43572768434908,2.46244216227597,4.33704596352268));
#17295=CARTESIAN_POINT('Ctrl Pts',(-3.43329507915076,2.40733835292718,4.33334136717041));
#17296=CARTESIAN_POINT('Ctrl Pts',(-3.43086247395245,2.35223454357839,4.32963677081815));
#17297=CARTESIAN_POINT('Ctrl Pts',(-3.45840865835118,2.29578121889103,4.32593217446588));
#17298=CARTESIAN_POINT('Ctrl Pts',(-3.50340586780517,2.26388777182752,4.32222757811361));
#17299=CARTESIAN_POINT('Ctrl Pts',(-3.54840307725917,2.23199432476401,4.31852298176134));
#17300=CARTESIAN_POINT('Ctrl Pts',(-3.61085131176843,2.22466075532434,4.31481838540907));
#17301=CARTESIAN_POINT('Ctrl Pts',(-3.66197498261058,2.24508842770105,4.3111137890568));
#17302=CARTESIAN_POINT('Ctrl Pts',(-3.71309865345273,2.26551610007776,4.30740919270453));
#17303=CARTESIAN_POINT('Ctrl Pts',(-3.75289776062778,2.31370501427083,4.30370459635227));
#17304=CARTESIAN_POINT('Ctrl Pts',(-3.76351293272515,2.3680769545372,4.3));
#17305=CARTESIAN_POINT('',(-3.60525668225574,2.5668198662348,4.3));
#17306=CARTESIAN_POINT('Origin',(-3.6,2.4,4.3));
#17307=CARTESIAN_POINT('',(-3.76634548976639,2.39993502697971,4.31714803633902));
#17308=CARTESIAN_POINT('Ctrl Pts',(-3.60525667864057,2.56682005840211,4.3));
#17309=CARTESIAN_POINT('Ctrl Pts',(-3.65930634748376,2.56504681426963,4.30363229181856));
#17310=CARTESIAN_POINT('Ctrl Pts',(-3.71251717627762,2.53457816039784,4.30726458363711));
#17311=CARTESIAN_POINT('Ctrl Pts',(-3.74128611123357,2.48878409483897,4.31089687545566));
#17312=CARTESIAN_POINT('Ctrl Pts',(-3.75778985504382,2.46251362194275,4.31298059575011));
#17313=CARTESIAN_POINT('Ctrl Pts',(-3.76624996614321,2.43119967804664,4.31506431604457));
#17314=CARTESIAN_POINT('Ctrl Pts',(-3.76634548976639,2.39993502697971,4.31714803633902));
#17315=CARTESIAN_POINT('',(-3.7666,2.4,4.2));
#17316=CARTESIAN_POINT('',(-3.7666,2.4,4.7));
#17317=CARTESIAN_POINT('Origin',(-3.6,2.4,4.2));
#17318=CARTESIAN_POINT('Ctrl Pts',(-3.76634548976639,2.39993502697971,4.31714803633902));
#17319=CARTESIAN_POINT('Ctrl Pts',(-3.7664197953026,2.37561500451544,4.31876891239683));
#17320=CARTESIAN_POINT('Ctrl Pts',(-3.76143276332865,2.35132480870382,4.32038978845465));
#17321=CARTESIAN_POINT('Ctrl Pts',(-3.75123332497294,2.32946153149726,4.32201066451247));
#17322=CARTESIAN_POINT('Ctrl Pts',(-3.72792197926853,2.27949187675561,4.32571526086474));
#17323=CARTESIAN_POINT('Ctrl Pts',(-3.67738233884271,2.24219983197054,4.329419857217));
#17324=CARTESIAN_POINT('Ctrl Pts',(-3.62274960712982,2.23467803877973,4.33312445356927));
#17325=CARTESIAN_POINT('Ctrl Pts',(-3.56811687541693,2.22715624558892,4.33682904992154));
#17326=CARTESIAN_POINT('Ctrl Pts',(-3.50939105241698,2.24940470399237,4.34053364627381));
#17327=CARTESIAN_POINT('Ctrl Pts',(-3.473445625673,2.29122843734541,4.34423824262608));
#17328=CARTESIAN_POINT('Ctrl Pts',(-3.43750019892903,2.33305217069845,4.34794283897834));
#17329=CARTESIAN_POINT('Ctrl Pts',(-3.42433516844104,2.39445117900107,4.35164743533061));
#17330=CARTESIAN_POINT('Ctrl Pts',(-3.43997694242044,2.44733227209049,4.35535203168288));
#17331=CARTESIAN_POINT('Ctrl Pts',(-3.45561871639985,2.50021336517992,4.35905662803515));
#17332=CARTESIAN_POINT('Ctrl Pts',(-3.50006729484665,2.54457654305613,4.36276122438742));
#17333=CARTESIAN_POINT('Ctrl Pts',(-3.55297985590111,2.56011554237715,4.36646582073968));
#17334=CARTESIAN_POINT('Ctrl Pts',(-3.60589241695558,2.57565454169817,4.37017041709195));
#17335=CARTESIAN_POINT('Ctrl Pts',(-3.6672689606177,2.562369362464,4.37387501344422));
#17336=CARTESIAN_POINT('Ctrl Pts',(-3.70902050221487,2.52634164219194,4.37757960979649));
#17337=CARTESIAN_POINT('Ctrl Pts',(-3.74496652897209,2.49532354447962,4.38076908531067));
#17338=CARTESIAN_POINT('Ctrl Pts',(-3.76636578927508,2.4474478468568,4.38395856082485));
#17339=CARTESIAN_POINT('Ctrl Pts',(-3.76675586981256,2.39987855699196,4.38714803633902));
#17340=CARTESIAN_POINT('Origin',(-3.6,2.4,4.7));
#17341=CARTESIAN_POINT('',(-3.76672468602162,2.4001324774977,4.45714803633902));
#17342=CARTESIAN_POINT('',(-3.7663710759754,2.40008323252274,4.43785196366098));
#17343=CARTESIAN_POINT('',(-3.7666,2.4,4.7));
#17344=CARTESIAN_POINT('Ctrl Pts',(-3.7663710759754,2.40008323252274,4.43785196366098));
#17345=CARTESIAN_POINT('Ctrl Pts',(-3.76647255964094,2.42251958309795,4.43635646533454));
#17346=CARTESIAN_POINT('Ctrl Pts',(-3.76225162287627,2.44491933914913,4.43486096700809));
#17347=CARTESIAN_POINT('Ctrl Pts',(-3.75352689637225,2.46540054190021,4.43336546868165));
#17348=CARTESIAN_POINT('Ctrl Pts',(-3.73191430783919,2.516135863806,4.42966087232938));
#17349=CARTESIAN_POINT('Ctrl Pts',(-3.6826649015976,2.55509827647583,4.42595627597711));
#17350=CARTESIAN_POINT('Ctrl Pts',(-3.62831779967194,2.56445627090432,4.42225167962485));
#17351=CARTESIAN_POINT('Ctrl Pts',(-3.57397069774627,2.57381426533281,4.41854708327258));
#17352=CARTESIAN_POINT('Ctrl Pts',(-3.51452590013653,2.55356784151996,4.41484248692031));
#17353=CARTESIAN_POINT('Ctrl Pts',(-3.47718895189484,2.51298317028118,4.41113789056804));
#17354=CARTESIAN_POINT('Ctrl Pts',(-3.43985200365314,2.4723984990424,4.40743329421577));
#17355=CARTESIAN_POINT('Ctrl Pts',(-3.42462290477948,2.41147558037768,4.40372869786351));
#17356=CARTESIAN_POINT('Ctrl Pts',(-3.43847074534366,2.35809557252044,4.40002410151124));
#17357=CARTESIAN_POINT('Ctrl Pts',(-3.45231858590785,2.30471556466319,4.39631950515897));
#17358=CARTESIAN_POINT('Ctrl Pts',(-3.49524336590988,2.25887846761341,4.3926149088067));
#17359=CARTESIAN_POINT('Ctrl Pts',(-3.54760150451765,2.24156301194163,4.38891031245443));
#17360=CARTESIAN_POINT('Ctrl Pts',(-3.59995964312543,2.22424755626985,4.38520571610216));
#17361=CARTESIAN_POINT('Ctrl Pts',(-3.66175114033895,2.23545374197608,4.3815011197499));
#17362=CARTESIAN_POINT('Ctrl Pts',(-3.70469438806425,2.2700507456572,4.37779652339763));
#17363=CARTESIAN_POINT('Ctrl Pts',(-3.74311977927038,2.30100796178371,4.37448167015208));
#17364=CARTESIAN_POINT('Ctrl Pts',(-3.76645417654063,2.35069321376496,4.37116681690653));
#17365=CARTESIAN_POINT('Ctrl Pts',(-3.76680083090633,2.40009693666208,4.36785196366098));
#17366=CARTESIAN_POINT('Ctrl Pts',(-3.76675586981256,2.39987855699196,4.38714803633902));
#17367=CARTESIAN_POINT('Ctrl Pts',(-3.76681887033176,2.39219581029783,4.38766315717711));
#17368=CARTESIAN_POINT('Ctrl Pts',(-3.76633386046459,2.38452105604489,4.3881782780152));
#17369=CARTESIAN_POINT('Ctrl Pts',(-3.76527361543791,2.37692660254772,4.38869339885329));
#17370=CARTESIAN_POINT('Ctrl Pts',(-3.75764864753156,2.32230954448549,4.39239799520556));
#17371=CARTESIAN_POINT('Ctrl Pts',(-3.72027217218665,2.27184568967097,4.39610259155783));
#17372=CARTESIAN_POINT('Ctrl Pts',(-3.67024982973388,2.2486305064859,4.3998071879101));
#17373=CARTESIAN_POINT('Ctrl Pts',(-3.62022748728111,2.22541532330082,4.40351178426237));
#17374=CARTESIAN_POINT('Ctrl Pts',(-3.55755927772049,2.22944881174518,4.40721638061463));
#17375=CARTESIAN_POINT('Ctrl Pts',(-3.51092562033288,2.25888482364762,4.4109209769669));
#17376=CARTESIAN_POINT('Ctrl Pts',(-3.46429196294527,2.28832083555005,4.41462557331917));
#17377=CARTESIAN_POINT('Ctrl Pts',(-3.43369285773067,2.34315937091056,4.41833016967144));
#17378=CARTESIAN_POINT('Ctrl Pts',(-3.43313217976425,2.39830336261017,4.42203476602371));
#17379=CARTESIAN_POINT('Ctrl Pts',(-3.43257150179783,2.45344735430978,4.42573936237597));
#17380=CARTESIAN_POINT('Ctrl Pts',(-3.46204925107959,2.5088968023485,4.42944395872824));
#17381=CARTESIAN_POINT('Ctrl Pts',(-3.5080747579799,2.53927490269551,4.43314855508051));
#17382=CARTESIAN_POINT('Ctrl Pts',(-3.55410026488021,2.56965300304252,4.43685315143278));
#17383=CARTESIAN_POINT('Ctrl Pts',(-3.61667352939907,2.57495975569782,4.44055774778505));
#17384=CARTESIAN_POINT('Ctrl Pts',(-3.66715754746926,2.55276652004746,4.44426234413731));
#17385=CARTESIAN_POINT('Ctrl Pts',(-3.71764156553946,2.53057328439709,4.44796694048958));
#17386=CARTESIAN_POINT('Ctrl Pts',(-3.756036337161,2.48088006044104,4.45167153684185));
#17387=CARTESIAN_POINT('Ctrl Pts',(-3.76477027476388,2.4264292215015,4.45537613319412));
#17388=CARTESIAN_POINT('Ctrl Pts',(-3.7661627513915,2.41774796866627,4.45596676757575));
#17389=CARTESIAN_POINT('Ctrl Pts',(-3.76680128414385,2.40894578279607,4.45655740195739));
#17390=CARTESIAN_POINT('Ctrl Pts',(-3.76672468602162,2.4001324774977,4.45714803633902));
#17391=CARTESIAN_POINT('Origin',(-3.6,2.4,4.7));
#17392=CARTESIAN_POINT('',(-3.76633791206845,2.40003802478337,4.52714803633902));
#17393=CARTESIAN_POINT('',(-3.76649857382306,2.39985687062932,4.50785196366098));
#17394=CARTESIAN_POINT('',(-3.7666,2.4,4.7));
#17395=CARTESIAN_POINT('Ctrl Pts',(-3.76649857382306,2.39985687062932,4.50785196366098));
#17396=CARTESIAN_POINT('Ctrl Pts',(-3.76617945752874,2.43880728528579,4.50525071011481));
#17397=CARTESIAN_POINT('Ctrl Pts',(-3.75254366540545,2.47795898788161,4.50264945656864));
#17398=CARTESIAN_POINT('Ctrl Pts',(-3.72758425733276,2.50756395676541,4.50004820302248));
#17399=CARTESIAN_POINT('Ctrl Pts',(-3.6920381137294,2.54972611350612,4.49634360667021));
#17400=CARTESIAN_POINT('Ctrl Pts',(-3.63352511396685,2.57252533344874,4.49263901031794));
#17401=CARTESIAN_POINT('Ctrl Pts',(-3.57882406188105,2.56552742213501,4.48893441396567));
#17402=CARTESIAN_POINT('Ctrl Pts',(-3.52412300979526,2.55852951082128,4.4852298176134));
#17403=CARTESIAN_POINT('Ctrl Pts',(-3.47323390538621,2.52173446825121,4.48152522126114));
#17404=CARTESIAN_POINT('Ctrl Pts',(-3.44944644044618,2.47198175864633,4.47782062490887));
#17405=CARTESIAN_POINT('Ctrl Pts',(-3.42565897550616,2.42222904904145,4.4741160285566));
#17406=CARTESIAN_POINT('Ctrl Pts',(-3.42897315003517,2.35951867240177,4.47041143220433));
#17407=CARTESIAN_POINT('Ctrl Pts',(-3.45787220405951,2.31255037948392,4.46670683585206));
#17408=CARTESIAN_POINT('Ctrl Pts',(-3.48677125808385,2.26558208656607,4.46300223949979));
#17409=CARTESIAN_POINT('Ctrl Pts',(-3.54125519160353,2.23435587737005,4.45929764314752));
#17410=CARTESIAN_POINT('Ctrl Pts',(-3.59638914193523,2.23316262102818,4.45559304679526));
#17411=CARTESIAN_POINT('Ctrl Pts',(-3.65152309226694,2.23196936468632,4.45188845044299));
#17412=CARTESIAN_POINT('Ctrl Pts',(-3.70730705941068,2.26080906119861,4.44818385409072));
#17413=CARTESIAN_POINT('Ctrl Pts',(-3.73821115757027,2.30648302502563,4.44447925773845));
#17414=CARTESIAN_POINT('Ctrl Pts',(-3.75663966522468,2.33371899184293,4.44227015971263));
#17415=CARTESIAN_POINT('Ctrl Pts',(-3.76622116784026,2.36694103711801,4.4400610616868));
#17416=CARTESIAN_POINT('Ctrl Pts',(-3.7663710759754,2.40008323252274,4.43785196366098));
#17417=CARTESIAN_POINT('Ctrl Pts',(-3.76672468602162,2.4001324774977,4.45714803633902));
#17418=CARTESIAN_POINT('Ctrl Pts',(-3.76632084288778,2.35366668006347,4.46026199830966));
#17419=CARTESIAN_POINT('Ctrl Pts',(-3.74603890809821,2.30689180212375,4.46337596028029));
#17420=CARTESIAN_POINT('Ctrl Pts',(-3.71156689963546,2.27590095059859,4.46648992225092));
#17421=CARTESIAN_POINT('Ctrl Pts',(-3.67055648331992,2.23903197255825,4.47019451860319));
#17422=CARTESIAN_POINT('Ctrl Pts',(-3.60946254710462,2.2245024704006,4.47389911495546));
#17423=CARTESIAN_POINT('Ctrl Pts',(-3.55624507667009,2.23896195008268,4.47760371130773));
#17424=CARTESIAN_POINT('Ctrl Pts',(-3.50302760623556,2.25342142976477,4.48130830766));
#17425=CARTESIAN_POINT('Ctrl Pts',(-3.45768660158179,2.29686989128659,4.48501290401227));
#17426=CARTESIAN_POINT('Ctrl Pts',(-3.4409726309165,2.34942290140806,4.48871750036453));
#17427=CARTESIAN_POINT('Ctrl Pts',(-3.4242586602512,2.40197591152952,4.4924220967168));
#17428=CARTESIAN_POINT('Ctrl Pts',(-3.43617172357437,2.46363347025063,4.49612669306907));
#17429=CARTESIAN_POINT('Ctrl Pts',(-3.47125973974121,2.50617764542895,4.49983128942133));
#17430=CARTESIAN_POINT('Ctrl Pts',(-3.50634775590806,2.54872182060726,4.5035358857736));
#17431=CARTESIAN_POINT('Ctrl Pts',(-3.56461072491859,2.57215261224279,4.50724048212587));
#17432=CARTESIAN_POINT('Ctrl Pts',(-3.61938426871317,2.56574678606726,4.51094507847814));
#17433=CARTESIAN_POINT('Ctrl Pts',(-3.67415781250775,2.55934095989172,4.51464967483041));
#17434=CARTESIAN_POINT('Ctrl Pts',(-3.72544193108638,2.52309851590513,4.51835427118267));
#17435=CARTESIAN_POINT('Ctrl Pts',(-3.7497661567401,2.47360601391412,4.52205886753494));
#17436=CARTESIAN_POINT('Ctrl Pts',(-3.7609045803459,2.45094266337894,4.5237552571363));
#17437=CARTESIAN_POINT('Ctrl Pts',(-3.76638989212213,2.42550096131782,4.52545164673766));
#17438=CARTESIAN_POINT('Ctrl Pts',(-3.76633791206845,2.40003802478337,4.52714803633902));
#17439=CARTESIAN_POINT('Origin',(-3.6,2.4,4.7));
#17440=CARTESIAN_POINT('',(-3.76658523827666,2.39984765670423,4.59714803633902));
#17441=CARTESIAN_POINT('',(-3.76687644222506,2.40000067112036,4.57785196366098));
#17442=CARTESIAN_POINT('',(-3.7666,2.4,4.7));
#17443=CARTESIAN_POINT('Ctrl Pts',(-3.76687644086079,2.40000067111705,4.57785196366098));
#17444=CARTESIAN_POINT('Ctrl Pts',(-3.76687973678962,2.45518344204594,4.57414495489509));
#17445=CARTESIAN_POINT('Ctrl Pts',(-3.73679497953693,2.51036312381259,4.57043794612919));
#17446=CARTESIAN_POINT('Ctrl Pts',(-3.69041339694851,2.54026106127768,4.5667309373633));
#17447=CARTESIAN_POINT('Ctrl Pts',(-3.64406199814677,2.57013954203352,4.56302634101103));
#17448=CARTESIAN_POINT('Ctrl Pts',(-3.58143498975323,2.57476917303812,4.55932174465876));
#17449=CARTESIAN_POINT('Ctrl Pts',(-3.53119397724287,2.55203117737673,4.55561714830649));
#17450=CARTESIAN_POINT('Ctrl Pts',(-3.4809529647325,2.52929318171533,4.55191255195423));
#17451=CARTESIAN_POINT('Ctrl Pts',(-3.44309794810529,2.47918755938795,4.54820795560196));
#17452=CARTESIAN_POINT('Ctrl Pts',(-3.43495349044459,2.42464543263837,4.54450335924969));
#17453=CARTESIAN_POINT('Ctrl Pts',(-3.42680903278389,2.37010330588879,4.54079876289742));
#17454=CARTESIAN_POINT('Ctrl Pts',(-3.44837513408969,2.31112467471701,4.53709416654516));
#17455=CARTESIAN_POINT('Ctrl Pts',(-3.48978194566841,2.27470144397531,4.53338957019289));
#17456=CARTESIAN_POINT('Ctrl Pts',(-3.53118875724712,2.23827821323361,4.52968497384062));
#17457=CARTESIAN_POINT('Ctrl Pts',(-3.59243627909875,2.22441038292198,4.52598037748835));
#17458=CARTESIAN_POINT('Ctrl Pts',(-3.64549423583691,2.23944464448895,4.52227578113608));
#17459=CARTESIAN_POINT('Ctrl Pts',(-3.69855219257508,2.25447890605592,4.51857118478381));
#17460=CARTESIAN_POINT('Ctrl Pts',(-3.74342058419978,2.29841525950148,4.51486658843154));
#17461=CARTESIAN_POINT('Ctrl Pts',(-3.75956513629004,2.35114598299368,4.51116199207928));
#17462=CARTESIAN_POINT('Ctrl Pts',(-3.76437348076611,2.36685081528665,4.51005864927318));
#17463=CARTESIAN_POINT('Ctrl Pts',(-3.76663392958958,2.3833357360905,4.50895530646708));
#17464=CARTESIAN_POINT('Ctrl Pts',(-3.76649857382306,2.39985687062932,4.50785196366098));
#17465=CARTESIAN_POINT('Ctrl Pts',(-3.76633791206845,2.40003802478337,4.52714803633902));
#17466=CARTESIAN_POINT('Ctrl Pts',(-3.76627637744537,2.36989468919261,4.52915624308993));
#17467=CARTESIAN_POINT('Ctrl Pts',(-3.758454818996,2.33972159536913,4.53116444984084));
#17468=CARTESIAN_POINT('Ctrl Pts',(-3.74306538301875,2.31409282238037,4.53317265659175));
#17469=CARTESIAN_POINT('Ctrl Pts',(-3.71467605091489,2.26681469283306,4.53687725294402));
#17470=CARTESIAN_POINT('Ctrl Pts',(-3.66053305397837,2.23500099373388,4.54058184929628));
#17471=CARTESIAN_POINT('Ctrl Pts',(-3.6054152417587,2.23321144482349,4.54428644564855));
#17472=CARTESIAN_POINT('Ctrl Pts',(-3.55029742953903,2.23142189591311,4.54799104200082));
#17473=CARTESIAN_POINT('Ctrl Pts',(-3.49420480203621,2.25965649719153,4.55169563835309));
#17474=CARTESIAN_POINT('Ctrl Pts',(-3.46280846829882,2.30499352330658,4.55540023470536));
#17475=CARTESIAN_POINT('Ctrl Pts',(-3.43141213456143,2.35033054942163,4.55910483105762));
#17476=CARTESIAN_POINT('Ctrl Pts',(-3.42471209458945,2.41277000037331,4.56280942740989));
#17477=CARTESIAN_POINT('Ctrl Pts',(-3.44577465966535,2.46373610736585,4.56651402376216));
#17478=CARTESIAN_POINT('Ctrl Pts',(-3.46683722474125,2.51470221435838,4.57021862011443));
#17479=CARTESIAN_POINT('Ctrl Pts',(-3.51566239486502,2.55419497739177,4.5739232164667));
#17480=CARTESIAN_POINT('Ctrl Pts',(-3.56990505407324,2.56414030953056,4.57762781281897));
#17481=CARTESIAN_POINT('Ctrl Pts',(-3.62414771328146,2.57408564166935,4.58133240917123));
#17482=CARTESIAN_POINT('Ctrl Pts',(-3.68380786157412,2.55448354291355,4.5850370055235));
#17483=CARTESIAN_POINT('Ctrl Pts',(-3.72158169378842,2.51430502490722,4.58874160187577));
#17484=CARTESIAN_POINT('Ctrl Pts',(-3.75015369954742,2.4839141225134,4.59154374669685));
#17485=CARTESIAN_POINT('Ctrl Pts',(-3.76620375341029,2.44175070750818,4.59434589151794));
#17486=CARTESIAN_POINT('Ctrl Pts',(-3.76658523827666,2.39984765670423,4.59714803633902));
#17487=CARTESIAN_POINT('Origin',(-3.6,2.4,4.7));
#17488=CARTESIAN_POINT('',(-3.76685426518066,2.40005503529171,4.66714803633902));
#17489=CARTESIAN_POINT('',(-3.76649661588353,2.40014270746765,4.64785196366098));
#17490=CARTESIAN_POINT('',(-3.7666,2.4,4.7));
#17491=CARTESIAN_POINT('Ctrl Pts',(-3.76649661588353,2.40014270746765,4.64785196366098));
#17492=CARTESIAN_POINT('Ctrl Pts',(-3.76663204639349,2.41673658143502,4.64674379602763));
#17493=CARTESIAN_POINT('Ctrl Pts',(-3.76435138934107,2.43329406659146,4.64563562839428));
#17494=CARTESIAN_POINT('Ctrl Pts',(-3.75950152904524,2.44906128711078,4.64452746076093));
#17495=CARTESIAN_POINT('Ctrl Pts',(-3.74328848128947,2.50177099082653,4.64082286440866));
#17496=CARTESIAN_POINT('Ctrl Pts',(-3.69836304459695,2.54564901270383,4.63711826805639));
#17497=CARTESIAN_POINT('Ctrl Pts',(-3.64528559981485,2.5606143272255,4.63341367170412));
#17498=CARTESIAN_POINT('Ctrl Pts',(-3.59220815503275,2.57557964174716,4.62970907535186));
#17499=CARTESIAN_POINT('Ctrl Pts',(-3.53097870216106,2.56163224891319,4.62600447899959));
#17500=CARTESIAN_POINT('Ctrl Pts',(-3.48961924750057,2.52515525214062,4.62229988264732));
#17501=CARTESIAN_POINT('Ctrl Pts',(-3.44825979284008,2.48867825536805,4.61859528629505));
#17502=CARTESIAN_POINT('Ctrl Pts',(-3.4267703363908,2.42967165465689,4.61489068994278));
#17503=CARTESIAN_POINT('Ctrl Pts',(-3.43498564975134,2.37514015541382,4.61118609359051));
#17504=CARTESIAN_POINT('Ctrl Pts',(-3.44320096311188,2.32060865617075,4.60748149723825));
#17505=CARTESIAN_POINT('Ctrl Pts',(-3.48112104628225,2.27055225839578,4.60377690088598));
#17506=CARTESIAN_POINT('Ctrl Pts',(-3.53139155817582,2.2478795563676,4.60007230453371));
#17507=CARTESIAN_POINT('Ctrl Pts',(-3.58166207006939,2.22520685433943,4.59636770818145));
#17508=CARTESIAN_POINT('Ctrl Pts',(-3.64428301068616,2.22991784805805,4.59266311182918));
#17509=CARTESIAN_POINT('Ctrl Pts',(-3.69059555147242,2.25985652453919,4.58895851547691));
#17510=CARTESIAN_POINT('Ctrl Pts',(-3.73687793377613,2.28977570511195,4.58525633153827));
#17511=CARTESIAN_POINT('Ctrl Pts',(-3.76687314922176,2.34488972287695,4.58155414759963));
#17512=CARTESIAN_POINT('Ctrl Pts',(-3.76687644086079,2.40000067111705,4.57785196366098));
#17513=CARTESIAN_POINT('Ctrl Pts',(-3.76658523827666,2.39984765670423,4.59714803633902));
#17514=CARTESIAN_POINT('Ctrl Pts',(-3.76670809830844,2.38635246827757,4.5980504878702));
#17515=CARTESIAN_POINT('Ctrl Pts',(-3.76520579898216,2.37288428508147,4.59895293940139));
#17516=CARTESIAN_POINT('Ctrl Pts',(-3.76197323034856,2.35984505467766,4.59985539093257));
#17517=CARTESIAN_POINT('Ctrl Pts',(-3.74870341855848,2.30631853971129,4.60355998728484));
#17518=CARTESIAN_POINT('Ctrl Pts',(-3.70627627884239,2.26002044703541,4.60726458363711));
#17519=CARTESIAN_POINT('Ctrl Pts',(-3.65410883226945,2.24213936129044,4.61096917998938));
#17520=CARTESIAN_POINT('Ctrl Pts',(-3.60194138569651,2.22425827554546,4.61467377634165));
#17521=CARTESIAN_POINT('Ctrl Pts',(-3.54003363226672,2.23479419673139,4.61837837269391));
#17522=CARTESIAN_POINT('Ctrl Pts',(-3.49671800637814,2.26892530077511,4.62208296904618));
#17523=CARTESIAN_POINT('Ctrl Pts',(-3.45340238048956,2.30305640481884,4.62578756539845));
#17524=CARTESIAN_POINT('Ctrl Pts',(-3.42867888214219,2.36078269172036,4.62949216175072));
#17525=CARTESIAN_POINT('Ctrl Pts',(-3.43386236054643,2.4156853989487,4.63319675810298));
#17526=CARTESIAN_POINT('Ctrl Pts',(-3.43904583895067,2.47058810617705,4.63690135445525));
#17527=CARTESIAN_POINT('Ctrl Pts',(-3.47413629410653,2.52266723373221,4.64060595080752));
#17528=CARTESIAN_POINT('Ctrl Pts',(-3.52307438023553,2.54808847357993,4.64431054715979));
#17529=CARTESIAN_POINT('Ctrl Pts',(-3.57201246636453,2.57350971342765,4.64801514351206));
#17530=CARTESIAN_POINT('Ctrl Pts',(-3.63479818346667,2.57227306556792,4.65171973986433));
#17531=CARTESIAN_POINT('Ctrl Pts',(-3.68269729209092,2.54494448890598,4.65542433621659));
#17532=CARTESIAN_POINT('Ctrl Pts',(-3.73059640071517,2.51761591224403,4.65912893256886));
#17533=CARTESIAN_POINT('Ctrl Pts',(-3.76360890086153,2.46419540677987,4.66283352892113));
#17534=CARTESIAN_POINT('Ctrl Pts',(-3.76662643464441,2.40913116975406,4.6665381252734));
#17535=CARTESIAN_POINT('Ctrl Pts',(-3.76679203318471,2.406109312194,4.66674142896194));
#17536=CARTESIAN_POINT('Ctrl Pts',(-3.76686729650514,2.4030825042416,4.66694473265048));
#17537=CARTESIAN_POINT('Ctrl Pts',(-3.76685426518066,2.40005503529171,4.66714803633902));
#17538=CARTESIAN_POINT('Origin',(-3.6,2.4,4.7));
#17539=CARTESIAN_POINT('',(-3.76642275699063,2.40011764661364,4.73714803633902));
#17540=CARTESIAN_POINT('',(-3.76637219462709,2.39991574862477,4.71785196366098));
#17541=CARTESIAN_POINT('',(-3.7666,2.4,4.7));
#17542=CARTESIAN_POINT('Ctrl Pts',(-3.76637219462709,2.39991574862477,4.71785196366098));
#17543=CARTESIAN_POINT('Ctrl Pts',(-3.76622008929152,2.43312978877493,4.7156380408079));
#17544=CARTESIAN_POINT('Ctrl Pts',(-3.75659374130514,2.46642503349729,4.71342411795483));
#17545=CARTESIAN_POINT('Ctrl Pts',(-3.73808953093009,2.49369647329664,4.71121019510175));
#17546=CARTESIAN_POINT('Ctrl Pts',(-3.70712610771876,2.53933025690454,4.70750559874949));
#17547=CARTESIAN_POINT('Ctrl Pts',(-3.65130473898255,2.56809743365675,4.70380100239722));
#17548=CARTESIAN_POINT('Ctrl Pts',(-3.59617239065227,2.56683254199167,4.70009640604495));
#17549=CARTESIAN_POINT('Ctrl Pts',(-3.541040042322,2.56556765032658,4.69639180969268));
#17550=CARTESIAN_POINT('Ctrl Pts',(-3.48659671439765,2.53427069024418,4.69268721334041));
#17551=CARTESIAN_POINT('Ctrl Pts',(-3.45775870461848,2.48726489299201,4.68898261698815));
#17552=CARTESIAN_POINT('Ctrl Pts',(-3.4289206948393,2.44025909573984,4.68527802063588));
#17553=CARTESIAN_POINT('Ctrl Pts',(-3.4256880032053,2.3775444613179,4.68157342428361));
#17554=CARTESIAN_POINT('Ctrl Pts',(-3.44954008937339,2.32782269778556,4.67786882793134));
#17555=CARTESIAN_POINT('Ctrl Pts',(-3.47339217554148,2.27810093425323,4.67416423157907));
#17556=CARTESIAN_POINT('Ctrl Pts',(-3.52432903951166,2.2413720416105,4.67045963522681));
#17557=CARTESIAN_POINT('Ctrl Pts',(-3.57903913665629,2.23444520584228,4.66675503887454));
#17558=CARTESIAN_POINT('Ctrl Pts',(-3.63374923380092,2.22751837007406,4.66305044252227));
#17559=CARTESIAN_POINT('Ctrl Pts',(-3.69223256411999,2.25039359118035,4.65934584617));
#17560=CARTESIAN_POINT('Ctrl Pts',(-3.72772389987002,2.29260189451059,4.65564124981773));
#17561=CARTESIAN_POINT('Ctrl Pts',(-3.75259860001318,2.32218429445987,4.65304482109882));
#17562=CARTESIAN_POINT('Ctrl Pts',(-3.766179303182,2.36126338124449,4.6504483923799));
#17563=CARTESIAN_POINT('Ctrl Pts',(-3.76649661588353,2.40014270746765,4.64785196366098));
#17564=CARTESIAN_POINT('Ctrl Pts',(-3.76685426518066,2.40005503529171,4.66714803633902));
#17565=CARTESIAN_POINT('Ctrl Pts',(-3.76662983993221,2.34791601656576,4.67064932900275));
#17566=CARTESIAN_POINT('Ctrl Pts',(-3.7402175145738,2.29558094816933,4.67415062166648));
#17567=CARTESIAN_POINT('Ctrl Pts',(-3.69804051189557,2.26495998737175,4.6776519143302));
#17568=CARTESIAN_POINT('Ctrl Pts',(-3.65341448794446,2.23256101060272,4.68135651068247));
#17569=CARTESIAN_POINT('Ctrl Pts',(-3.59113987262282,2.22447102565214,4.68506110703474));
#17570=CARTESIAN_POINT('Ctrl Pts',(-3.53971699675369,2.24439246000598,4.68876570338701));
#17571=CARTESIAN_POINT('Ctrl Pts',(-3.48829412088457,2.26431389435981,4.69247029973927));
#17572=CARTESIAN_POINT('Ctrl Pts',(-3.44772298446796,2.31224674801807,4.69617489609154));
#17573=CARTESIAN_POINT('Ctrl Pts',(-3.43657119813891,2.36625427870627,4.69987949244381));
#17574=CARTESIAN_POINT('Ctrl Pts',(-3.42541941180987,2.42026180939447,4.70358408879608));
#17575=CARTESIAN_POINT('Ctrl Pts',(-3.44368697556839,2.48034401711262,4.70728868514835));
#17576=CARTESIAN_POINT('Ctrl Pts',(-3.48301363527625,2.51900393880922,4.71099328150062));
#17577=CARTESIAN_POINT('Ctrl Pts',(-3.52234029498412,2.55766386050582,4.71469787785288));
#17578=CARTESIAN_POINT('Ctrl Pts',(-3.58272605064134,2.57490149618086,4.71840247420515));
#17579=CARTESIAN_POINT('Ctrl Pts',(-3.63653501876085,2.56282794412363,4.72210707055742));
#17580=CARTESIAN_POINT('Ctrl Pts',(-3.69034398688037,2.5507543920664,4.72581166690969));
#17581=CARTESIAN_POINT('Ctrl Pts',(-3.73757616746218,2.50936965227689,4.72951626326196));
#17582=CARTESIAN_POINT('Ctrl Pts',(-3.75661548523835,2.45761368558721,4.73322085961422));
#17583=CARTESIAN_POINT('Ctrl Pts',(-3.76334323265594,2.43932515890074,4.73452991852249));
#17584=CARTESIAN_POINT('Ctrl Pts',(-3.76655071173719,2.4197416412828,4.73583897743076));
#17585=CARTESIAN_POINT('Ctrl Pts',(-3.76642275699063,2.40011764661364,4.73714803633902));
#17586=CARTESIAN_POINT('Origin',(-3.6,2.4,4.7));
#17587=CARTESIAN_POINT('',(-3.76642910764821,2.39987935508533,4.80714803633902));
#17588=CARTESIAN_POINT('',(-3.76680408556428,2.39990252619421,4.78785196366098));
#17589=CARTESIAN_POINT('',(-3.7666,2.4,4.7));
#17590=CARTESIAN_POINT('Ctrl Pts',(-3.76680408556428,2.39990252619421,4.78785196366098));
#17591=CARTESIAN_POINT('Ctrl Pts',(-3.76646018913848,2.44937641051311,4.78453228558818));
#17592=CARTESIAN_POINT('Ctrl Pts',(-3.74304696564969,2.49913297683607,4.78121260751538));
#17593=CARTESIAN_POINT('Ctrl Pts',(-3.70452480260444,2.53008579208055,4.77789292944258));
#17594=CARTESIAN_POINT('Ctrl Pts',(-3.66153597610701,2.56462760123568,4.77418833309031));
#17595=CARTESIAN_POINT('Ctrl Pts',(-3.59973129998187,2.5757522439241,4.77048373673804));
#17596=CARTESIAN_POINT('Ctrl Pts',(-3.54739603471406,2.55836846433844,4.76677914038578));
#17597=CARTESIAN_POINT('Ctrl Pts',(-3.49506076944624,2.54098468475278,4.76307454403351));
#17598=CARTESIAN_POINT('Ctrl Pts',(-3.45219491503573,2.49509248289304,4.75936994768124));
#17599=CARTESIAN_POINT('Ctrl Pts',(-3.43841627281944,2.44169468516681,4.75566535132897));
#17600=CARTESIAN_POINT('Ctrl Pts',(-3.42463763060315,2.38829688744059,4.7519607549767));
#17601=CARTESIAN_POINT('Ctrl Pts',(-3.43994620058106,2.32739349384788,4.74825615862443));
#17602=CARTESIAN_POINT('Ctrl Pts',(-3.4773359288973,2.28685728781211,4.74455156227217));
#17603=CARTESIAN_POINT('Ctrl Pts',(-3.51472565721353,2.24632108177635,4.7408469659199));
#17604=CARTESIAN_POINT('Ctrl Pts',(-3.57419654386808,2.22615206329753,4.73714236956763));
#17605=CARTESIAN_POINT('Ctrl Pts',(-3.62853140036063,2.23558069804861,4.73343777321536));
#17606=CARTESIAN_POINT('Ctrl Pts',(-3.68286625685319,2.24500933279969,4.7297331768631));
#17607=CARTESIAN_POINT('Ctrl Pts',(-3.73206508318374,2.28403562078066,4.72602858051083));
#17608=CARTESIAN_POINT('Ctrl Pts',(-3.7536117575058,2.33479896000292,4.72232398415856));
#17609=CARTESIAN_POINT('Ctrl Pts',(-3.76228181312143,2.35522535934946,4.72083331065937));
#17610=CARTESIAN_POINT('Ctrl Pts',(-3.76647460984564,2.37755214666628,4.71934263716017));
#17611=CARTESIAN_POINT('Ctrl Pts',(-3.76637219462709,2.39991574862477,4.71785196366098));
#17612=CARTESIAN_POINT('Ctrl Pts',(-3.76642275699063,2.40011764661364,4.73714803633902));
#17613=CARTESIAN_POINT('Ctrl Pts',(-3.76618860374924,2.36420634137441,4.73954357378302));
#17614=CARTESIAN_POINT('Ctrl Pts',(-3.75478479252022,2.32815948710566,4.74193911122702));
#17615=CARTESIAN_POINT('Ctrl Pts',(-3.73334402193678,2.29966496724918,4.74433464867103));
#17616=CARTESIAN_POINT('Ctrl Pts',(-3.70018678588852,2.25559940919069,4.74803924502329));
#17617=CARTESIAN_POINT('Ctrl Pts',(-3.64302585882149,2.22959548666357,4.75174384137557));
#17618=CARTESIAN_POINT('Ctrl Pts',(-3.58802126313241,2.23355404226464,4.75544843772783));
#17619=CARTESIAN_POINT('Ctrl Pts',(-3.53301666744333,2.2375125978657,4.7591530340801));
#17620=CARTESIAN_POINT('Ctrl Pts',(-3.48016840313221,2.27143363159494,4.76285763043237));
#17621=CARTESIAN_POINT('Ctrl Pts',(-3.45366277803107,2.31979299002082,4.76656222678463));
#17622=CARTESIAN_POINT('Ctrl Pts',(-3.42715715292992,2.36815234844671,4.7702668231369));
#17623=CARTESIAN_POINT('Ctrl Pts',(-3.42699416703876,2.43095003156924,4.77397141948917));
#17624=CARTESIAN_POINT('Ctrl Pts',(-3.45324841177486,2.47944632362031,4.77767601584144));
#17625=CARTESIAN_POINT('Ctrl Pts',(-3.47950265651095,2.52794261567138,4.78138061219371));
#17626=CARTESIAN_POINT('Ctrl Pts',(-3.53217413187432,2.56213751665099,4.78508520854598));
#17627=CARTESIAN_POINT('Ctrl Pts',(-3.58715743849732,2.56638153622754,4.78878980489824));
#17628=CARTESIAN_POINT('Ctrl Pts',(-3.64214074512033,2.57062555580409,4.79249440125051));
#17629=CARTESIAN_POINT('Ctrl Pts',(-3.69943588300298,2.54491869397758,4.79619899760278));
#17630=CARTESIAN_POINT('Ctrl Pts',(-3.73282140740775,2.50102584183074,4.79990359395505));
#17631=CARTESIAN_POINT('Ctrl Pts',(-3.754583518131,2.4724146061108,4.80231840808304));
#17632=CARTESIAN_POINT('Ctrl Pts',(-3.76618645992471,2.43607616275589,4.80473322221103));
#17633=CARTESIAN_POINT('Ctrl Pts',(-3.76642910764821,2.39987935508533,4.80714803633902));
#17634=CARTESIAN_POINT('Origin',(-3.6,2.4,4.7));
#17635=CARTESIAN_POINT('',(-3.76685809662611,2.39994994258553,4.87714803633902));
#17636=CARTESIAN_POINT('',(-3.7666675037778,2.40014587506062,4.85785196366098));
#17637=CARTESIAN_POINT('',(-3.7666,2.4,4.7));
#17638=CARTESIAN_POINT('Ctrl Pts',(-3.7666675037778,2.40014587506062,4.85785196366098));
#17639=CARTESIAN_POINT('Ctrl Pts',(-3.76676616841865,2.41091157707528,4.85713112672072));
#17640=CARTESIAN_POINT('Ctrl Pts',(-3.76581236284584,2.4216598706667,4.85641028978047));
#17641=CARTESIAN_POINT('Ctrl Pts',(-3.76374257225157,2.43218878210118,4.85568945284021));
#17642=CARTESIAN_POINT('Ctrl Pts',(-3.7531053001346,2.48630000298229,4.85198485648794));
#17643=CARTESIAN_POINT('Ctrl Pts',(-3.71299219510172,2.53461681652064,4.84828026013567));
#17644=CARTESIAN_POINT('Ctrl Pts',(-3.66176124712798,2.5550267590254,4.8445756637834));
#17645=CARTESIAN_POINT('Ctrl Pts',(-3.61053029915424,2.57543670153016,4.84087106743113));
#17646=CARTESIAN_POINT('Ctrl Pts',(-3.54818150823965,2.56793977300133,4.83716647107887));
#17647=CARTESIAN_POINT('Ctrl Pts',(-3.50324915208796,2.53596698529063,4.8334618747266));
#17648=CARTESIAN_POINT('Ctrl Pts',(-3.45831679593627,2.50399419757992,4.82975727837433));
#17649=CARTESIAN_POINT('Ctrl Pts',(-3.43080087454749,2.44754555068734,4.82605268202206));
#17650=CARTESIAN_POINT('Ctrl Pts',(-3.43329420537107,2.39245508794886,4.8223480856698));
#17651=CARTESIAN_POINT('Ctrl Pts',(-3.43578753619466,2.33736462521039,4.81864348931753));
#17652=CARTESIAN_POINT('Ctrl Pts',(-3.46829011923061,2.28363234662601,4.81493889296526));
#17653=CARTESIAN_POINT('Ctrl Pts',(-3.51592696305034,2.25584913417262,4.81123429661299));
#17654=CARTESIAN_POINT('Ctrl Pts',(-3.56356380687008,2.22806592171924,4.80752970026072));
#17655=CARTESIAN_POINT('Ctrl Pts',(-3.62633491147359,2.22623177539684,4.80382510390846));
#17656=CARTESIAN_POINT('Ctrl Pts',(-3.67551272490272,2.25118610267019,4.80012050755619));
#17657=CARTESIAN_POINT('Ctrl Pts',(-3.72469053833185,2.27614042994354,4.79641591120392));
#17658=CARTESIAN_POINT('Ctrl Pts',(-3.76027506058658,2.32788323081264,4.79271131485165));
#17659=CARTESIAN_POINT('Ctrl Pts',(-3.76598083327909,2.38273411905811,4.78900671849938));
#17660=CARTESIAN_POINT('Ctrl Pts',(-3.76657367957029,2.38843328504628,4.78862180021992));
#17661=CARTESIAN_POINT('Ctrl Pts',(-3.76684396052131,2.39416600535905,4.78823688194045));
#17662=CARTESIAN_POINT('Ctrl Pts',(-3.76680408556428,2.39990252619421,4.78785196366098));
#17663=CARTESIAN_POINT('Ctrl Pts',(-3.76642910764821,2.39987935508533,4.80714803633902));
#17664=CARTESIAN_POINT('Ctrl Pts',(-3.76655870881167,2.38054619044631,4.8084378185633));
#17665=CARTESIAN_POINT('Ctrl Pts',(-3.76344748981416,2.36125343108011,4.80972760078758));
#17666=CARTESIAN_POINT('Ctrl Pts',(-3.75691243582065,2.3432000486953,4.81101738301185));
#17667=CARTESIAN_POINT('Ctrl Pts',(-3.73814202890189,2.29134595017387,4.81472197936412));
#17668=CARTESIAN_POINT('Ctrl Pts',(-3.6911253041375,2.24971659559817,4.81842657571639));
#17669=CARTESIAN_POINT('Ctrl Pts',(-3.63737973221885,2.2373638951443,4.82213117206866));
#17670=CARTESIAN_POINT('Ctrl Pts',(-3.58363416030021,2.22501119469043,4.82583576842093));
#17671=CARTESIAN_POINT('Ctrl Pts',(-3.52315974122731,2.24193514835838,4.82954036477319));
#17672=CARTESIAN_POINT('Ctrl Pts',(-3.48363293580215,2.28039041278662,4.83324496112546));
#17673=CARTESIAN_POINT('Ctrl Pts',(-3.44410613037699,2.31884567721486,4.83694955747773));
#17674=CARTESIAN_POINT('Ctrl Pts',(-3.42552693859956,2.3788322524034,4.84065415383));
#17675=CARTESIAN_POINT('Ctrl Pts',(-3.436398232938,2.43289694207027,4.84435875018227));
#17676=CARTESIAN_POINT('Ctrl Pts',(-3.44726952727644,2.48696163173715,4.84806334653453));
#17677=CARTESIAN_POINT('Ctrl Pts',(-3.48759130773074,2.53510443588236,4.8517679428868));
#17678=CARTESIAN_POINT('Ctrl Pts',(-3.53891008283594,2.5552925272004,4.85547253923907));
#17679=CARTESIAN_POINT('Ctrl Pts',(-3.59022885794113,2.57548061851844,4.85917713559134));
#17680=CARTESIAN_POINT('Ctrl Pts',(-3.65254462769722,2.56771399700931,4.86288173194361));
#17681=CARTESIAN_POINT('Ctrl Pts',(-3.6973382267209,2.53554710104677,4.86658632829587));
#17682=CARTESIAN_POINT('Ctrl Pts',(-3.73990668943618,2.50497810589362,4.87010689764359));
#17683=CARTESIAN_POINT('Ctrl Pts',(-3.76665058188897,2.4523728080809,4.8736274669913));
#17684=CARTESIAN_POINT('Ctrl Pts',(-3.76685809662611,2.39994994258553,4.87714803633902));
#17685=CARTESIAN_POINT('Origin',(-3.6,2.4,4.7));
#17686=CARTESIAN_POINT('',(-3.76657659596252,2.40015219042981,4.94714803633902));
#17687=CARTESIAN_POINT('',(-3.76633013671136,2.4000063325357,4.92785196366098));
#17688=CARTESIAN_POINT('',(-3.7666,2.4,4.7));
#17689=CARTESIAN_POINT('Ctrl Pts',(-3.76633013671136,2.4000063325357,4.92785196366098));
#17690=CARTESIAN_POINT('Ctrl Pts',(-3.76633943338483,2.42742681836579,4.926025371501));
#17691=CARTESIAN_POINT('Ctrl Pts',(-3.75993532163491,2.454843216144,4.92419877934102));
#17692=CARTESIAN_POINT('Ctrl Pts',(-3.74709395519472,2.478810633836,4.92237218718103));
#17693=CARTESIAN_POINT('Ctrl Pts',(-3.72104978380566,2.52742006625356,4.91866759082877));
#17694=CARTESIAN_POINT('Ctrl Pts',(-3.66852675119931,2.56184254018683,4.9149629944765));
#17695=CARTESIAN_POINT('Ctrl Pts',(-3.61356232107187,2.56632441524918,4.91125839812423));
#17696=CARTESIAN_POINT('Ctrl Pts',(-3.55859789094443,2.57080629031153,4.90755380177196));
#17697=CARTESIAN_POINT('Ctrl Pts',(-3.5011920632959,2.54534756650297,4.90384920541969));
#17698=CARTESIAN_POINT('Ctrl Pts',(-3.46761694066379,2.50159957313644,4.90014460906742));
#17699=CARTESIAN_POINT('Ctrl Pts',(-3.43404181803167,2.45785157976992,4.89644001271516));
#17700=CARTESIAN_POINT('Ctrl Pts',(-3.42429740041597,2.39581431684543,4.89273541636289));
#17701=CARTESIAN_POINT('Ctrl Pts',(-3.44284327579263,2.34387948951498,4.88903082001062));
#17702=CARTESIAN_POINT('Ctrl Pts',(-3.46138915116929,2.29194466218454,4.88532622365835));
#17703=CARTESIAN_POINT('Ctrl Pts',(-3.50822531953831,2.25011227044814,4.88162162730609));
#17704=CARTESIAN_POINT('Ctrl Pts',(-3.56191694286671,2.23752714559004,4.87791703095382));
#17705=CARTESIAN_POINT('Ctrl Pts',(-3.61560856619511,2.22494202073194,4.87421243460155));
#17706=CARTESIAN_POINT('Ctrl Pts',(-3.6761556444829,2.24160416275214,4.87050783824928));
#17707=CARTESIAN_POINT('Ctrl Pts',(-3.71584846402625,2.27988804787417,4.86680324189701));
#17708=CARTESIAN_POINT('Ctrl Pts',(-3.7478178913646,2.31072268995097,4.863819482485));
#17709=CARTESIAN_POINT('Ctrl Pts',(-3.76625910135787,2.35558341867251,4.86083572307299));
#17710=CARTESIAN_POINT('Ctrl Pts',(-3.7666675037778,2.40014587506062,4.85785196366098));
#17711=CARTESIAN_POINT('Ctrl Pts',(-3.76685809662611,2.39994994258553,4.87714803633902));
#17712=CARTESIAN_POINT('Ctrl Pts',(-3.76686894382487,2.39720969748472,4.87733206334357));
#17713=CARTESIAN_POINT('Ctrl Pts',(-3.76680728418873,2.39446995085397,4.87751609034812));
#17714=CARTESIAN_POINT('Ctrl Pts',(-3.76667158779769,2.39173387609673,4.87770011735268));
#17715=CARTESIAN_POINT('Ctrl Pts',(-3.76393992155949,2.33665471752516,4.88140471370494));
#17716=CARTESIAN_POINT('Ctrl Pts',(-3.73120516079181,2.28306357079796,4.88510931005722));
#17717=CARTESIAN_POINT('Ctrl Pts',(-3.68344855437882,2.25548672809881,4.88881390640948));
#17718=CARTESIAN_POINT('Ctrl Pts',(-3.63569194796583,2.22790988539967,4.89251850276175));
#17719=CARTESIAN_POINT('Ctrl Pts',(-3.57291349590753,2.22634734672859,4.89622309911402));
#17720=CARTESIAN_POINT('Ctrl Pts',(-3.52384411276617,2.25151421676554,4.89992769546629));
#17721=CARTESIAN_POINT('Ctrl Pts',(-3.47477472962482,2.27668108680249,4.90363229181855));
#17722=CARTESIAN_POINT('Ctrl Pts',(-3.43941441540042,2.32857736554749,4.90733688817082));
#17723=CARTESIAN_POINT('Ctrl Pts',(-3.43394601840489,2.38345242676704,4.91104148452309));
#17724=CARTESIAN_POINT('Ctrl Pts',(-3.42847762140937,2.4383274879866,4.91474608087536));
#17725=CARTESIAN_POINT('Ctrl Pts',(-3.45290114164273,2.49618133168073,4.91845067722763));
#17726=CARTESIAN_POINT('Ctrl Pts',(-3.49603901657836,2.530536818217,4.9221552735799));
#17727=CARTESIAN_POINT('Ctrl Pts',(-3.539176891514,2.56489230475327,4.92585986993216));
#17728=CARTESIAN_POINT('Ctrl Pts',(-3.60102912115191,2.5757494341317,4.92956446628443));
#17729=CARTESIAN_POINT('Ctrl Pts',(-3.65328868187437,2.55813937955255,4.9332690626367));
#17730=CARTESIAN_POINT('Ctrl Pts',(-3.70554824259683,2.54052932497339,4.93697365898897));
#17731=CARTESIAN_POINT('Ctrl Pts',(-3.74821513440384,2.49445208643666,4.94067825534123));
#17732=CARTESIAN_POINT('Ctrl Pts',(-3.76176261231807,2.4409951733855,4.9443828516935));
#17733=CARTESIAN_POINT('Ctrl Pts',(-3.76513331494005,2.42769473782655,4.94530457990868));
#17734=CARTESIAN_POINT('Ctrl Pts',(-3.7667013875235,2.41393746536136,4.94622630812385));
#17735=CARTESIAN_POINT('Ctrl Pts',(-3.76657659596252,2.40015219042981,4.94714803633902));
#17736=CARTESIAN_POINT('Origin',(-3.6,2.4,4.7));
#17737=CARTESIAN_POINT('',(-3.76634000089015,2.39995738785102,5.01714803633902));
#17738=CARTESIAN_POINT('',(-3.76664425875303,2.39985083704439,4.99785196366098));
#17739=CARTESIAN_POINT('',(-3.7666,2.4,4.7));
#17740=CARTESIAN_POINT('Ctrl Pts',(-3.76664425875303,2.39985083704439,4.99785196366098));
#17741=CARTESIAN_POINT('Ctrl Pts',(-3.76623994328637,2.44366117230771,4.99491961628127));
#17742=CARTESIAN_POINT('Ctrl Pts',(-3.74849621432459,2.48776127465667,4.99198726890157));
#17743=CARTESIAN_POINT('Ctrl Pts',(-3.71750016303509,2.5184966637895,4.98905492152186));
#17744=CARTESIAN_POINT('Ctrl Pts',(-3.67834114001603,2.55732637791376,4.98535032516959));
#17745=CARTESIAN_POINT('Ctrl Pts',(-3.61803053064114,2.57482512236184,4.98164572881732));
#17746=CARTESIAN_POINT('Ctrl Pts',(-3.56416982715023,2.56298449736068,4.97794113246505));
#17747=CARTESIAN_POINT('Ctrl Pts',(-3.51030912365932,2.55114387235952,4.97423653611279));
#17748=CARTESIAN_POINT('Ctrl Pts',(-3.46289832605237,2.50996387790913,4.97053193976052));
#17749=CARTESIAN_POINT('Ctrl Pts',(-3.44363525475417,2.45829077205198,4.96682734340825));
#17750=CARTESIAN_POINT('Ctrl Pts',(-3.42437218345597,2.40661766619482,4.96312274705598));
#17751=CARTESIAN_POINT('Ctrl Pts',(-3.4332568384665,2.34445144893089,4.95941815070372));
#17752=CARTESIAN_POINT('Ctrl Pts',(-3.4662231070096,2.30024284205961,4.95571355435145));
#17753=CARTESIAN_POINT('Ctrl Pts',(-3.4991893755527,2.25603423518832,4.95200895799918));
#17754=CARTESIAN_POINT('Ctrl Pts',(-3.55623725762836,2.22978323870968,4.94830436164691));
#17755=CARTESIAN_POINT('Ctrl Pts',(-3.61125846653673,2.23350377003431,4.94459976529464));
#17756=CARTESIAN_POINT('Ctrl Pts',(-3.66627967544511,2.23722430135893,4.94089516894237));
#17757=CARTESIAN_POINT('Ctrl Pts',(-3.71927421118621,2.27091636048683,4.9371905725901));
#17758=CARTESIAN_POINT('Ctrl Pts',(-3.74598882397087,2.31916058550171,4.93348597623784));
#17759=CARTESIAN_POINT('Ctrl Pts',(-3.75953150177818,2.3436174623693,4.93160797204555));
#17760=CARTESIAN_POINT('Ctrl Pts',(-3.76632057836981,2.37181405816179,4.92972996785327));
#17761=CARTESIAN_POINT('Ctrl Pts',(-3.76633013671136,2.4000063325357,4.92785196366098));
#17762=CARTESIAN_POINT('Ctrl Pts',(-3.76657659596252,2.40015219042981,4.94714803633902));
#17763=CARTESIAN_POINT('Ctrl Pts',(-3.76619982713509,2.35853189310505,4.94993090447612));
#17764=CARTESIAN_POINT('Ctrl Pts',(-3.7503917908276,2.31665633988757,4.95271377261321));
#17765=CARTESIAN_POINT('Ctrl Pts',(-3.72217338919013,2.28632762005297,4.95549664075031));
#17766=CARTESIAN_POINT('Ctrl Pts',(-3.68460862412651,2.24595356733716,4.95920123710258));
#17767=CARTESIAN_POINT('Ctrl Pts',(-3.62505102997782,2.22604204947114,4.96290583345484));
#17768=CARTESIAN_POINT('Ctrl Pts',(-3.57075747740423,2.23570568531624,4.96661042980711));
#17769=CARTESIAN_POINT('Ctrl Pts',(-3.51646392483064,2.24536932116134,4.97031502615938));
#17770=CARTESIAN_POINT('Ctrl Pts',(-3.46743441383215,2.28460811071757,4.97401962251165));
#17771=CARTESIAN_POINT('Ctrl Pts',(-3.44610757816651,2.33546419983794,4.97772421886392));
#17772=CARTESIAN_POINT('Ctrl Pts',(-3.42478074250087,2.38632028895831,4.98142881521618));
#17773=CARTESIAN_POINT('Ctrl Pts',(-3.43115658216808,2.44879367764282,4.98513341156845));
#17774=CARTESIAN_POINT('Ctrl Pts',(-3.46231715792478,2.49429306452592,4.98883800792072));
#17775=CARTESIAN_POINT('Ctrl Pts',(-3.49347773368148,2.53979245140902,4.99254260427299));
#17776=CARTESIAN_POINT('Ctrl Pts',(-3.54942304552767,2.56831783649071,4.99624720062526));
#17777=CARTESIAN_POINT('Ctrl Pts',(-3.60454940439799,2.56681441711196,4.99995179697753));
#17778=CARTESIAN_POINT('Ctrl Pts',(-3.6596757632683,2.5653109977332,5.00365639332979));
#17779=CARTESIAN_POINT('Ctrl Pts',(-3.71398316916273,2.533778773894,5.00736098968206));
#17780=CARTESIAN_POINT('Ctrl Pts',(-3.7426175295644,2.48664864348361,5.01106558603433));
#17781=CARTESIAN_POINT('Ctrl Pts',(-3.75828878922747,2.46085485932866,5.01309306946923));
#17782=CARTESIAN_POINT('Ctrl Pts',(-3.76627033413891,2.43038911475947,5.01512055290412));
#17783=CARTESIAN_POINT('Ctrl Pts',(-3.76634000089015,2.39995738785102,5.01714803633902));
#17784=CARTESIAN_POINT('Origin',(-3.6,2.4,4.7));
#17785=CARTESIAN_POINT('',(-3.76673280722786,2.39986996770474,5.08714803633902));
#17786=CARTESIAN_POINT('',(-3.76682061973634,2.40008640134019,5.06785196366098));
#17787=CARTESIAN_POINT('',(-3.7666,2.4,4.7));
#17788=CARTESIAN_POINT('Ctrl Pts',(-3.76682061973634,2.40008640134019,5.06785196366098));
#17789=CARTESIAN_POINT('Ctrl Pts',(-3.76685198409984,2.40505542063702,5.06751845741382));
#17790=CARTESIAN_POINT('Ctrl Pts',(-3.76664920930319,2.41002184448446,5.06718495116665));
#17791=CARTESIAN_POINT('Ctrl Pts',(-3.76620395659798,2.41496643342036,5.06685144491949));
#17792=CARTESIAN_POINT('Ctrl Pts',(-3.76125807758801,2.46989106014367,5.06314684856722));
#17793=CARTESIAN_POINT('Ctrl Pts',(-3.7263932711654,2.5221215151067,5.05944225221495));
#17794=CARTESIAN_POINT('Ctrl Pts',(-3.67756562981921,2.54775425401002,5.05573765586269));
#17795=CARTESIAN_POINT('Ctrl Pts',(-3.62873798847301,2.57338699291335,5.05203305951042));
#17796=CARTESIAN_POINT('Ctrl Pts',(-3.56594751220322,2.57242201575698,5.04832846315815));
#17797=CARTESIAN_POINT('Ctrl Pts',(-3.51793061046379,2.54530094002895,5.04462386680588));
#17798=CARTESIAN_POINT('Ctrl Pts',(-3.46991370872435,2.51817986430092,5.04091927045361));
#17799=CARTESIAN_POINT('Ctrl Pts',(-3.43667038151527,2.46490269000124,5.03721467410135));
#17800=CARTESIAN_POINT('Ctrl Pts',(-3.4334146300602,2.40985202293434,5.03351007774908));
#17801=CARTESIAN_POINT('Ctrl Pts',(-3.43015887860513,2.35480135586744,5.02980548139681));
#17802=CARTESIAN_POINT('Ctrl Pts',(-3.45689070290407,2.29797719603331,5.02610088504454));
#17803=CARTESIAN_POINT('Ctrl Pts',(-3.50137612997721,2.26538543995573,5.02239628869227));
#17804=CARTESIAN_POINT('Ctrl Pts',(-3.54586155705034,2.23279368387816,5.01869169234));
#17805=CARTESIAN_POINT('Ctrl Pts',(-3.60810058689768,2.22443433155712,5.01498709598773));
#17806=CARTESIAN_POINT('Ctrl Pts',(-3.65960917559394,2.24413308920132,5.01128249963547));
#17807=CARTESIAN_POINT('Ctrl Pts',(-3.7111177642902,2.26383184684551,5.0075779032832));
#17808=CARTESIAN_POINT('Ctrl Pts',(-3.75189591183539,2.31158871445493,5.00387330693093));
#17809=CARTESIAN_POINT('Ctrl Pts',(-3.76328126727638,2.36554749015986,5.00016871057866));
#17810=CARTESIAN_POINT('Ctrl Pts',(-3.76565462410273,2.37679557365843,4.9993964616061));
#17811=CARTESIAN_POINT('Ctrl Pts',(-3.76675073733939,2.38831315681292,4.99862421263354));
#17812=CARTESIAN_POINT('Ctrl Pts',(-3.76664425875303,2.39985083704439,4.99785196366098));
#17813=CARTESIAN_POINT('Ctrl Pts',(-3.76634000089015,2.39995738785102,5.01714803633902));
#17814=CARTESIAN_POINT('Ctrl Pts',(-3.76639762849214,2.37478458425737,5.01882514925639));
#17815=CARTESIAN_POINT('Ctrl Pts',(-3.76104161363815,2.34963505698934,5.02050226217376));
#17816=CARTESIAN_POINT('Ctrl Pts',(-3.75014621226255,2.32717238066401,5.02217937509113));
#17817=CARTESIAN_POINT('Ctrl Pts',(-3.72607921965016,2.27755428523638,5.0258839714434));
#17818=CARTESIAN_POINT('Ctrl Pts',(-3.67498391951647,2.2410461313627,5.02958856779567));
#17819=CARTESIAN_POINT('Ctrl Pts',(-3.62024436463387,2.23435607004762,5.03329316414794));
#17820=CARTESIAN_POINT('Ctrl Pts',(-3.56550480975127,2.22766600873255,5.03699776050021));
#17821=CARTESIAN_POINT('Ctrl Pts',(-3.50712100011975,2.25079403997609,5.04070235685247));
#17822=CARTESIAN_POINT('Ctrl Pts',(-3.47181261940603,2.29315551442515,5.04440695320474));
#17823=CARTESIAN_POINT('Ctrl Pts',(-3.43650423869231,2.33551698887421,5.04811154955701));
#17824=CARTESIAN_POINT('Ctrl Pts',(-3.42427128689639,2.39711190652879,5.05181614590928));
#17825=CARTESIAN_POINT('Ctrl Pts',(-3.44071223950815,2.44975095341954,5.05552074226154));
#17826=CARTESIAN_POINT('Ctrl Pts',(-3.45715319211991,2.50239000031029,5.05922533861381));
#17827=CARTESIAN_POINT('Ctrl Pts',(-3.50226804913935,2.54607317643722,5.06292993496608));
#17828=CARTESIAN_POINT('Ctrl Pts',(-3.55540974897266,2.56080872993518,5.06663453131835));
#17829=CARTESIAN_POINT('Ctrl Pts',(-3.60855144880598,2.57554428343315,5.07033912767062));
#17830=CARTESIAN_POINT('Ctrl Pts',(-3.66971999145316,2.56133221430215,5.07404372402289));
#17831=CARTESIAN_POINT('Ctrl Pts',(-3.71092122942369,2.52467655355957,5.07774832037516));
#17832=CARTESIAN_POINT('Ctrl Pts',(-3.74576802490479,2.49367427362722,5.08088155902978));
#17833=CARTESIAN_POINT('Ctrl Pts',(-3.76633165033452,2.44661746651941,5.0840147976844));
#17834=CARTESIAN_POINT('Ctrl Pts',(-3.76673280722786,2.39986996770474,5.08714803633902));
#17835=CARTESIAN_POINT('Origin',(-3.6,2.4,4.7));
#17836=CARTESIAN_POINT('',(-3.76674783252531,2.40012156540224,5.15714803633902));
#17837=CARTESIAN_POINT('',(-3.76638442018051,2.4000942147675,5.13785196366098));
#17838=CARTESIAN_POINT('',(-3.7666,2.4,4.7));
#17839=CARTESIAN_POINT('',(-3.47309291201476,2.50793586530485,5.2));
#17840=CARTESIAN_POINT('Ctrl Pts',(-3.76674783252531,2.40012156540224,5.15714803633902));
#17841=CARTESIAN_POINT('Ctrl Pts',(-3.76635429688688,2.35284438834095,5.16031823516921));
#17842=CARTESIAN_POINT('Ctrl Pts',(-3.74524547308137,2.30526839815283,5.1634884339994));
#17843=CARTESIAN_POINT('Ctrl Pts',(-3.70967617106781,2.27424023606977,5.16665863282959));
#17844=CARTESIAN_POINT('Ctrl Pts',(-3.66811098429235,2.23798168503636,5.17036322918186));
#17845=CARTESIAN_POINT('Ctrl Pts',(-3.60679923783928,2.22432008207827,5.17406782553412));
#17846=CARTESIAN_POINT('Ctrl Pts',(-3.55380863333633,2.23961508023379,5.17777242188639));
#17847=CARTESIAN_POINT('Ctrl Pts',(-3.50081802883339,2.2549100783893,5.18147701823866));
#17848=CARTESIAN_POINT('Ctrl Pts',(-3.45614856628056,2.29916167765842,5.18518161459093));
#17849=CARTESIAN_POINT('Ctrl Pts',(-3.44024447629705,2.35186821788708,5.1888862109432));
#17850=CARTESIAN_POINT('Ctrl Pts',(-3.42434038631354,2.40457475811575,5.19259080729547));
#17851=CARTESIAN_POINT('Ctrl Pts',(-3.43720166889934,2.46573623930395,5.19629540364773));
#17852=CARTESIAN_POINT('Ctrl Pts',(-3.47309291201476,2.50793586530485,5.2));
#17853=CARTESIAN_POINT('',(-3.72714753727462,2.50812032359617,5.2));
#17854=CARTESIAN_POINT('Origin',(-3.6,2.4,5.2));
#17855=CARTESIAN_POINT('Ctrl Pts',(-3.72714768981588,2.50812044061668,5.2));
#17856=CARTESIAN_POINT('Ctrl Pts',(-3.69206189497277,2.54927257104909,5.19636770818145));
#17857=CARTESIAN_POINT('Ctrl Pts',(-3.63506413165932,2.57187758396405,5.19273541636289));
#17858=CARTESIAN_POINT('Ctrl Pts',(-3.58132375091077,2.56581791151438,5.18910312454434));
#17859=CARTESIAN_POINT('Ctrl Pts',(-3.52651361217864,2.55963761500343,5.18539852819207));
#17860=CARTESIAN_POINT('Ctrl Pts',(-3.475091829903,2.5236400741886,5.1816939318398));
#17861=CARTESIAN_POINT('Ctrl Pts',(-3.45055836676857,2.47425895866487,5.17798933548753));
#17862=CARTESIAN_POINT('Ctrl Pts',(-3.42602490363414,2.42487784314114,5.17428473913526));
#17863=CARTESIAN_POINT('Ctrl Pts',(-3.42837975964092,2.3621131529085,5.17058014278299));
#17864=CARTESIAN_POINT('Ctrl Pts',(-3.4565619363393,2.31470980183002,5.16687554643073));
#17865=CARTESIAN_POINT('Ctrl Pts',(-3.48474411303769,2.26730645075154,5.16317095007846));
#17866=CARTESIAN_POINT('Ctrl Pts',(-3.53875361042767,2.23526443882722,5.15946635372619));
#17867=CARTESIAN_POINT('Ctrl Pts',(-3.59386432951576,2.23323784347702,5.15576175737392));
#17868=CARTESIAN_POINT('Ctrl Pts',(-3.64897504860385,2.23121124812682,5.15205716102166));
#17869=CARTESIAN_POINT('Ctrl Pts',(-3.70518698939006,2.25920006935074,5.14835256466939));
#17870=CARTESIAN_POINT('Ctrl Pts',(-3.73677860664843,2.30440012364175,5.14464796831712));
#17871=CARTESIAN_POINT('Ctrl Pts',(-3.75609666072391,2.3320396422478,5.14238263343174));
#17872=CARTESIAN_POINT('Ctrl Pts',(-3.76620859139621,2.36611484945711,5.14011729854636));
#17873=CARTESIAN_POINT('Ctrl Pts',(-3.76638442018051,2.4000942147675,5.13785196366098));
#17874=CARTESIAN_POINT('Origin',(-3.6,2.4,5.35459252805377));
#17875=CARTESIAN_POINT('',(-3.80572269346025,2.40011955618633,4.34540747194623));
#17876=CARTESIAN_POINT('',(-3.8051611014991,2.39991986595833,4.33959252805377));
#17877=CARTESIAN_POINT('',(-3.805475,2.40000000000001,5.35459252805377));
#17878=CARTESIAN_POINT('',(-3.41173724903364,2.31767678198965,4.3));
#17879=CARTESIAN_POINT('Ctrl Pts',(-3.8051611014991,2.39991986595833,4.33959252805377));
#17880=CARTESIAN_POINT('Ctrl Pts',(-3.80504328807488,2.43847991504582,4.33750880775932));
#17881=CARTESIAN_POINT('Ctrl Pts',(-3.77605831390311,2.54576383181508,4.33172049111259));
#17882=CARTESIAN_POINT('Ctrl Pts',(-3.60297477126067,2.64299057240655,4.32222757811361));
#17883=CARTESIAN_POINT('Ctrl Pts',(-3.39749753058122,2.53388381093044,4.3111137890568));
#17884=CARTESIAN_POINT('Ctrl Pts',(-3.38436282049399,2.380278625644,4.30370459635227));
#17885=CARTESIAN_POINT('Ctrl Pts',(-3.41173724903364,2.31767678198965,4.3));
#17886=CARTESIAN_POINT('',(-3.47764162137361,2.23446466486417,4.3));
#17887=CARTESIAN_POINT('Origin',(-3.6,2.4,4.3));
#17888=CARTESIAN_POINT('Ctrl Pts',(-3.80572269346025,2.40011955618633,4.34540747194623));
#17889=CARTESIAN_POINT('Ctrl Pts',(-3.80577296183019,2.40728359294699,4.34501772883951));
#17890=CARTESIAN_POINT('Ctrl Pts',(-3.80218372831243,2.48249299452007,4.34092338938053));
#17891=CARTESIAN_POINT('Ctrl Pts',(-3.70962996035205,2.61673302206395,4.33312445356927));
#17892=CARTESIAN_POINT('Ctrl Pts',(-3.47734458963256,2.60960762555316,4.32201066451247));
#17893=CARTESIAN_POINT('Ctrl Pts',(-3.35820165688085,2.41200908723629,4.31096917998938));
#17894=CARTESIAN_POINT('Ctrl Pts',(-3.42405717417692,2.27417969332383,4.30363229181855));
#17895=CARTESIAN_POINT('Ctrl Pts',(-3.477641490197,2.23446446733471,4.3));
#17896=CARTESIAN_POINT('Origin',(-3.6,2.4,5.35459252805377));
#17897=CARTESIAN_POINT('',(-3.8051926580795,2.40010265427736,4.41540747194623));
#17898=CARTESIAN_POINT('',(-3.80566724099481,2.39985021907517,4.40959252805377));
#17899=CARTESIAN_POINT('',(-3.805475,2.40000000000001,5.35459252805377));
#17900=CARTESIAN_POINT('Ctrl Pts',(-3.80566724099481,2.39985021907517,4.40959252805377));
#17901=CARTESIAN_POINT('Ctrl Pts',(-3.80518613776288,2.45851948579172,4.40640305253959));
#17902=CARTESIAN_POINT('Ctrl Pts',(-3.74813828696622,2.58615032985374,4.39950898067314));
#17903=CARTESIAN_POINT('Ctrl Pts',(-3.53156902199863,2.63302754596983,4.38891031245443));
#17904=CARTESIAN_POINT('Ctrl Pts',(-3.36710794775451,2.46888245639993,4.37779652339763));
#17905=CARTESIAN_POINT('Ctrl Pts',(-3.41581895566904,2.24170428297288,4.36668273434082));
#17906=CARTESIAN_POINT('Ctrl Pts',(-3.63310626324856,2.15938431915927,4.35556894528402));
#17907=CARTESIAN_POINT('Ctrl Pts',(-3.78504422722635,2.27149586782626,4.34653887652167));
#17908=CARTESIAN_POINT('Ctrl Pts',(-3.80525274573711,2.36992492828818,4.34121340411158));
#17909=CARTESIAN_POINT('Ctrl Pts',(-3.8051611014991,2.39991986595833,4.33959252805377));
#17910=CARTESIAN_POINT('Ctrl Pts',(-3.8051926580795,2.40010265427736,4.41540747194623));
#17911=CARTESIAN_POINT('Ctrl Pts',(-3.80531782228225,2.42777437777342,4.41391197361979));
#17912=CARTESIAN_POINT('Ctrl Pts',(-3.78721617252902,2.52383659362796,4.40871187894108));
#17913=CARTESIAN_POINT('Ctrl Pts',(-3.64121277856108,2.63934345799643,4.3998071879101));
#17914=CARTESIAN_POINT('Ctrl Pts',(-3.4212652433475,2.56443108225311,4.38869339885329));
#17915=CARTESIAN_POINT('Ctrl Pts',(-3.36491712045917,2.33901445477475,4.3775796097965));
#17916=CARTESIAN_POINT('Ctrl Pts',(-3.52374009472539,2.16941582002738,4.36646582073968));
#17917=CARTESIAN_POINT('Ctrl Pts',(-3.7443527804805,2.20942499341216,4.3557417747896));
#17918=CARTESIAN_POINT('Ctrl Pts',(-3.80529514960796,2.33918780371163,4.34872232519178));
#17919=CARTESIAN_POINT('Ctrl Pts',(-3.80572269346025,2.40011955618633,4.34540747194623));
#17920=CARTESIAN_POINT('Origin',(-3.6,2.4,5.35459252805377));
#17921=CARTESIAN_POINT('',(-3.80534990670044,2.39982347234431,4.48540747194623));
#17922=CARTESIAN_POINT('',(-3.80562878067403,2.40016339023914,4.47959252805377));
#17923=CARTESIAN_POINT('',(-3.805475,2.40000000000001,5.35459252805377));
#17924=CARTESIAN_POINT('Ctrl Pts',(-3.80562878067403,2.40016339023914,4.47959252805377));
#17925=CARTESIAN_POINT('Ctrl Pts',(-3.80572325245773,2.41103322160878,4.47900189367213));
#17926=CARTESIAN_POINT('Ctrl Pts',(-3.79999615010417,2.4899814340984,4.47470666293823));
#17927=CARTESIAN_POINT('Ctrl Pts',(-3.69773850528383,2.62233049702197,4.46670683585206));
#17928=CARTESIAN_POINT('Ctrl Pts',(-3.46621554861493,2.60269535293104,4.45559304679526));
#17929=CARTESIAN_POINT('Ctrl Pts',(-3.35714699158608,2.39753073103871,4.44447925773845));
#17930=CARTESIAN_POINT('Ctrl Pts',(-3.47036459922058,2.19462650439043,4.43336546868165));
#17931=CARTESIAN_POINT('Ctrl Pts',(-3.70223885539349,2.17970247609322,4.42225167962484));
#17932=CARTESIAN_POINT('Ctrl Pts',(-3.80084479883202,2.31283530811152,4.41432736608222));
#17933=CARTESIAN_POINT('Ctrl Pts',(-3.80574494226542,2.39037475462753,4.41010764889186));
#17934=CARTESIAN_POINT('Ctrl Pts',(-3.80566724099481,2.39985021907517,4.40959252805377));
#17935=CARTESIAN_POINT('Ctrl Pts',(-3.80534990670044,2.39982347234431,4.48540747194623));
#17936=CARTESIAN_POINT('Ctrl Pts',(-3.804956326745,2.4478627067473,4.48280621840006));
#17937=CARTESIAN_POINT('Ctrl Pts',(-3.76418777279803,2.56491922132028,4.47650036850163));
#17938=CARTESIAN_POINT('Ctrl Pts',(-3.56918135753979,2.64090223654315,4.46648992225092));
#17939=CARTESIAN_POINT('Ctrl Pts',(-3.38089014394226,2.50475947474088,4.45537613319412));
#17940=CARTESIAN_POINT('Ctrl Pts',(-3.3931526891646,2.27272919910994,4.44426234413731));
#17941=CARTESIAN_POINT('Ctrl Pts',(-3.59474487835949,2.15719128792351,4.43314855508051));
#17942=CARTESIAN_POINT('Ctrl Pts',(-3.77337323137102,2.2495401787091,4.42353026435015));
#17943=CARTESIAN_POINT('Ctrl Pts',(-3.80500776987982,2.35922694839029,4.41761656997206));
#17944=CARTESIAN_POINT('Ctrl Pts',(-3.8051926580795,2.40010265427736,4.41540747194623));
#17945=CARTESIAN_POINT('Origin',(-3.6,2.4,5.35459252805377));
#17946=CARTESIAN_POINT('',(-3.80581594817644,2.40000082772184,4.55540747194624));
#17947=CARTESIAN_POINT('',(-3.80515175559583,2.40004689761323,4.54959252805377));
#17948=CARTESIAN_POINT('',(-3.805475,2.40000000000001,5.35459252805377));
#17949=CARTESIAN_POINT('Ctrl Pts',(-3.80515175559583,2.40004689761323,4.54959252805377));
#17950=CARTESIAN_POINT('Ctrl Pts',(-3.80521586484871,2.43145144073697,4.54789613845241));
#17951=CARTESIAN_POINT('Ctrl Pts',(-3.78367650680796,2.53135422698056,4.54249515249878));
#17952=CARTESIAN_POINT('Ctrl Pts',(-3.62821111800771,2.64122148806661,4.53338957019289));
#17953=CARTESIAN_POINT('Ctrl Pts',(-3.41263638408026,2.55452685581013,4.52227578113608));
#17954=CARTESIAN_POINT('Ctrl Pts',(-3.36855769224962,2.32639203807509,4.51116199207928));
#17955=CARTESIAN_POINT('Ctrl Pts',(-3.536320770243,2.1656314264689,4.50004820302247));
#17956=CARTESIAN_POINT('Ctrl Pts',(-3.75035693400944,2.21653400528296,4.48952504834731));
#17957=CARTESIAN_POINT('Ctrl Pts',(-3.80513070343558,2.34285510855967,4.4827064900244));
#17958=CARTESIAN_POINT('Ctrl Pts',(-3.80562878067403,2.40016339023914,4.47959252805377));
#17959=CARTESIAN_POINT('Ctrl Pts',(-3.80581594649383,2.40000082771776,4.55540747194623));
#17960=CARTESIAN_POINT('Ctrl Pts',(-3.80581594913922,2.4000451187351,4.55540505953261));
#17961=CARTESIAN_POINT('Ctrl Pts',(-3.80579587912807,2.46810441912583,4.55169805076672));
#17962=CARTESIAN_POINT('Ctrl Pts',(-3.73158417538336,2.60413054603043,4.54428644564855));
#17963=CARTESIAN_POINT('Ctrl Pts',(-3.49986236476522,2.62126031969194,4.53317265659175));
#17964=CARTESIAN_POINT('Ctrl Pts',(-3.35979766713961,2.43586801331045,4.52205886753494));
#17965=CARTESIAN_POINT('Ctrl Pts',(-3.43959288921302,2.2176453079079,4.51094507847814));
#17966=CARTESIAN_POINT('Ctrl Pts',(-3.66621055822496,2.16633391955349,4.49983128942134));
#17967=CARTESIAN_POINT('Ctrl Pts',(-3.79336822071197,2.29085017253336,4.4913187539107));
#17968=CARTESIAN_POINT('Ctrl Pts',(-3.80551684683325,2.37944724113564,4.48651081475233));
#17969=CARTESIAN_POINT('Ctrl Pts',(-3.80534990670044,2.39982347234431,4.48540747194623));
#17970=CARTESIAN_POINT('Origin',(-3.6,2.4,5.35459252805377));
#17971=CARTESIAN_POINT('',(-3.80534749188876,2.40017600730441,4.62540747194623));
#17972=CARTESIAN_POINT('',(-3.80545679372687,2.39981210841117,4.61959252805377));
#17973=CARTESIAN_POINT('',(-3.805475,2.40000000000001,5.35459252805377));
#17974=CARTESIAN_POINT('Ctrl Pts',(-3.80545679372687,2.39981210841117,4.61959252805377));
#17975=CARTESIAN_POINT('Ctrl Pts',(-3.80498629190864,2.45149295693423,4.61679038323268));
#17976=CARTESIAN_POINT('Ctrl Pts',(-3.75902063818539,2.5722445101987,4.61028364205933));
#17977=CARTESIAN_POINT('Ctrl Pts',(-3.55620097488638,2.63888348417682,4.60007230453371));
#17978=CARTESIAN_POINT('Ctrl Pts',(-3.3755463800872,2.4927590756963,4.58895851547691));
#17979=CARTESIAN_POINT('Ctrl Pts',(-3.40033672906513,2.26173123324197,4.5778447264201));
#17980=CARTESIAN_POINT('Ctrl Pts',(-3.60788113427776,2.15726236113484,4.5667309373633));
#17981=CARTESIAN_POINT('Ctrl Pts',(-3.77763371313004,2.25700670057819,4.55731353790785));
#17982=CARTESIAN_POINT('Ctrl Pts',(-3.80507586227844,2.36286981549731,4.55160073480468));
#17983=CARTESIAN_POINT('Ctrl Pts',(-3.80515175559583,2.40004689761323,4.54959252805377));
#17984=CARTESIAN_POINT('Ctrl Pts',(-3.80534749188876,2.40017600730441,4.62540747194623));
#17985=CARTESIAN_POINT('Ctrl Pts',(-3.80551452420589,2.42064195120264,4.62429930431288));
#17986=CARTESIAN_POINT('Ctrl Pts',(-3.79329841012664,2.50933048388748,4.61948654032726));
#17987=CARTESIAN_POINT('Ctrl Pts',(-3.66590691767206,2.63375190534549,4.61096917998937));
#17988=CARTESIAN_POINT('Ctrl Pts',(-3.43935610442817,2.58214613327058,4.59985539093257));
#17989=CARTESIAN_POINT('Ctrl Pts',(-3.35984447062414,2.36381993973287,4.58874160187577));
#17990=CARTESIAN_POINT('Ctrl Pts',(-3.50014991641224,2.17860976567263,4.57762781281897));
#17991=CARTESIAN_POINT('Ctrl Pts',(-3.73179898227351,2.19603680019893,4.56651643617579));
#17992=CARTESIAN_POINT('Ctrl Pts',(-3.80581188677276,2.33203010689162,4.55910965588488));
#17993=CARTESIAN_POINT('Ctrl Pts',(-3.80581594649383,2.40000082771776,4.55540747194623));
#17994=CARTESIAN_POINT('Origin',(-3.6,2.4,5.35459252805377));
#17995=CARTESIAN_POINT('',(-3.80519403776112,2.3998960891277,4.69540747194623));
#17996=CARTESIAN_POINT('',(-3.80578859626649,2.40006787741036,4.68959252805377));
#17997=CARTESIAN_POINT('',(-3.805475,2.40000000000001,5.35459252805377));
#17998=CARTESIAN_POINT('Ctrl Pts',(-3.80578859626649,2.40006787741036,4.68959252805377));
#17999=CARTESIAN_POINT('Ctrl Pts',(-3.80580466836371,2.40380178606869,4.68938922436523));
#18000=CARTESIAN_POINT('Ctrl Pts',(-3.8040203778982,2.4755592442775,4.68548132432442));
#18001=CARTESIAN_POINT('Ctrl Pts',(-3.7203544535977,2.61094662622203,4.67786882793133));
#18002=CARTESIAN_POINT('Ctrl Pts',(-3.48804541599454,2.61552226041731,4.66675503887454));
#18003=CARTESIAN_POINT('Ctrl Pts',(-3.35820967878295,2.42282792546417,4.65564124981773));
#18004=CARTESIAN_POINT('Ctrl Pts',(-3.44968736466998,2.20923893144694,4.64452746076093));
#18005=CARTESIAN_POINT('Ctrl Pts',(-3.67874791033599,2.17025570685489,4.63341367170413));
#18006=CARTESIAN_POINT('Ctrl Pts',(-3.79614945128685,2.2983686897146,4.62510202746841));
#18007=CARTESIAN_POINT('Ctrl Pts',(-3.80560832232849,2.38316790767908,4.62049497958495));
#18008=CARTESIAN_POINT('Ctrl Pts',(-3.80545679372687,2.39981210841117,4.61959252805377));
#18009=CARTESIAN_POINT('Ctrl Pts',(-3.80519403776112,2.3998960891277,4.69540747194623));
#18010=CARTESIAN_POINT('Ctrl Pts',(-3.80500643965891,2.44086040425288,4.69319354909316));
#18011=CARTESIAN_POINT('Ctrl Pts',(-3.77326722861529,2.55063877508332,4.68727502988781));
#18012=CARTESIAN_POINT('Ctrl Pts',(-3.59442944478611,2.64280165560495,4.6776519143302));
#18013=CARTESIAN_POINT('Ctrl Pts',(-3.39298749751263,2.52700196401557,4.6665381252734));
#18014=CARTESIAN_POINT('Ctrl Pts',(-3.38102644144724,2.29495593446246,4.65542433621659));
#18015=CARTESIAN_POINT('Ctrl Pts',(-3.56949436685434,2.15905792937668,4.64431054715979));
#18016=CARTESIAN_POINT('Ctrl Pts',(-3.76430796130134,2.23525748954489,4.63430492573634));
#18017=CARTESIAN_POINT('Ctrl Pts',(-3.80495613638248,2.352224449347,4.62800390066515));
#18018=CARTESIAN_POINT('Ctrl Pts',(-3.80534749188876,2.40017600730441,4.62540747194623));
#18019=CARTESIAN_POINT('Origin',(-3.6,2.4,5.35459252805377));
#18020=CARTESIAN_POINT('',(-3.80572670757095,2.39987978133106,4.76540747194623));
#18021=CARTESIAN_POINT('',(-3.8052563985153,2.4001450986671,4.75959252805377));
#18022=CARTESIAN_POINT('',(-3.805475,2.40000000000001,5.35459252805377));
#18023=CARTESIAN_POINT('Ctrl Pts',(-3.8052563985153,2.4001450986671,4.75959252805377));
#18024=CARTESIAN_POINT('Ctrl Pts',(-3.80541421064946,2.4243482217442,4.7582834691455));
#18025=CARTESIAN_POINT('Ctrl Pts',(-3.79026314769432,2.51685423684082,4.75326981388497));
#18026=CARTESIAN_POINT('Ctrl Pts',(-3.65317165905879,2.6369735181158,4.74455156227217));
#18027=CARTESIAN_POINT('Ctrl Pts',(-3.42974255082951,2.57319374878213,4.73343777321536));
#18028=CARTESIAN_POINT('Ctrl Pts',(-3.36215201667677,2.35088777703746,4.72232398415856));
#18029=CARTESIAN_POINT('Ctrl Pts',(-3.51226643903938,2.1735347799409,4.71121019510176));
#18030=CARTESIAN_POINT('Ctrl Pts',(-3.73846936695489,2.20292040156477,4.70029970973349));
#18031=CARTESIAN_POINT('Ctrl Pts',(-3.80551180288158,2.33576256604952,4.6930938207175));
#18032=CARTESIAN_POINT('Ctrl Pts',(-3.80578859626649,2.40006787741036,4.68959252805377));
#18033=CARTESIAN_POINT('Ctrl Pts',(-3.80572670757095,2.39987978133106,4.76540747194623));
#18034=CARTESIAN_POINT('Ctrl Pts',(-3.80530256520545,2.46089806692785,4.76208779387343));
#18035=CARTESIAN_POINT('Ctrl Pts',(-3.74420122965308,2.59074745124221,4.75506351944836));
#18036=CARTESIAN_POINT('Ctrl Pts',(-3.52344221510783,2.63048336300545,4.74433464867103));
#18037=CARTESIAN_POINT('Ctrl Pts',(-3.36483726729874,2.46068083880743,4.73322085961422));
#18038=CARTESIAN_POINT('Ctrl Pts',(-3.42147943565789,2.23533645468145,4.72210707055742));
#18039=CARTESIAN_POINT('Ctrl Pts',(-3.64152350112028,2.16071048099716,4.71099328150062));
#18040=CARTESIAN_POINT('Ctrl Pts',(-3.7872979195691,2.27634402063526,4.70209341529689));
#18041=CARTESIAN_POINT('Ctrl Pts',(-3.80532035088855,2.37231408965339,4.69689814544543));
#18042=CARTESIAN_POINT('Ctrl Pts',(-3.80519403776112,2.3998960891277,4.69540747194623));
#18043=CARTESIAN_POINT('Origin',(-3.6,2.4,5.35459252805377));
#18044=CARTESIAN_POINT('',(-3.80555825533459,2.40017991403412,4.83540747194623));
#18045=CARTESIAN_POINT('',(-3.80526423105652,2.39985120339831,4.82959252805377));
#18046=CARTESIAN_POINT('',(-3.805475,2.40000000000001,5.35459252805377));
#18047=CARTESIAN_POINT('Ctrl Pts',(-3.80526423105652,2.39985120339831,4.82959252805377));
#18048=CARTESIAN_POINT('Ctrl Pts',(-3.80496496310342,2.44449429497159,4.82717771392578));
#18049=CARTESIAN_POINT('Ctrl Pts',(-3.76870077292898,2.55806758042747,4.82105830344552));
#18050=CARTESIAN_POINT('Ctrl Pts',(-3.58130943065524,2.64214527918755,4.81123429661299));
#18051=CARTESIAN_POINT('Ctrl Pts',(-3.38642339103422,2.51562311930547,4.80012050755619));
#18052=CARTESIAN_POINT('Ctrl Pts',(-3.38702644372307,2.28326980706774,4.78900671849939));
#18053=CARTESIAN_POINT('Ctrl Pts',(-3.58256660775658,2.15776096423133,4.77789292944257));
#18054=CARTESIAN_POINT('Ctrl Pts',(-3.76915215745557,2.24264335554317,4.76808819929404));
#18055=CARTESIAN_POINT('Ctrl Pts',(-3.80496760717513,2.35585412961529,4.76198806549777));
#18056=CARTESIAN_POINT('Ctrl Pts',(-3.8052563985153,2.4001450986671,4.75959252805377));
#18057=CARTESIAN_POINT('Ctrl Pts',(-3.80555825533459,2.40017991403412,4.83540747194623));
#18058=CARTESIAN_POINT('Ctrl Pts',(-3.80567994271202,2.41345772088563,4.83468663500598));
#18059=CARTESIAN_POINT('Ctrl Pts',(-3.79845785744155,2.49484232907173,4.83026120171345));
#18060=CARTESIAN_POINT('Ctrl Pts',(-3.68988494016744,2.62561997380774,4.82213117206865));
#18061=CARTESIAN_POINT('Ctrl Pts',(-3.45919254257122,2.59788111325323,4.81101738301186));
#18062=CARTESIAN_POINT('Ctrl Pts',(-3.35738280762477,2.38901942561361,4.79990359395505));
#18063=CARTESIAN_POINT('Ctrl Pts',(-3.47764334032546,2.19020838223802,4.78878980489825));
#18064=CARTESIAN_POINT('Ctrl Pts',(-3.70989831124516,2.18342198579874,4.77767601584144));
#18065=CARTESIAN_POINT('Ctrl Pts',(-3.8022342613798,2.31768599661427,4.76988190485744));
#18066=CARTESIAN_POINT('Ctrl Pts',(-3.80577588708354,2.39280468157954,4.7657923902257));
#18067=CARTESIAN_POINT('Ctrl Pts',(-3.80572670757095,2.39987978133106,4.76540747194623));
#18068=CARTESIAN_POINT('Origin',(-3.6,2.4,5.35459252805377));
#18069=CARTESIAN_POINT('',(-3.80514216591097,2.40000781019071,4.90540747194623));
#18070=CARTESIAN_POINT('',(-3.8057933217542,2.39993826202139,4.89959252805377));
#18071=CARTESIAN_POINT('',(-3.805475,2.40000000000001,5.35459252805377));
#18072=CARTESIAN_POINT('Ctrl Pts',(-3.8057933217542,2.39993826202139,4.89959252805377));
#18073=CARTESIAN_POINT('Ctrl Pts',(-3.80553738483576,2.46459365390411,4.89607195870605));
#18074=CARTESIAN_POINT('Ctrl Pts',(-3.73784442289473,2.59774586534896,4.88884679300607));
#18075=CARTESIAN_POINT('Ctrl Pts',(-3.51109208760397,2.62600676257303,4.87791703095382));
#18076=CARTESIAN_POINT('Ctrl Pts',(-3.36190028978558,2.44787694237367,4.86680324189701));
#18077=CARTESIAN_POINT('Ctrl Pts',(-3.43064385696086,2.2259248138587,4.85568945284022));
#18078=CARTESIAN_POINT('Ctrl Pts',(-3.65440102248913,2.16330567736551,4.8445756637834));
#18079=CARTESIAN_POINT('Ctrl Pts',(-3.7905654137645,2.28386779123864,4.83587668885459));
#18080=CARTESIAN_POINT('Ctrl Pts',(-3.80542407378798,2.37600677360117,4.83088231027805));
#18081=CARTESIAN_POINT('Ctrl Pts',(-3.80526423105652,2.39985120339831,4.82959252805377));
#18082=CARTESIAN_POINT('Ctrl Pts',(-3.80514216591096,2.40000781019071,4.90540747194623));
#18083=CARTESIAN_POINT('Ctrl Pts',(-3.80515363190124,2.43382668369574,4.90358087978625));
#18084=CARTESIAN_POINT('Ctrl Pts',(-3.78123591260341,2.53621991664107,4.898049691274));
#18085=CARTESIAN_POINT('Ctrl Pts',(-3.6197380796992,2.64206214751696,4.88881390640948));
#18086=CARTESIAN_POINT('Ctrl Pts',(-3.40733479453568,2.54786410535795,4.87770011735268));
#18087=CARTESIAN_POINT('Ctrl Pts',(-3.37128015690807,2.3183243706747,4.86658632829587));
#18088=CARTESIAN_POINT('Ctrl Pts',(-3.54457538552076,2.16354326577609,4.85547253923908));
#18089=CARTESIAN_POINT('Ctrl Pts',(-3.75407113442107,2.22119506367479,4.84507958712252));
#18090=CARTESIAN_POINT('Ctrl Pts',(-3.80505455493103,2.34521910535256,4.83839123135824));
#18091=CARTESIAN_POINT('Ctrl Pts',(-3.80555825533459,2.40017991403412,4.83540747194623));
#18092=CARTESIAN_POINT('Origin',(-3.6,2.4,5.35459252805377));
#18093=CARTESIAN_POINT('',(-3.80552958623817,2.39981603086253,4.97540747194623));
#18094=CARTESIAN_POINT('',(-3.8054461347863,2.4001877030526,4.96959252805377));
#18095=CARTESIAN_POINT('',(-3.805475,2.40000000000001,5.35459252805377));
#18096=CARTESIAN_POINT('Ctrl Pts',(-3.80544613478631,2.4001877030526,4.96959252805377));
#18097=CARTESIAN_POINT('Ctrl Pts',(-3.8056000456266,2.41718968004276,4.9686707998386));
#18098=CARTESIAN_POINT('Ctrl Pts',(-3.79589308272504,2.50235240455911,4.96404447527116));
#18099=CARTESIAN_POINT('Ctrl Pts',(-3.67755429503925,2.63014996180817,4.95571355435145));
#18100=CARTESIAN_POINT('Ctrl Pts',(-3.44869918906956,2.58997825726379,4.94459976529464));
#18101=CARTESIAN_POINT('Ctrl Pts',(-3.35833143120733,2.37591729928569,4.93348597623784));
#18102=CARTESIAN_POINT('Ctrl Pts',(-3.48916565507154,2.18389951041786,4.92237218718103));
#18103=CARTESIAN_POINT('Ctrl Pts',(-3.72144781179447,2.18968095039579,4.91125839812423));
#18104=CARTESIAN_POINT('Ctrl Pts',(-3.80419976151153,2.32515687187029,4.90366517841514));
#18105=CARTESIAN_POINT('Ctrl Pts',(-3.80580670007452,2.39655859898363,4.89977655505832));
#18106=CARTESIAN_POINT('Ctrl Pts',(-3.8057933217542,2.39993826202139,4.89959252805377));
#18107=CARTESIAN_POINT('Ctrl Pts',(-3.80552958623817,2.39981603086253,4.97540747194623));
#18108=CARTESIAN_POINT('Ctrl Pts',(-3.80503092645118,2.45384921596595,4.97247512456653));
#18109=CARTESIAN_POINT('Ctrl Pts',(-3.75549941221135,2.57695439031686,4.96583818083456));
#18110=CARTESIAN_POINT('Ctrl Pts',(-3.54785414659174,2.63720135974049,4.9554966407503));
#18111=CARTESIAN_POINT('Ctrl Pts',(-3.37243277255298,2.48483414437987,4.94438285169351));
#18112=CARTESIAN_POINT('Ctrl Pts',(-3.40530626273826,2.25481727477052,4.9332690626367));
#18113=CARTESIAN_POINT('Ctrl Pts',(-3.61638513853951,2.15768779995451,4.9221552735799));
#18114=CARTESIAN_POINT('Ctrl Pts',(-3.78023981554385,2.2618608319249,4.91286807668307));
#18115=CARTESIAN_POINT('Ctrl Pts',(-3.80513037719409,2.36523705642733,4.90728547613852));
#18116=CARTESIAN_POINT('Ctrl Pts',(-3.80514216591096,2.40000781019071,4.90540747194623));
#18117=CARTESIAN_POINT('Origin',(-3.6,2.4,5.35459252805377));
#18118=CARTESIAN_POINT('',(-3.8057470998819,2.40010656251728,5.04540747194623));
#18119=CARTESIAN_POINT('',(-3.80515433183015,2.39994744458997,5.03959252805377));
#18120=CARTESIAN_POINT('',(-3.805475,2.40000000000001,5.35459252805377));
#18121=CARTESIAN_POINT('Ctrl Pts',(-3.80515433183015,2.39994744458997,5.03959252805377));
#18122=CARTESIAN_POINT('Ctrl Pts',(-3.80506840880667,2.4374802122161,5.03756504461887));
#18123=CARTESIAN_POINT('Ctrl Pts',(-3.77723759754696,2.54371107308321,5.03183296483171));
#18124=CARTESIAN_POINT('Ctrl Pts',(-3.60662102779949,2.64277527582587,5.02239628869227));
#18125=CARTESIAN_POINT('Ctrl Pts',(-3.39962169493761,2.53723049491962,5.01128249963547));
#18126=CARTESIAN_POINT('Ctrl Pts',(-3.3760308968172,2.30607708183528,5.00016871057867));
#18127=CARTESIAN_POINT('Ctrl Pts',(-3.55744155898554,2.16089238284251,4.98905492152186));
#18128=CARTESIAN_POINT('Ctrl Pts',(-3.75953036163254,2.22845546798632,4.97886286068023));
#18129=CARTESIAN_POINT('Ctrl Pts',(-3.80498144946327,2.34885558664921,4.97237539619086));
#18130=CARTESIAN_POINT('Ctrl Pts',(-3.80544613478631,2.4001877030526,4.96959252805377));
#18131=CARTESIAN_POINT('Ctrl Pts',(-3.8057470998819,2.40010656251728,5.04540747194623));
#18132=CARTESIAN_POINT('Ctrl Pts',(-3.80578578291066,2.40623506936011,5.04507396569907));
#18133=CARTESIAN_POINT('Ctrl Pts',(-3.80275767503742,2.48040043607423,5.04103586309964));
#18134=CARTESIAN_POINT('Ctrl Pts',(-3.71288602216703,2.61503584063672,5.03329316414794));
#18135=CARTESIAN_POINT('Ctrl Pts',(-3.48055937550073,2.61146539619723,5.02217937509113));
#18136=CARTESIAN_POINT('Ctrl Pts',(-3.35755806712823,2.4143382523336,5.01106558603433));
#18137=CARTESIAN_POINT('Ctrl Pts',(-3.45646661930996,2.20408715554039,4.99995179697752));
#18138=CARTESIAN_POINT('Ctrl Pts',(-3.68675289766315,2.17315730107164,4.98883800792072));
#18139=CARTESIAN_POINT('Ctrl Pts',(-3.79782383296962,2.3032367743191,4.98065656624362));
#18140=CARTESIAN_POINT('Ctrl Pts',(-3.80566091089323,2.38558610982074,4.97617972091879));
#18141=CARTESIAN_POINT('Ctrl Pts',(-3.80552958623817,2.39981603086253,4.97540747194623));
#18142=CARTESIAN_POINT('Origin',(-3.6,2.4,5.35459252805377));
#18143=CARTESIAN_POINT('',(-3.80520911606596,2.40011619915578,5.11540747194623));
#18144=CARTESIAN_POINT('',(-3.80563879690963,2.399839625535,5.10959252805377));
#18145=CARTESIAN_POINT('',(-3.805475,2.40000000000001,5.35459252805377));
#18146=CARTESIAN_POINT('Ctrl Pts',(-3.80563879690963,2.399839625535,5.10959252805377));
#18147=CARTESIAN_POINT('Ctrl Pts',(-3.805144032728,2.45749534173516,5.10645928939914));
#18148=CARTESIAN_POINT('Ctrl Pts',(-3.74979515516761,2.58415303951777,5.09962145439226));
#18149=CARTESIAN_POINT('Ctrl Pts',(-3.53510505788101,2.63403473315196,5.0890790230331));
#18150=CARTESIAN_POINT('Ctrl Pts',(-3.36817873292179,2.47240567046266,5.07796523397629));
#18151=CARTESIAN_POINT('Ctrl Pts',(-3.41344102170209,2.24450262655374,5.06685144491949));
#18152=CARTESIAN_POINT('Ctrl Pts',(-3.6294628695539,2.15892821683407,5.05573765586269));
#18153=CARTESIAN_POINT('Ctrl Pts',(-3.78402795283848,2.2693666686934,5.04665135024078));
#18154=CARTESIAN_POINT('Ctrl Pts',(-3.80522540644911,2.36890073499569,5.04126964097114));
#18155=CARTESIAN_POINT('Ctrl Pts',(-3.80515433183015,2.39994744458997,5.03959252805377));
#18156=CARTESIAN_POINT('Ctrl Pts',(-3.80520911606596,2.40011619915578,5.11540747194623));
#18157=CARTESIAN_POINT('Ctrl Pts',(-3.80534689450199,2.42674223668704,5.11396821047934));
#18158=CARTESIAN_POINT('Ctrl Pts',(-3.7881600578547,2.52173200460476,5.10882435266019));
#18159=CARTESIAN_POINT('Ctrl Pts',(-3.64483147349944,2.63869087951471,5.09997589848877));
#18160=CARTESIAN_POINT('Ctrl Pts',(-3.42377646220466,2.56711959422357,5.08886210943196));
#18161=CARTESIAN_POINT('Ctrl Pts',(-3.36401957377094,2.34258029572384,5.07774832037515));
#18162=CARTESIAN_POINT('Ctrl Pts',(-3.52025888482579,2.17059867951396,5.06663453131835));
#18163=CARTESIAN_POINT('Ctrl Pts',(-3.7426071061349,2.20745024082863,5.05585424850871));
#18164=CARTESIAN_POINT('Ctrl Pts',(-3.80535609078813,2.33815945072363,5.04877856205134));
#18165=CARTESIAN_POINT('Ctrl Pts',(-3.8057470998819,2.40010656251728,5.04540747194623));
#18166=CARTESIAN_POINT('Origin',(-3.6,2.4,5.35459252805377));
#18167=CARTESIAN_POINT('',(-3.80526708520764,2.39977040928181,5.18540747194623));
#18168=CARTESIAN_POINT('',(-3.80565732826014,2.40014993187889,5.17959252805377));
#18169=CARTESIAN_POINT('',(-3.805475,2.40000000000001,5.35459252805377));
#18170=CARTESIAN_POINT('',(-3.65301702171886,2.20148256743283,5.2));
#18171=CARTESIAN_POINT('Ctrl Pts',(-3.65301702171886,2.20148256743283,5.2));
#18172=CARTESIAN_POINT('Ctrl Pts',(-3.71902879097456,2.21911198848201,5.19629540364773));
#18173=CARTESIAN_POINT('Ctrl Pts',(-3.79249439061758,2.28872811842027,5.19143122762981));
#18174=CARTESIAN_POINT('Ctrl Pts',(-3.80542873353734,2.378346888084,5.18656705161189));
#18175=CARTESIAN_POINT('Ctrl Pts',(-3.80526708520764,2.39977040928181,5.18540747194623));
#18176=CARTESIAN_POINT('',(-3.54686846753247,2.20112677390461,5.2));
#18177=CARTESIAN_POINT('Origin',(-3.6,2.4,5.2));
#18178=CARTESIAN_POINT('Ctrl Pts',(-3.54686839490754,2.2011265482535,5.2));
#18179=CARTESIAN_POINT('Ctrl Pts',(-3.61132828593009,2.18399467910883,5.19636770818144));
#18180=CARTESIAN_POINT('Ctrl Pts',(-3.74930829171963,2.21593295369214,5.1895652175327));
#18181=CARTESIAN_POINT('Ctrl Pts',(-3.80517196370246,2.34184094054235,5.18276272688396));
#18182=CARTESIAN_POINT('Ctrl Pts',(-3.80565732826014,2.40014993187889,5.17959252805377));
#18183=CARTESIAN_POINT('Origin',(0.,-2.4,2.2));
#18184=CARTESIAN_POINT('',(7.34788079488412E-17,-2.8,2.8));
#18185=CARTESIAN_POINT('Origin',(0.,-2.8,2.2));
#18186=CARTESIAN_POINT('',(7.34788079488412E-17,-2.,2.8));
#18187=CARTESIAN_POINT('',(7.34788079488412E-17,-2.4,2.8));
#18188=CARTESIAN_POINT('Origin',(0.,-2.,2.2));
#18189=CARTESIAN_POINT('Origin',(-2.4,1.,0.4));
#18190=CARTESIAN_POINT('',(-2.,1.,0.4));
#18191=CARTESIAN_POINT('Origin',(-2.4,1.,0.4));
#18192=CARTESIAN_POINT('',(-2.15,1.,0.4));
#18193=CARTESIAN_POINT('Origin',(-2.4,1.,0.4));
#18194=CARTESIAN_POINT('Origin',(-2.4,1.,0.2));
#18195=CARTESIAN_POINT('',(-2.,1.,0.));
#18196=CARTESIAN_POINT('Origin',(-2.4,1.,0.));
#18197=CARTESIAN_POINT('',(-2.,1.,0.2));
#18198=CARTESIAN_POINT('Origin',(-2.4,1.,0.4));
#18199=CARTESIAN_POINT('',(-2.15,1.,0.8));
#18200=CARTESIAN_POINT('',(-2.15,1.,0.4));
#18201=CARTESIAN_POINT('Origin',(-2.4,1.,0.8));
#18202=CARTESIAN_POINT('Origin',(2.4,1.,0.4));
#18203=CARTESIAN_POINT('',(2.8,1.,0.4));
#18204=CARTESIAN_POINT('Origin',(2.4,1.,0.4));
#18205=CARTESIAN_POINT('',(2.65,1.,0.4));
#18206=CARTESIAN_POINT('Origin',(2.4,1.,0.4));
#18207=CARTESIAN_POINT('Origin',(2.4,1.,0.2));
#18208=CARTESIAN_POINT('',(2.8,1.,0.));
#18209=CARTESIAN_POINT('Origin',(2.4,1.,0.));
#18210=CARTESIAN_POINT('',(2.8,1.,0.2));
#18211=CARTESIAN_POINT('Origin',(2.4,1.,0.4));
#18212=CARTESIAN_POINT('',(2.65,1.,0.8));
#18213=CARTESIAN_POINT('',(2.65,1.,0.4));
#18214=CARTESIAN_POINT('Origin',(2.4,1.,0.8));
#18215=CARTESIAN_POINT('Origin',(-3.6,2.4,4.3));
#18216=CARTESIAN_POINT('Ctrl Pts',(-3.76351293272515,2.3680769545372,4.3));
#18217=CARTESIAN_POINT('Ctrl Pts',(-3.76286871316717,2.35978063266222,4.3));
#18218=CARTESIAN_POINT('Ctrl Pts',(-3.76155560899202,2.35157023575845,4.3));
#18219=CARTESIAN_POINT('Ctrl Pts',(-3.75963220387653,2.34349709858594,4.3));
#18220=CARTESIAN_POINT('Ctrl Pts',(-3.75857027766629,2.33903985975814,4.3));
#18221=CARTESIAN_POINT('Ctrl Pts',(-3.75732203034493,2.33462439532847,4.3));
#18222=CARTESIAN_POINT('Ctrl Pts',(-3.75589532649161,2.33025917511629,4.3));
#18223=CARTESIAN_POINT('Ctrl Pts',(-3.75435560971578,2.32554817445892,4.3));
#18224=CARTESIAN_POINT('Ctrl Pts',(-3.75261043848503,2.32090359735875,4.3));
#18225=CARTESIAN_POINT('Ctrl Pts',(-3.75067344213558,2.31634215529567,4.3));
#18226=CARTESIAN_POINT('Ctrl Pts',(-3.74745267041618,2.30875754441053,4.3));
#18227=CARTESIAN_POINT('Ctrl Pts',(-3.74370039609997,2.30139711771457,4.3));
#18228=CARTESIAN_POINT('Ctrl Pts',(-3.73945961576596,2.29430909563144,4.3));
#18229=CARTESIAN_POINT('Ctrl Pts',(-3.73760645031824,2.29121172284092,4.3));
#18230=CARTESIAN_POINT('Ctrl Pts',(-3.73566013813008,2.28816728583911,4.3));
#18231=CARTESIAN_POINT('Ctrl Pts',(-3.73363014813367,2.28518827452246,4.3));
#18232=CARTESIAN_POINT('Ctrl Pts',(-3.72675415090804,2.27509774521709,4.3));
#18233=CARTESIAN_POINT('Ctrl Pts',(-3.71890632139719,2.26572975853371,4.3));
#18234=CARTESIAN_POINT('Ctrl Pts',(-3.71022045861654,2.25723279915054,4.3));
#18235=CARTESIAN_POINT('Ctrl Pts',(-3.7059906475113,2.25309497956169,4.3));
#18236=CARTESIAN_POINT('Ctrl Pts',(-3.70156132140551,2.2491639079058,4.3));
#18237=CARTESIAN_POINT('Ctrl Pts',(-3.6969439956845,2.24545878490313,4.3));
#18238=CARTESIAN_POINT('Ctrl Pts',(-3.69303802929494,2.24232448448942,4.3));
#18239=CARTESIAN_POINT('Ctrl Pts',(-3.68899297342194,2.23934940616711,4.3));
#18240=CARTESIAN_POINT('Ctrl Pts',(-3.68484121061819,2.23656266363051,4.3));
#18241=CARTESIAN_POINT('Ctrl Pts',(-3.67976592507208,2.23315603498015,4.3));
#18242=CARTESIAN_POINT('Ctrl Pts',(-3.6745257104219,2.23002554470273,4.3));
#18243=CARTESIAN_POINT('Ctrl Pts',(-3.66913582629221,2.22718930926681,4.3));
#18244=CARTESIAN_POINT('Ctrl Pts',(-3.6615627323528,2.22320423706977,4.3));
#18245=CARTESIAN_POINT('Ctrl Pts',(-3.65369447955584,2.21979946771843,4.3));
#18246=CARTESIAN_POINT('Ctrl Pts',(-3.64559786041243,2.21695927257373,4.3));
#18247=CARTESIAN_POINT('Ctrl Pts',(-3.6396877011334,2.21488606085518,4.3));
#18248=CARTESIAN_POINT('Ctrl Pts',(-3.63365563048822,2.21311388420288,4.3));
#18249=CARTESIAN_POINT('Ctrl Pts',(-3.62752539225901,2.21164027047228,4.3));
#18250=CARTESIAN_POINT('Ctrl Pts',(-3.62399744472375,2.21079220686783,4.3));
#18251=CARTESIAN_POINT('Ctrl Pts',(-3.62044147481098,2.2100443281221,4.3));
#18252=CARTESIAN_POINT('Ctrl Pts',(-3.61687028704666,2.20939689951074,4.3));
#18253=CARTESIAN_POINT('Ctrl Pts',(-3.605353381675,2.20730897399576,4.3));
#18254=CARTESIAN_POINT('Ctrl Pts',(-3.59365536798806,2.20625732317521,4.3));
#18255=CARTESIAN_POINT('Ctrl Pts',(-3.58193303067035,2.20620865478203,4.3));
#18256=CARTESIAN_POINT('Ctrl Pts',(-3.57526869322992,2.20618098601718,4.3));
#18257=CARTESIAN_POINT('Ctrl Pts',(-3.56859610554753,2.20647808326505,4.3));
#18258=CARTESIAN_POINT('Ctrl Pts',(-3.5619424077193,2.20709864598645,4.3));
#18259=CARTESIAN_POINT('Ctrl Pts',(-3.55784552037318,2.20748074562885,4.3));
#18260=CARTESIAN_POINT('Ctrl Pts',(-3.55375372321261,2.20798587206127,4.3));
#18261=CARTESIAN_POINT('Ctrl Pts',(-3.54967985340644,2.20861337807665,4.3));
#18262=CARTESIAN_POINT('Ctrl Pts',(-3.53642392777045,2.21065521384261,4.3));
#18263=CARTESIAN_POINT('Ctrl Pts',(-3.52344437883893,2.21397442298982,4.3));
#18264=CARTESIAN_POINT('Ctrl Pts',(-3.51095539964347,2.2185383760968,4.3));
#18265=CARTESIAN_POINT('Ctrl Pts',(-3.50062245090115,2.22231443279277,4.3));
#18266=CARTESIAN_POINT('Ctrl Pts',(-3.49062431451358,2.22694342333832,4.3));
#18267=CARTESIAN_POINT('Ctrl Pts',(-3.48108410337466,2.23243384161104,4.3));
#18268=CARTESIAN_POINT('Ctrl Pts',(-3.47992982403391,2.23309813260964,4.3));
#18269=CARTESIAN_POINT('Ctrl Pts',(-3.47878225959784,2.23377506397182,4.3));
#18270=CARTESIAN_POINT('Ctrl Pts',(-3.47764149019701,2.2344644673347,4.3));
#18271=CARTESIAN_POINT('Ctrl Pts',(-3.41173724903364,2.31767678198965,4.3));
#18272=CARTESIAN_POINT('Ctrl Pts',(-3.40908132667977,2.32572936887695,4.3));
#18273=CARTESIAN_POINT('Ctrl Pts',(-3.40697195743913,2.3339396046188,4.3));
#18274=CARTESIAN_POINT('Ctrl Pts',(-3.40539675516275,2.34225613248928,4.3));
#18275=CARTESIAN_POINT('Ctrl Pts',(-3.40421042715,2.34851953759571,4.3));
#18276=CARTESIAN_POINT('Ctrl Pts',(-3.40332726918042,2.35484328996956,4.3));
#18277=CARTESIAN_POINT('Ctrl Pts',(-3.40274510142185,2.36120518228067,4.3));
#18278=CARTESIAN_POINT('Ctrl Pts',(-3.40230911384944,2.36596962679656,4.3));
#18279=CARTESIAN_POINT('Ctrl Pts',(-3.40204239822336,2.37075409356134,4.3));
#18280=CARTESIAN_POINT('Ctrl Pts',(-3.40194406709946,2.37553699140669,4.3));
#18281=CARTESIAN_POINT('Ctrl Pts',(-3.40173837831389,2.38554184450123,4.3));
#18282=CARTESIAN_POINT('Ctrl Pts',(-3.40226689742789,2.39555478383888,4.3));
#18283=CARTESIAN_POINT('Ctrl Pts',(-3.40352192589958,2.40548747856692,4.3));
#18284=CARTESIAN_POINT('Ctrl Pts',(-3.40417748512669,2.41067578291694,4.3));
#18285=CARTESIAN_POINT('Ctrl Pts',(-3.40503255607762,2.41584510393915,4.3));
#18286=CARTESIAN_POINT('Ctrl Pts',(-3.40608151604784,2.42095776789691,4.3));
#18287=CARTESIAN_POINT('Ctrl Pts',(-3.40864845689543,2.4334691184973,4.3));
#18288=CARTESIAN_POINT('Ctrl Pts',(-3.41237570095201,2.44567367466126,4.3));
#18289=CARTESIAN_POINT('Ctrl Pts',(-3.41724958122609,2.45738288213971,4.3));
#18290=CARTESIAN_POINT('Ctrl Pts',(-3.41948715125122,2.46275851104282,4.3));
#18291=CARTESIAN_POINT('Ctrl Pts',(-3.42196701213329,2.46802938689262,4.3));
#18292=CARTESIAN_POINT('Ctrl Pts',(-3.4246907645117,2.47317480637784,4.3));
#18293=CARTESIAN_POINT('Ctrl Pts',(-3.42647139059006,2.47653857328711,4.3));
#18294=CARTESIAN_POINT('Ctrl Pts',(-3.42835735887431,2.47985042338477,4.3));
#18295=CARTESIAN_POINT('Ctrl Pts',(-3.43034607421528,2.48309853180527,4.3));
#18296=CARTESIAN_POINT('Ctrl Pts',(-3.4346184872232,2.49007653432835,4.3));
#18297=CARTESIAN_POINT('Ctrl Pts',(-3.43934735204432,2.49673388406761,4.3));
#18298=CARTESIAN_POINT('Ctrl Pts',(-3.44453054699271,2.50301823813816,4.3));
#18299=CARTESIAN_POINT('Ctrl Pts',(-3.45023589251222,2.50993567259632,4.3));
#18300=CARTESIAN_POINT('Ctrl Pts',(-3.45649190823175,2.51640147868906,4.3));
#18301=CARTESIAN_POINT('Ctrl Pts',(-3.46322632730094,2.52238265672963,4.3));
#18302=CARTESIAN_POINT('Ctrl Pts',(-3.46747028515846,2.52615193026038,4.3));
#18303=CARTESIAN_POINT('Ctrl Pts',(-3.47190440586361,2.52972849539073,4.3));
#18304=CARTESIAN_POINT('Ctrl Pts',(-3.4765114687556,2.53310132051434,4.3));
#18305=CARTESIAN_POINT('Ctrl Pts',(-3.47932494356125,2.53516106198772,4.3));
#18306=CARTESIAN_POINT('Ctrl Pts',(-3.48219950761294,2.53714209816472,4.3));
#18307=CARTESIAN_POINT('Ctrl Pts',(-3.48512412807744,2.53903826687632,4.3));
#18308=CARTESIAN_POINT('Ctrl Pts',(-3.49373597317477,2.5446217302422,4.3));
#18309=CARTESIAN_POINT('Ctrl Pts',(-3.50279826970664,2.54948377957132,4.3));
#18310=CARTESIAN_POINT('Ctrl Pts',(-3.51220207894208,2.55357333967367,4.3));
#18311=CARTESIAN_POINT('Ctrl Pts',(-3.5210279439966,2.5574115614721,4.3));
#18312=CARTESIAN_POINT('Ctrl Pts',(-3.53015530415702,2.56056927246177,4.3));
#18313=CARTESIAN_POINT('Ctrl Pts',(-3.53949459164804,2.56298239916129,4.3));
#18314=CARTESIAN_POINT('Ctrl Pts',(-3.54298202528158,2.5638834977967,4.3));
#18315=CARTESIAN_POINT('Ctrl Pts',(-3.54649047145145,2.5646782882288,4.3));
#18316=CARTESIAN_POINT('Ctrl Pts',(-3.55001192980026,2.5653638227639,4.3));
#18317=CARTESIAN_POINT('Ctrl Pts',(-3.56109314401874,2.567521041247,4.3));
#18318=CARTESIAN_POINT('Ctrl Pts',(-3.57231422450356,2.56860269457927,4.3));
#18319=CARTESIAN_POINT('Ctrl Pts',(-3.58352456323646,2.56851224856759,4.3));
#18320=CARTESIAN_POINT('Ctrl Pts',(-3.58970650036672,2.56846237214805,4.3));
#18321=CARTESIAN_POINT('Ctrl Pts',(-3.59588506606642,2.56805522595141,4.3));
#18322=CARTESIAN_POINT('Ctrl Pts',(-3.60203269728429,2.56726809931874,4.3));
#18323=CARTESIAN_POINT('Ctrl Pts',(-3.60310836212971,2.56713037400346,4.3));
#18324=CARTESIAN_POINT('Ctrl Pts',(-3.60418307356748,2.56698100334876,4.3));
#18325=CARTESIAN_POINT('Ctrl Pts',(-3.60525667864057,2.56682005840211,4.3));
#18326=CARTESIAN_POINT('Origin',(-3.6,2.4,5.35459252805377));
#18327=CARTESIAN_POINT('Ctrl Pts',(-3.80565732826014,2.40014993187889,5.17959252805377));
#18328=CARTESIAN_POINT('Ctrl Pts',(-3.80573914572043,2.40997902530624,5.17905813053169));
#18329=CARTESIAN_POINT('Ctrl Pts',(-3.80062938236564,2.48786313470717,5.17481913665734));
#18330=CARTESIAN_POINT('Ctrl Pts',(-3.70109553522054,2.62084298334156,5.16687554643073));
#18331=CARTESIAN_POINT('Ctrl Pts',(-3.46929950811782,2.60468896536386,5.15576175737392));
#18332=CARTESIAN_POINT('Ctrl Pts',(-3.35713783891219,2.401213058351,5.14464796831712));
#18333=CARTESIAN_POINT('Ctrl Pts',(-3.46726930372222,2.19661072251331,5.13353417926031));
#18334=CARTESIAN_POINT('Ctrl Pts',(-3.69889135748228,2.17818094124235,5.12242039020352));
#18335=CARTESIAN_POINT('Ctrl Pts',(-3.80021577778504,2.31073764355723,5.11443983980133));
#18336=CARTESIAN_POINT('Ctrl Pts',(-3.80572901899447,2.38932589169745,5.11016388575141));
#18337=CARTESIAN_POINT('Ctrl Pts',(-3.80563879690963,2.399839625535,5.10959252805377));
#18338=CARTESIAN_POINT('Ctrl Pts',(-3.80526708520764,2.39977040928181,5.18540747194623));
#18339=CARTESIAN_POINT('Ctrl Pts',(-3.80491230346332,2.4467902221928,5.18286245525962));
#18340=CARTESIAN_POINT('Ctrl Pts',(-3.76565540874154,2.56295294620881,5.17661284222074));
#18341=CARTESIAN_POINT('Ctrl Pts',(-3.57278676575927,2.64128531597693,5.16665863282959));
#18342=CARTESIAN_POINT('Ctrl Pts',(-3.38252462806861,2.5080933346037,5.15554484377278));
#18343=CARTESIAN_POINT('Ctrl Pts',(-3.39123766596766,2.27586209704876,5.14443105471597));
#18344=CARTESIAN_POINT('Ctrl Pts',(-3.59107442724388,2.15730569128375,5.13331726565918));
#18345=CARTESIAN_POINT('Ctrl Pts',(-3.77212564275939,2.247453977085,5.12364273806926));
#18346=CARTESIAN_POINT('Ctrl Pts',(-3.80499225880634,2.35820797534334,5.11767280683161));
#18347=CARTESIAN_POINT('Ctrl Pts',(-3.80520911606596,2.40011619915578,5.11540747194623));
#18348=CARTESIAN_POINT('Ctrl Pts',(-3.47309291201476,2.50793586530485,5.2));
#18349=CARTESIAN_POINT('Ctrl Pts',(-3.43720166889934,2.46573623930395,5.19629540364773));
#18350=CARTESIAN_POINT('Ctrl Pts',(-3.41147910372774,2.34341327692754,5.1888862109432));
#18351=CARTESIAN_POINT('Ctrl Pts',(-3.54548749138621,2.21065847912018,5.17777242188639));
#18352=CARTESIAN_POINT('Ctrl Pts',(-3.72942273074541,2.25164328799446,5.16665863282959));
#18353=CARTESIAN_POINT('Ctrl Pts',(-3.79487861203899,2.42820978532064,5.15554484377278));
#18354=CARTESIAN_POINT('Ctrl Pts',(-3.68196868800459,2.57906042596279,5.14443105471598));
#18355=CARTESIAN_POINT('Ctrl Pts',(-3.49402748778406,2.56596267978888,5.13331726565918));
#18356=CARTESIAN_POINT('Ctrl Pts',(-3.40308633148933,2.40098355284719,5.12220347660236));
#18357=CARTESIAN_POINT('Ctrl Pts',(-3.49238138946403,2.23509111264493,5.11108968754557));
#18358=CARTESIAN_POINT('Ctrl Pts',(-3.68018153136171,2.22014816795705,5.09997589848877));
#18359=CARTESIAN_POINT('Ctrl Pts',(-3.79459033398193,2.36982238810866,5.08886210943195));
#18360=CARTESIAN_POINT('Ctrl Pts',(-3.73088853410035,2.54712014517116,5.07774832037516));
#18361=CARTESIAN_POINT('Ctrl Pts',(-3.54738290615879,2.58975635256414,5.06663453131835));
#18362=CARTESIAN_POINT('Ctrl Pts',(-3.41203833510047,2.45870682418337,5.05552074226154));
#18363=CARTESIAN_POINT('Ctrl Pts',(-3.44873719048823,2.27392207121964,5.04440695320474));
#18364=CARTESIAN_POINT('Ctrl Pts',(-3.62388861938279,2.20453797748901,5.03329316414794));
#18365=CARTESIAN_POINT('Ctrl Pts',(-3.77717451978384,2.31406243911007,5.02217937509113));
#18366=CARTESIAN_POINT('Ctrl Pts',(-3.76829057505717,2.5022465500548,5.01106558603433));
#18367=CARTESIAN_POINT('Ctrl Pts',(-3.60536835737386,2.5968432215724,4.99995179697752));
#18368=CARTESIAN_POINT('Ctrl Pts',(-3.43753242183529,2.51126706632734,4.98883800792072));
#18369=CARTESIAN_POINT('Ctrl Pts',(-3.41840490283366,2.32384690027379,4.97772421886392));
#18370=CARTESIAN_POINT('Ctrl Pts',(-3.56549343582914,2.20613053160512,4.96661042980711));
#18371=CARTESIAN_POINT('Ctrl Pts',(-3.74416621827519,2.26586508520319,4.95549664075031));
#18372=CARTESIAN_POINT('Ctrl Pts',(-3.79088202621085,2.44837484789993,4.9443828516935));
#18373=CARTESIAN_POINT('Ctrl Pts',(-3.66288135078982,2.58660656351012,4.9332690626367));
#18374=CARTESIAN_POINT('Ctrl Pts',(-3.47732466187608,2.55403517537485,4.9221552735799));
#18375=CARTESIAN_POINT('Ctrl Pts',(-3.40405410117601,2.38047364429248,4.91104148452309));
#18376=CARTESIAN_POINT('Ctrl Pts',(-3.51013504384922,2.2247848080575,4.89992769546628));
#18377=CARTESIAN_POINT('Ctrl Pts',(-3.69847040002413,2.22947242407076,4.88881390640949));
#18378=CARTESIAN_POINT('Ctrl Pts',(-3.79667468232717,2.39024586425236,4.87770011735267));
#18379=CARTESIAN_POINT('Ctrl Pts',(-3.7148603974533,2.55994737550017,4.86658632829588));
#18380=CARTESIAN_POINT('Ctrl Pts',(-3.52791308818505,2.58324724002758,4.85547253923907));
#18381=CARTESIAN_POINT('Ctrl Pts',(-3.40694774682213,2.43881882759193,4.84435875018226));
#18382=CARTESIAN_POINT('Ctrl Pts',(-3.46268532215442,2.25885910202633,4.83324496112546));
#18383=CARTESIAN_POINT('Ctrl Pts',(-3.64410857937311,2.20808724102248,4.82213117206866));
#18384=CARTESIAN_POINT('Ctrl Pts',(-3.78515875366629,2.33297530474957,4.81101738301185));
#18385=CARTESIAN_POINT('Ctrl Pts',(-3.75673102088563,2.51921183215107,4.79990359395505));
#18386=CARTESIAN_POINT('Ctrl Pts',(-3.58484560723768,2.59633241763059,4.78878980489824));
#18387=CARTESIAN_POINT('Ctrl Pts',(-3.42683118114759,2.49374771469177,4.77767601584145));
#18388=CARTESIAN_POINT('Ctrl Pts',(-3.42732013882109,2.30535466532418,4.76656222678463));
#18389=CARTESIAN_POINT('Ctrl Pts',(-3.58586493175446,2.20359156413646,4.75544843772784));
#18390=CARTESIAN_POINT('Ctrl Pts',(-3.75734771295555,2.28160333171781,4.74433464867102));
#18391=CARTESIAN_POINT('Ctrl Pts',(-3.784808348044,2.46798491248738,4.73322085961423));
#18392=CARTESIAN_POINT('Ctrl Pts',(-3.64311180629855,2.59213913185591,4.72210707055742));
#18393=CARTESIAN_POINT('Ctrl Pts',(-3.46195453932691,2.54042622483077,4.71099328150062));
#18394=CARTESIAN_POINT('Ctrl Pts',(-3.40715184805135,2.36017960167632,4.69987949244381));
#18395=CARTESIAN_POINT('Ctrl Pts',(-3.52886525730118,2.21638104070156,4.688765703387));
#18396=CARTESIAN_POINT('Ctrl Pts',(-3.7156891032661,2.24065099555331,4.67765191433021));
#18397=CARTESIAN_POINT('Ctrl Pts',(-3.79662140100789,2.41077490131571,4.6665381252734));
#18398=CARTESIAN_POINT('Ctrl Pts',(-3.69758390056881,2.57103641770819,4.65542433621659));
#18399=CARTESIAN_POINT('Ctrl Pts',(-3.50922674926239,2.57474636128738,4.64431054715979));
#18400=CARTESIAN_POINT('Ctrl Pts',(-3.40395538379481,2.41850897862188,4.63319675810298));
#18401=CARTESIAN_POINT('Ctrl Pts',(-3.47812587883694,2.24533011791732,4.62208296904618));
#18402=CARTESIAN_POINT('Ctrl Pts',(-3.6638491391263,2.21372235435953,4.61096917998938));
#18403=CARTESIAN_POINT('Ctrl Pts',(-3.79113055827457,2.35261663238717,4.59985539093257));
#18404=CARTESIAN_POINT('Ctrl Pts',(-3.74346800986679,2.53488144415775,4.58874160187577));
#18405=CARTESIAN_POINT('Ctrl Pts',(-3.56448756498879,2.59368774042515,4.57762781281897));
#18406=CARTESIAN_POINT('Ctrl Pts',(-3.41801205461748,2.475209451325,4.56651402376216));
#18407=CARTESIAN_POINT('Ctrl Pts',(-3.4381121745334,2.28789109846994,4.55540023470536));
#18408=CARTESIAN_POINT('Ctrl Pts',(-3.60639005704185,2.20318729463469,4.54428644564855));
#18409=CARTESIAN_POINT('Ctrl Pts',(-3.76881904785141,2.29862839193225,4.53317265659175));
#18410=CARTESIAN_POINT('Ctrl Pts',(-3.77672604966501,2.48685607191854,4.52205886753494));
#18411=CARTESIAN_POINT('Ctrl Pts',(-3.62287369392911,2.59558340387831,4.51094507847814));
#18412=CARTESIAN_POINT('Ctrl Pts',(-3.44808478689753,2.52529102897173,4.49983128942133));
#18413=CARTESIAN_POINT('Ctrl Pts',(-3.41234559692803,2.34031835280842,4.48871750036453));
#18414=CARTESIAN_POINT('Ctrl Pts',(-3.54836861088932,2.20997296824294,4.47760371130773));
#18415=CARTESIAN_POINT('Ctrl Pts',(-3.73165041953522,2.2535614747159,4.46648992225092));
#18416=CARTESIAN_POINT('Ctrl Pts',(-3.79443110878254,2.431186836485,4.45537613319412));
#18417=CARTESIAN_POINT('Ctrl Pts',(-3.67924679391792,2.58026650835313,4.44426234413731));
#18418=CARTESIAN_POINT('Ctrl Pts',(-3.49152700036135,2.56434625038721,4.43314855508051));
#18419=CARTESIAN_POINT('Ctrl Pts',(-3.40309375251607,2.39799790627107,4.4220347660237));
#18420=CARTESIAN_POINT('Ctrl Pts',(-3.49489106815987,2.23348230018954,4.4109209769669));
#18421=CARTESIAN_POINT('Ctrl Pts',(-3.68289569684173,2.22138183485646,4.3998071879101));
#18422=CARTESIAN_POINT('Ctrl Pts',(-3.79502512287648,2.37277339930001,4.38869339885329));
#18423=CARTESIAN_POINT('Ctrl Pts',(-3.72864550427982,2.54908418322982,4.37757960979649));
#18424=CARTESIAN_POINT('Ctrl Pts',(-3.54451587329345,2.58893972093235,4.36646582073968));
#18425=CARTESIAN_POINT('Ctrl Pts',(-3.41117013795305,2.4558501873037,4.35535203168288));
#18426=CARTESIAN_POINT('Ctrl Pts',(-3.45066522941702,2.27165316239582,4.34423824262608));
#18427=CARTESIAN_POINT('Ctrl Pts',(-3.62684269841689,2.20490778718547,4.33312445356927));
#18428=CARTESIAN_POINT('Ctrl Pts',(-3.77846161969435,2.31678392154068,4.32201066451247));
#18429=CARTESIAN_POINT('Ctrl Pts',(-3.76671077264337,2.50472571563538,4.31089687545566));
#18430=CARTESIAN_POINT('Ctrl Pts',(-3.6024119571336,2.59701778495161,4.29978308639886));
#18431=CARTESIAN_POINT('Ctrl Pts',(-3.43581014038123,2.50855356077874,4.28866929734205));
#18432=CARTESIAN_POINT('Ctrl Pts',(-3.42516046182893,2.38400982617005,4.28126010463752));
#18433=CARTESIAN_POINT('Ctrl Pts',(-3.44735576439472,2.33325198627315,4.27755550828525));
#18434=CARTESIAN_POINT('Ctrl Pts',(-3.46322193753412,2.51633123698097,5.20748149723825));
#18435=CARTESIAN_POINT('Ctrl Pts',(-3.42453903360215,2.47084927712496,5.20377690088598));
#18436=CARTESIAN_POINT('Ctrl Pts',(-3.39681573869656,2.33901189865735,5.19636770818145));
#18437=CARTESIAN_POINT('Ctrl Pts',(-3.54124744782407,2.19593128499412,5.18525391912464));
#18438=CARTESIAN_POINT('Ctrl Pts',(-3.73948937471845,2.24010393789599,5.17414013006784));
#18439=CARTESIAN_POINT('Ctrl Pts',(-3.81003648727512,2.43040397380471,5.16302634101103));
#18440=CARTESIAN_POINT('Ctrl Pts',(-3.68834430374324,2.59298794508905,5.15191255195423));
#18441=CARTESIAN_POINT('Ctrl Pts',(-3.48578482789531,2.57887144164721,5.14079876289743));
#18442=CARTESIAN_POINT('Ctrl Pts',(-3.38777016729695,2.40106005468179,5.12968497384062));
#18443=CARTESIAN_POINT('Ctrl Pts',(-3.48401069421676,2.22226431593439,5.11857118478382));
#18444=CARTESIAN_POINT('Ctrl Pts',(-3.68641814006856,2.20615909238548,5.10745739572702));
#18445=CARTESIAN_POINT('Ctrl Pts',(-3.80972578663008,2.36747513988482,5.0963436066702));
#18446=CARTESIAN_POINT('Ctrl Pts',(-3.74106918988897,2.55856331372564,5.0852298176134));
#18447=CARTESIAN_POINT('Ctrl Pts',(-3.5432902900662,2.60451581276008,5.0741160285566));
#18448=CARTESIAN_POINT('Ctrl Pts',(-3.39741846770758,2.46327310627647,5.06300223949979));
#18449=CARTESIAN_POINT('Ctrl Pts',(-3.43697180089285,2.26411558966434,5.05188845044299));
#18450=CARTESIAN_POINT('Ctrl Pts',(-3.62574670277316,2.18933472393736,5.04077466138618));
#18451=CARTESIAN_POINT('Ctrl Pts',(-3.79095535102953,2.30737812002324,5.02966087232938));
#18452=CARTESIAN_POINT('Ctrl Pts',(-3.78138040319912,2.51019940046172,5.01854708327258));
#18453=CARTESIAN_POINT('Ctrl Pts',(-3.60578591418241,2.61215390632356,5.00743329421578));
#18454=CARTESIAN_POINT('Ctrl Pts',(-3.42489551286939,2.51992154252476,4.99631950515897));
#18455=CARTESIAN_POINT('Ctrl Pts',(-3.40428023416151,2.31792362746096,4.98520571610217));
#18456=CARTESIAN_POINT('Ctrl Pts',(-3.56280947688127,2.19105114868425,4.97409192704536));
#18457=CARTESIAN_POINT('Ctrl Pts',(-3.75537962710962,2.25543192231258,4.96297813798856));
#18458=CARTESIAN_POINT('Ctrl Pts',(-3.80572904255528,2.45213749738394,4.95186434893175));
#18459=CARTESIAN_POINT('Ctrl Pts',(-3.6677723322063,2.60112102960948,4.94075055987495));
#18460=CARTESIAN_POINT('Ctrl Pts',(-3.46778283760724,2.56601620267116,4.92963677081815));
#18461=CARTESIAN_POINT('Ctrl Pts',(-3.38881321118645,2.37895486262355,4.91852298176134));
#18462=CARTESIAN_POINT('Ctrl Pts',(-3.50314524759,2.21115637551095,4.90740919270453));
#18463=CARTESIAN_POINT('Ctrl Pts',(-3.70612953728091,2.21620859951243,4.89629540364773));
#18464=CARTESIAN_POINT('Ctrl Pts',(-3.81197225790835,2.38948717672297,4.88518161459093));
#18465=CARTESIAN_POINT('Ctrl Pts',(-3.72379436694309,2.57238826029923,4.87406782553412));
#18466=CARTESIAN_POINT('Ctrl Pts',(-3.52230608799136,2.5975004142094,4.86295403647732));
#18467=CARTESIAN_POINT('Ctrl Pts',(-3.39193192780995,2.44183819918584,4.85184024742051));
#18468=CARTESIAN_POINT('Ctrl Pts',(-3.45200483375657,2.24788100597045,4.84072645836371));
#18469=CARTESIAN_POINT('Ctrl Pts',(-3.64753939374511,2.19316005313682,4.8296126693069));
#18470=CARTESIAN_POINT('Ctrl Pts',(-3.79956060750538,2.3277620493917,4.81849888025011));
#18471=CARTESIAN_POINT('Ctrl Pts',(-3.76892173404475,2.52848426107239,4.80738509119329));
#18472=CARTESIAN_POINT('Ctrl Pts',(-3.5836668817102,2.61160337148291,4.7962713021365));
#18473=CARTESIAN_POINT('Ctrl Pts',(-3.41336191777647,2.50103951622967,4.78515751307969));
#18474=CARTESIAN_POINT('Ctrl Pts',(-3.41388890712174,2.29799304590536,4.77404372402289));
#18475=CARTESIAN_POINT('Ctrl Pts',(-3.58476549042184,2.18831469750142,4.76292993496608));
#18476=CARTESIAN_POINT('Ctrl Pts',(-3.76958639310991,2.27239430714904,4.75181614590928));
#18477=CARTESIAN_POINT('Ctrl Pts',(-3.79918294694398,2.47327285461012,4.74070235685247));
#18478=CARTESIAN_POINT('Ctrl Pts',(-3.64646509055197,2.60708392727588,4.72958856779567));
#18479=CARTESIAN_POINT('Ctrl Pts',(-3.45121720982778,2.55134873281456,4.71847477873886));
#18480=CARTESIAN_POINT('Ctrl Pts',(-3.39215190425982,2.3570823267967,4.70736098968206));
#18481=CARTESIAN_POINT('Ctrl Pts',(-3.52333231788058,2.20209895378134,4.69624720062526));
#18482=CARTESIAN_POINT('Ctrl Pts',(-3.7246875304159,2.22825665272044,4.68513341156845));
#18483=CARTESIAN_POINT('Ctrl Pts',(-3.81191483230877,2.41161298512653,4.67401962251165));
#18484=CARTESIAN_POINT('Ctrl Pts',(-3.70517408491178,2.58433982054614,4.66290583345484));
#18485=CARTESIAN_POINT('Ctrl Pts',(-3.50216630483977,2.58833832766402,4.65179204439804));
#18486=CARTESIAN_POINT('Ctrl Pts',(-3.38870681545753,2.41994862756931,4.64067825534123));
#18487=CARTESIAN_POINT('Ctrl Pts',(-3.46864637411461,2.23329972242719,4.62956446628443));
#18488=CARTESIAN_POINT('Ctrl Pts',(-3.6688153961962,2.19923347185799,4.61845067722763));
#18489=CARTESIAN_POINT('Ctrl Pts',(-3.80599690571939,2.34893110134286,4.60733688817082));
#18490=CARTESIAN_POINT('Ctrl Pts',(-3.7546271112745,2.54537267293252,4.59622309911402));
#18491=CARTESIAN_POINT('Ctrl Pts',(-3.56172536828799,2.60875298834237,4.58510931005721));
#18492=CARTESIAN_POINT('Ctrl Pts',(-3.40385682977405,2.48105932611543,4.57399552100042));
#18493=CARTESIAN_POINT('Ctrl Pts',(-3.42552035937731,2.27917114339395,4.5628817319436));
#18494=CARTESIAN_POINT('Ctrl Pts',(-3.60688708278715,2.18787898346807,4.5517679428868));
#18495=CARTESIAN_POINT('Ctrl Pts',(-3.7819499811952,2.2907435954864,4.54065415383));
#18496=CARTESIAN_POINT('Ctrl Pts',(-3.79047199840596,2.49361183381496,4.52954036477319));
#18497=CARTESIAN_POINT('Ctrl Pts',(-3.62465283528865,2.61079609860775,4.51842657571639));
#18498=CARTESIAN_POINT('Ctrl Pts',(-3.43626865262511,2.53503630458453,4.50731278665958));
#18499=CARTESIAN_POINT('Ctrl Pts',(-3.39774962870189,2.33567624789731,4.49619899760278));
#18500=CARTESIAN_POINT('Ctrl Pts',(-3.54435266400721,2.19519245431826,4.48508520854598));
#18501=CARTESIAN_POINT('Ctrl Pts',(-3.74189033562052,2.24217132331451,4.47397141948917));
#18502=CARTESIAN_POINT('Ctrl Pts',(-3.80955417671754,2.43361258332043,4.46285763043237));
#18503=CARTESIAN_POINT('Ctrl Pts',(-3.68541069770656,2.59428783790942,4.45174384137556));
#18504=CARTESIAN_POINT('Ctrl Pts',(-3.48308984977921,2.57712928456848,4.44063005231877));
#18505=CARTESIAN_POINT('Ctrl Pts',(-3.38777816553941,2.39784218119362,4.42951626326195));
#18506=CARTESIAN_POINT('Ctrl Pts',(-3.48671557851344,2.22053036825651,4.41840247420515));
#18507=CARTESIAN_POINT('Ctrl Pts',(-3.68934341635898,2.20748871526871,4.40728868514834));
#18508=CARTESIAN_POINT('Ctrl Pts',(-3.81019439388853,2.37065568400947,4.39617489609154));
#18509=CARTESIAN_POINT('Ctrl Pts',(-3.73865169471375,2.56068011684939,4.38506110703474));
#18510=CARTESIAN_POINT('Ctrl Pts',(-3.54020025619518,2.60363566261151,4.37394731797793));
#18511=CARTESIAN_POINT('Ctrl Pts',(-3.3964827412202,2.46019427700244,4.36283352892113));
#18512=CARTESIAN_POINT('Ctrl Pts',(-3.43904980483436,2.26167020258818,4.35171973986432));
#18513=CARTESIAN_POINT('Ctrl Pts',(-3.62893055336078,2.18973329784341,4.34060595080752));
#18514=CARTESIAN_POINT('Ctrl Pts',(-3.79234256300291,2.3103112823848,4.32949216175072));
#18515=CARTESIAN_POINT('Ctrl Pts',(-3.77967772199614,2.5128713982991,4.31837837269391));
#18516=CARTESIAN_POINT('Ctrl Pts',(-3.60259956184262,2.61234204743659,4.30726458363711));
#18517=CARTESIAN_POINT('Ctrl Pts',(-3.42303927044789,2.51699697749597,4.2961507945803));
#18518=CARTESIAN_POINT('Ctrl Pts',(-3.41156124805062,2.38276609266137,4.28874160187577));
#18519=CARTESIAN_POINT('Ctrl Pts',(-3.43548292594103,2.32806025151199,4.2850370055235));
#18520=CARTESIAN_POINT('Ctrl Pts',(-3.45335096305347,2.52472660865709,5.2149629944765));
#18521=CARTESIAN_POINT('Ctrl Pts',(-3.41187639830495,2.47596231494597,5.21125839812423));
#18522=CARTESIAN_POINT('Ctrl Pts',(-3.38215237366538,2.33461052038716,5.20384920541969));
#18523=CARTESIAN_POINT('Ctrl Pts',(-3.53700740426192,2.18120409086806,5.19273541636289));
#18524=CARTESIAN_POINT('Ctrl Pts',(-3.7495560186915,2.22856458779753,5.18162162730609));
#18525=CARTESIAN_POINT('Ctrl Pts',(-3.82519436251124,2.43259816228878,5.17050783824928));
#18526=CARTESIAN_POINT('Ctrl Pts',(-3.69471991948189,2.60691546421531,5.15939404919248));
#18527=CARTESIAN_POINT('Ctrl Pts',(-3.47754216800657,2.59178020350553,5.14828026013568));
#18528=CARTESIAN_POINT('Ctrl Pts',(-3.37245400310457,2.4011365565164,5.13716647107886));
#18529=CARTESIAN_POINT('Ctrl Pts',(-3.47563999896949,2.20943751922385,5.12605268202207));
#18530=CARTESIAN_POINT('Ctrl Pts',(-3.69265474877542,2.19217001681392,5.11493889296526));
#18531=CARTESIAN_POINT('Ctrl Pts',(-3.82486123927823,2.36512789166097,5.10382510390846));
#18532=CARTESIAN_POINT('Ctrl Pts',(-3.75124984567759,2.57000648228012,5.09271131485165));
#18533=CARTESIAN_POINT('Ctrl Pts',(-3.53919767397361,2.61927527295602,5.08159752579485));
#18534=CARTESIAN_POINT('Ctrl Pts',(-3.38279860031468,2.46783938836956,5.07048373673804));
#18535=CARTESIAN_POINT('Ctrl Pts',(-3.42520641129747,2.25430910810904,5.05936994768124));
#18536=CARTESIAN_POINT('Ctrl Pts',(-3.62760478616353,2.17413147038572,5.04825615862444));
#18537=CARTESIAN_POINT('Ctrl Pts',(-3.80473618227523,2.30069380093641,5.03714236956763));
#18538=CARTESIAN_POINT('Ctrl Pts',(-3.79447023134107,2.51815225086865,5.02602858051083));
#18539=CARTESIAN_POINT('Ctrl Pts',(-3.60620347099095,2.62746459107471,5.01491479145402));
#18540=CARTESIAN_POINT('Ctrl Pts',(-3.4122586039035,2.52857601872219,5.00380100239722));
#18541=CARTESIAN_POINT('Ctrl Pts',(-3.39015556548935,2.31200035464812,4.99268721334042));
#18542=CARTESIAN_POINT('Ctrl Pts',(-3.56012551793341,2.17597176576338,4.98157342428361));
#18543=CARTESIAN_POINT('Ctrl Pts',(-3.76659303594405,2.24499875942197,4.9704596352268));
#18544=CARTESIAN_POINT('Ctrl Pts',(-3.82057605889971,2.45590014686796,4.95934584617));
#18545=CARTESIAN_POINT('Ctrl Pts',(-3.67266331362277,2.61563549570883,4.94823205711319));
#18546=CARTESIAN_POINT('Ctrl Pts',(-3.4582410133384,2.57799722996748,4.93711826805639));
#18547=CARTESIAN_POINT('Ctrl Pts',(-3.37357232119689,2.37743608095462,4.92600447899959));
#18548=CARTESIAN_POINT('Ctrl Pts',(-3.49615545133077,2.19752794296441,4.91489068994278));
#18549=CARTESIAN_POINT('Ctrl Pts',(-3.71378867453769,2.20294477495411,4.90377690088598));
#18550=CARTESIAN_POINT('Ctrl Pts',(-3.82726983348952,2.38872848919359,4.89266311182918));
#18551=CARTESIAN_POINT('Ctrl Pts',(-3.73272833643288,2.58482914509829,4.88154932277237));
#18552=CARTESIAN_POINT('Ctrl Pts',(-3.51669908779767,2.61175358839122,4.87043553371557));
#18553=CARTESIAN_POINT('Ctrl Pts',(-3.37691610879776,2.44485757077975,4.85932174465876));
#18554=CARTESIAN_POINT('Ctrl Pts',(-3.44132434535872,2.23690290991458,4.84820795560196));
#18555=CARTESIAN_POINT('Ctrl Pts',(-3.65097020811712,2.17823286525116,4.83709416654515));
#18556=CARTESIAN_POINT('Ctrl Pts',(-3.81396246134447,2.32254879403384,4.82598037748835));
#18557=CARTESIAN_POINT('Ctrl Pts',(-3.78111244720387,2.5377566899937,4.81486658843155));
#18558=CARTESIAN_POINT('Ctrl Pts',(-3.58248815618272,2.62687432533523,4.80375279937474));
#18559=CARTESIAN_POINT('Ctrl Pts',(-3.39989265440535,2.50833131776757,4.79263901031794));
#18560=CARTESIAN_POINT('Ctrl Pts',(-3.4004576754224,2.29063142648655,4.78152522126113));
#18561=CARTESIAN_POINT('Ctrl Pts',(-3.58366604908921,2.17303783086637,4.77041143220433));
#18562=CARTESIAN_POINT('Ctrl Pts',(-3.78182507326426,2.26318528258027,4.75929764314753));
#18563=CARTESIAN_POINT('Ctrl Pts',(-3.81355754584396,2.47856079673287,4.74818385409072));
#18564=CARTESIAN_POINT('Ctrl Pts',(-3.64981837480538,2.62202872269584,4.73707006503392));
#18565=CARTESIAN_POINT('Ctrl Pts',(-3.44047988032865,2.56227124079834,4.72595627597711));
#18566=CARTESIAN_POINT('Ctrl Pts',(-3.3771519604683,2.35398505191708,4.71484248692031));
#18567=CARTESIAN_POINT('Ctrl Pts',(-3.51779937845998,2.18781686686112,4.7037286978635));
#18568=CARTESIAN_POINT('Ctrl Pts',(-3.73368595756569,2.21586230988758,4.6926149088067));
#18569=CARTESIAN_POINT('Ctrl Pts',(-3.82720826360965,2.41245106893735,4.6815011197499));
#18570=CARTESIAN_POINT('Ctrl Pts',(-3.71276426925474,2.59764322338409,4.67038733069309));
#18571=CARTESIAN_POINT('Ctrl Pts',(-3.49510586041716,2.60193029404067,4.65927354163629));
#18572=CARTESIAN_POINT('Ctrl Pts',(-3.37345824712023,2.42138827651674,4.64815975257948));
#18573=CARTESIAN_POINT('Ctrl Pts',(-3.4591668693923,2.22126932693707,4.63704596352268));
#18574=CARTESIAN_POINT('Ctrl Pts',(-3.67378165326609,2.18474458935644,4.62593217446588));
#18575=CARTESIAN_POINT('Ctrl Pts',(-3.82086325316422,2.34524557029854,4.61481838540907));
#18576=CARTESIAN_POINT('Ctrl Pts',(-3.7657862126822,2.55586390170729,4.60370459635227));
#18577=CARTESIAN_POINT('Ctrl Pts',(-3.55896317158719,2.6238182362596,4.59259080729546));
#18578=CARTESIAN_POINT('Ctrl Pts',(-3.38970160493063,2.48690920090586,4.58147701823866));
#18579=CARTESIAN_POINT('Ctrl Pts',(-3.41292854422122,2.27045118831796,4.57036322918185));
#18580=CARTESIAN_POINT('Ctrl Pts',(-3.60738410853246,2.17257067230145,4.55924944012505));
#18581=CARTESIAN_POINT('Ctrl Pts',(-3.79508091453898,2.28285879904056,4.54813565106825));
#18582=CARTESIAN_POINT('Ctrl Pts',(-3.80421794714692,2.50036759571139,4.53702186201144));
#18583=CARTESIAN_POINT('Ctrl Pts',(-3.62643197664818,2.62600879333718,4.52590807295464));
#18584=CARTESIAN_POINT('Ctrl Pts',(-3.42445251835268,2.54478158019733,4.51479428389783));
#18585=CARTESIAN_POINT('Ctrl Pts',(-3.38315366047576,2.3310341429862,4.50368049484103));
#18586=CARTESIAN_POINT('Ctrl Pts',(-3.54033671712511,2.18041194039358,4.49256670578422));
#18587=CARTESIAN_POINT('Ctrl Pts',(-3.75213025170582,2.23078117191311,4.48145291672742));
#18588=CARTESIAN_POINT('Ctrl Pts',(-3.82467724465257,2.43603833015588,4.47033912767062));
#18589=CARTESIAN_POINT('Ctrl Pts',(-3.69157460149519,2.60830916746569,4.45922533861381));
#18590=CARTESIAN_POINT('Ctrl Pts',(-3.47465269919707,2.58991231874976,4.44811154955701));
#18591=CARTESIAN_POINT('Ctrl Pts',(-3.37246257856274,2.39768645611616,4.4369977605002));
#18592=CARTESIAN_POINT('Ctrl Pts',(-3.47854008886701,2.20757843632347,4.4258839714434));
#18593=CARTESIAN_POINT('Ctrl Pts',(-3.69579113587624,2.19359559568096,4.41477018238659));
#18594=CARTESIAN_POINT('Ctrl Pts',(-3.82536366490058,2.36853796871893,4.4036563933298));
#18595=CARTESIAN_POINT('Ctrl Pts',(-3.74865788514769,2.57227605046896,4.39254260427298));
#18596=CARTESIAN_POINT('Ctrl Pts',(-3.5358846390969,2.61833160429067,4.38142881521619));
#18597=CARTESIAN_POINT('Ctrl Pts',(-3.38179534448736,2.46453836670119,4.37031502615938));
#18598=CARTESIAN_POINT('Ctrl Pts',(-3.4274343802517,2.25168724278053,4.35920123710257));
#18599=CARTESIAN_POINT('Ctrl Pts',(-3.63101840830467,2.17455880850134,4.34808744804577));
#18600=CARTESIAN_POINT('Ctrl Pts',(-3.80622350631146,2.30383864322893,4.33697365898897));
#18601=CARTESIAN_POINT('Ctrl Pts',(-3.79264467134891,2.52101708096281,4.32585986993216));
#18602=CARTESIAN_POINT('Ctrl Pts',(-3.60278716655164,2.62766630992157,4.31474608087536));
#18603=CARTESIAN_POINT('Ctrl Pts',(-3.41026840051456,2.5254403942132,4.30363229181855));
#18604=CARTESIAN_POINT('Ctrl Pts',(-3.3979620342723,2.38152235915268,4.29622309911402));
#18605=CARTESIAN_POINT('Ctrl Pts',(-3.42361008748734,2.32286851675082,4.29251850276175));
#18606=CARTESIAN_POINT('Ctrl Pts',(-3.44347998857283,2.53312198033322,5.22244449171475));
#18607=CARTESIAN_POINT('Ctrl Pts',(-3.39921376300775,2.48107535276698,5.21873989536248));
#18608=CARTESIAN_POINT('Ctrl Pts',(-3.36748900863419,2.33020914211697,5.21133070265795));
#18609=CARTESIAN_POINT('Ctrl Pts',(-3.53276736069978,2.16647689674201,5.20021691360114));
#18610=CARTESIAN_POINT('Ctrl Pts',(-3.75962266266454,2.21702523769905,5.18910312454434));
#18611=CARTESIAN_POINT('Ctrl Pts',(-3.84035223774737,2.43479235077285,5.17798933548753));
#18612=CARTESIAN_POINT('Ctrl Pts',(-3.70109553522054,2.62084298334156,5.16687554643073));
#18613=CARTESIAN_POINT('Ctrl Pts',(-3.46929950811782,2.60468896536386,5.15576175737392));
#18614=CARTESIAN_POINT('Ctrl Pts',(-3.35713783891219,2.401213058351,5.14464796831712));
#18615=CARTESIAN_POINT('Ctrl Pts',(-3.46726930372222,2.19661072251331,5.13353417926031));
#18616=CARTESIAN_POINT('Ctrl Pts',(-3.69889135748228,2.17818094124235,5.12242039020352));
#18617=CARTESIAN_POINT('Ctrl Pts',(-3.83999669192638,2.36278064343714,5.1113066011467));
#18618=CARTESIAN_POINT('Ctrl Pts',(-3.76143050146621,2.5814496508346,5.1001928120899));
#18619=CARTESIAN_POINT('Ctrl Pts',(-3.53510505788101,2.63403473315196,5.0890790230331));
#18620=CARTESIAN_POINT('Ctrl Pts',(-3.36817873292179,2.47240567046266,5.07796523397629));
#18621=CARTESIAN_POINT('Ctrl Pts',(-3.41344102170209,2.24450262655374,5.06685144491949));
#18622=CARTESIAN_POINT('Ctrl Pts',(-3.6294628695539,2.15892821683407,5.05573765586269));
#18623=CARTESIAN_POINT('Ctrl Pts',(-3.81851701352091,2.29400948184958,5.04462386680588));
#18624=CARTESIAN_POINT('Ctrl Pts',(-3.80756005948302,2.52610510127557,5.03351007774908));
#18625=CARTESIAN_POINT('Ctrl Pts',(-3.60662102779949,2.64277527582587,5.02239628869227));
#18626=CARTESIAN_POINT('Ctrl Pts',(-3.39962169493761,2.53723049491962,5.01128249963547));
#18627=CARTESIAN_POINT('Ctrl Pts',(-3.3760308968172,2.30607708183528,5.00016871057867));
#18628=CARTESIAN_POINT('Ctrl Pts',(-3.55744155898554,2.16089238284251,4.98905492152186));
#18629=CARTESIAN_POINT('Ctrl Pts',(-3.77780644477848,2.23456559653136,4.97794113246506));
#18630=CARTESIAN_POINT('Ctrl Pts',(-3.83542307524414,2.45966279635197,4.96682734340825));
#18631=CARTESIAN_POINT('Ctrl Pts',(-3.67755429503925,2.63014996180817,4.95571355435145));
#18632=CARTESIAN_POINT('Ctrl Pts',(-3.44869918906956,2.58997825726379,4.94459976529464));
#18633=CARTESIAN_POINT('Ctrl Pts',(-3.35833143120733,2.37591729928569,4.93348597623784));
#18634=CARTESIAN_POINT('Ctrl Pts',(-3.48916565507154,2.18389951041786,4.92237218718103));
#18635=CARTESIAN_POINT('Ctrl Pts',(-3.72144781179447,2.18968095039579,4.91125839812423));
#18636=CARTESIAN_POINT('Ctrl Pts',(-3.84256740907069,2.38796980166419,4.90014460906742));
#18637=CARTESIAN_POINT('Ctrl Pts',(-3.74166230592267,2.59727002989735,4.88903082001062));
#18638=CARTESIAN_POINT('Ctrl Pts',(-3.51109208760397,2.62600676257303,4.87791703095382));
#18639=CARTESIAN_POINT('Ctrl Pts',(-3.36190028978558,2.44787694237367,4.86680324189701));
#18640=CARTESIAN_POINT('Ctrl Pts',(-3.43064385696086,2.2259248138587,4.85568945284022));
#18641=CARTESIAN_POINT('Ctrl Pts',(-3.65440102248913,2.16330567736551,4.8445756637834));
#18642=CARTESIAN_POINT('Ctrl Pts',(-3.82836431518356,2.31733553867597,4.8334618747266));
#18643=CARTESIAN_POINT('Ctrl Pts',(-3.79330316036299,2.54702911891502,4.8223480856698));
#18644=CARTESIAN_POINT('Ctrl Pts',(-3.58130943065524,2.64214527918755,4.81123429661299));
#18645=CARTESIAN_POINT('Ctrl Pts',(-3.38642339103422,2.51562311930547,4.80012050755619));
#18646=CARTESIAN_POINT('Ctrl Pts',(-3.38702644372307,2.28326980706774,4.78900671849939));
#18647=CARTESIAN_POINT('Ctrl Pts',(-3.58256660775658,2.15776096423133,4.77789292944257));
#18648=CARTESIAN_POINT('Ctrl Pts',(-3.79406375341862,2.2539762580115,4.76677914038578));
#18649=CARTESIAN_POINT('Ctrl Pts',(-3.82793214474394,2.48384873885561,4.75566535132897));
#18650=CARTESIAN_POINT('Ctrl Pts',(-3.65317165905879,2.6369735181158,4.74455156227217));
#18651=CARTESIAN_POINT('Ctrl Pts',(-3.42974255082951,2.57319374878213,4.73343777321536));
#18652=CARTESIAN_POINT('Ctrl Pts',(-3.36215201667677,2.35088777703746,4.72232398415856));
#18653=CARTESIAN_POINT('Ctrl Pts',(-3.51226643903938,2.1735347799409,4.71121019510176));
#18654=CARTESIAN_POINT('Ctrl Pts',(-3.74268438471549,2.20346796705471,4.70009640604495));
#18655=CARTESIAN_POINT('Ctrl Pts',(-3.84250169491054,2.41328915274817,4.68898261698815));
#18656=CARTESIAN_POINT('Ctrl Pts',(-3.7203544535977,2.61094662622203,4.67786882793133));
#18657=CARTESIAN_POINT('Ctrl Pts',(-3.48804541599454,2.61552226041731,4.66675503887454));
#18658=CARTESIAN_POINT('Ctrl Pts',(-3.35820967878295,2.42282792546417,4.65564124981773));
#18659=CARTESIAN_POINT('Ctrl Pts',(-3.44968736466998,2.20923893144694,4.64452746076093));
#18660=CARTESIAN_POINT('Ctrl Pts',(-3.67874791033599,2.17025570685489,4.63341367170413));
#18661=CARTESIAN_POINT('Ctrl Pts',(-3.83572960060904,2.34156003925422,4.62229988264732));
#18662=CARTESIAN_POINT('Ctrl Pts',(-3.77694531408991,2.56635513048207,4.61118609359051));
#18663=CARTESIAN_POINT('Ctrl Pts',(-3.55620097488638,2.63888348417682,4.60007230453371));
#18664=CARTESIAN_POINT('Ctrl Pts',(-3.3755463800872,2.4927590756963,4.58895851547691));
#18665=CARTESIAN_POINT('Ctrl Pts',(-3.40033672906513,2.26173123324197,4.5778447264201));
#18666=CARTESIAN_POINT('Ctrl Pts',(-3.60788113427776,2.15726236113484,4.5667309373633));
#18667=CARTESIAN_POINT('Ctrl Pts',(-3.80821184788277,2.27497400259471,4.55561714830649));
#18668=CARTESIAN_POINT('Ctrl Pts',(-3.81796389588787,2.50712335760782,4.54450335924969));
#18669=CARTESIAN_POINT('Ctrl Pts',(-3.62821111800771,2.64122148806661,4.53338957019289));
#18670=CARTESIAN_POINT('Ctrl Pts',(-3.41263638408026,2.55452685581013,4.52227578113608));
#18671=CARTESIAN_POINT('Ctrl Pts',(-3.36855769224962,2.32639203807509,4.51116199207928));
#18672=CARTESIAN_POINT('Ctrl Pts',(-3.536320770243,2.1656314264689,4.50004820302247));
#18673=CARTESIAN_POINT('Ctrl Pts',(-3.76237016779111,2.21939102051171,4.48893441396567));
#18674=CARTESIAN_POINT('Ctrl Pts',(-3.83980031258758,2.43846407699132,4.47782062490887));
#18675=CARTESIAN_POINT('Ctrl Pts',(-3.69773850528383,2.62233049702197,4.46670683585206));
#18676=CARTESIAN_POINT('Ctrl Pts',(-3.46621554861493,2.60269535293104,4.45559304679526));
#18677=CARTESIAN_POINT('Ctrl Pts',(-3.35714699158608,2.39753073103871,4.44447925773845));
#18678=CARTESIAN_POINT('Ctrl Pts',(-3.47036459922058,2.19462650439043,4.43336546868165));
#18679=CARTESIAN_POINT('Ctrl Pts',(-3.70223885539349,2.17970247609322,4.42225167962484));
#18680=CARTESIAN_POINT('Ctrl Pts',(-3.84053293591263,2.36642025342839,4.41113789056805));
#18681=CARTESIAN_POINT('Ctrl Pts',(-3.75866407558161,2.58387198408852,4.40002410151123));
#18682=CARTESIAN_POINT('Ctrl Pts',(-3.53156902199863,2.63302754596983,4.38891031245443));
#18683=CARTESIAN_POINT('Ctrl Pts',(-3.36710794775451,2.46888245639993,4.37779652339763));
#18684=CARTESIAN_POINT('Ctrl Pts',(-3.41581895566904,2.24170428297288,4.36668273434082));
#18685=CARTESIAN_POINT('Ctrl Pts',(-3.63310626324856,2.15938431915927,4.35556894528402));
#18686=CARTESIAN_POINT('Ctrl Pts',(-3.82010444962002,2.29736600407305,4.34445515622722));
#18687=CARTESIAN_POINT('Ctrl Pts',(-3.80561162070166,2.52916276362653,4.33334136717041));
#18688=CARTESIAN_POINT('Ctrl Pts',(-3.60297477126067,2.64299057240655,4.32222757811361));
#18689=CARTESIAN_POINT('Ctrl Pts',(-3.39749753058122,2.53388381093044,4.3111137890568));
#18690=CARTESIAN_POINT('Ctrl Pts',(-3.38436282049399,2.380278625644,4.30370459635227));
#18691=CARTESIAN_POINT('Ctrl Pts',(-3.41173724903364,2.31767678198965,4.3));
#18692=CARTESIAN_POINT('Ctrl Pts',(-3.47309291201476,2.50793586530485,5.2));
#18693=CARTESIAN_POINT('Ctrl Pts',(-3.46488109712516,2.50027511355887,5.2));
#18694=CARTESIAN_POINT('Ctrl Pts',(-3.45756392397337,2.49177395403935,5.2));
#18695=CARTESIAN_POINT('Ctrl Pts',(-3.45114582175476,2.48262659215394,5.2));
#18696=CARTESIAN_POINT('Ctrl Pts',(-3.44637505636198,2.47582708724863,5.2));
#18697=CARTESIAN_POINT('Ctrl Pts',(-3.44210140258396,2.46866923691254,5.2));
#18698=CARTESIAN_POINT('Ctrl Pts',(-3.4383368615674,2.46121837901648,5.2));
#18699=CARTESIAN_POINT('Ctrl Pts',(-3.43611956164057,2.45682985287343,5.2));
#18700=CARTESIAN_POINT('Ctrl Pts',(-3.43407749071882,2.45233446363919,5.2));
#18701=CARTESIAN_POINT('Ctrl Pts',(-3.4322255599542,2.44777399682775,5.2));
#18702=CARTESIAN_POINT('Ctrl Pts',(-3.42766722424942,2.43654888026604,5.2));
#18703=CARTESIAN_POINT('Ctrl Pts',(-3.42424189960471,2.42490562017205,5.2));
#18704=CARTESIAN_POINT('Ctrl Pts',(-3.42197767565222,2.41304271238881,5.2));
#18705=CARTESIAN_POINT('Ctrl Pts',(-3.42053879301361,2.40550400048974,5.2));
#18706=CARTESIAN_POINT('Ctrl Pts',(-3.41956954249672,2.39787570455109,5.2));
#18707=CARTESIAN_POINT('Ctrl Pts',(-3.41908669765048,2.39020364672881,5.2));
#18708=CARTESIAN_POINT('Ctrl Pts',(-3.4188613702662,2.3866233564252,5.2));
#18709=CARTESIAN_POINT('Ctrl Pts',(-3.4187425132976,2.38303698501937,5.2));
#18710=CARTESIAN_POINT('Ctrl Pts',(-3.4187312729093,2.37945933257344,5.2));
#18711=CARTESIAN_POINT('Ctrl Pts',(-3.41869622423253,2.36830384747272,5.2));
#18712=CARTESIAN_POINT('Ctrl Pts',(-3.4197031160267,2.35720597826242,5.2));
#18713=CARTESIAN_POINT('Ctrl Pts',(-3.42178566785009,2.34630687436894,5.2));
#18714=CARTESIAN_POINT('Ctrl Pts',(-3.42294604955552,2.3402339783087,5.2));
#18715=CARTESIAN_POINT('Ctrl Pts',(-3.42444092603953,2.33422255306027,5.2));
#18716=CARTESIAN_POINT('Ctrl Pts',(-3.42625156753842,2.32828873958556,5.2));
#18717=CARTESIAN_POINT('Ctrl Pts',(-3.42738421175614,2.32457685099508,5.2));
#18718=CARTESIAN_POINT('Ctrl Pts',(-3.42864107094821,2.32089381471682,5.2));
#18719=CARTESIAN_POINT('Ctrl Pts',(-3.4300164442918,2.31724844575858,5.2));
#18720=CARTESIAN_POINT('Ctrl Pts',(-3.43439823178552,2.30563470307137,5.2));
#18721=CARTESIAN_POINT('Ctrl Pts',(-3.43994733372525,2.29448387749046,5.2));
#18722=CARTESIAN_POINT('Ctrl Pts',(-3.44649833143843,2.28391851131164,5.2));
#18723=CARTESIAN_POINT('Ctrl Pts',(-3.45083930540137,2.27691744345919,5.2));
#18724=CARTESIAN_POINT('Ctrl Pts',(-3.45562139981211,2.27017330264703,5.2));
#18725=CARTESIAN_POINT('Ctrl Pts',(-3.46080803162185,2.26372396193311,5.2));
#18726=CARTESIAN_POINT('Ctrl Pts',(-3.46351816065219,2.2603540397685,5.2));
#18727=CARTESIAN_POINT('Ctrl Pts',(-3.46634013864158,2.25706328802701,5.2));
#18728=CARTESIAN_POINT('Ctrl Pts',(-3.46926558695491,2.25386191331523,5.2));
#18729=CARTESIAN_POINT('Ctrl Pts',(-3.47553201369268,2.24700444124844,5.2));
#18730=CARTESIAN_POINT('Ctrl Pts',(-3.48224798017073,2.24058272300471,5.2));
#18731=CARTESIAN_POINT('Ctrl Pts',(-3.48935940275436,2.23464751188384,5.2));
#18732=CARTESIAN_POINT('Ctrl Pts',(-3.49388585721574,2.23086972163985,5.2));
#18733=CARTESIAN_POINT('Ctrl Pts',(-3.49857277644925,2.2272891074735,5.2));
#18734=CARTESIAN_POINT('Ctrl Pts',(-3.50340840926684,2.2239201748241,5.2));
#18735=CARTESIAN_POINT('Ctrl Pts',(-3.50748096973522,2.22108286635877,5.2));
#18736=CARTESIAN_POINT('Ctrl Pts',(-3.51165201299164,2.21840074277452,5.2));
#18737=CARTESIAN_POINT('Ctrl Pts',(-3.51591072169151,2.21588342574414,5.2));
#18738=CARTESIAN_POINT('Ctrl Pts',(-3.52463381704441,2.21072721571968,5.2));
#18739=CARTESIAN_POINT('Ctrl Pts',(-3.53372795060187,2.20625881994954,5.2));
#18740=CARTESIAN_POINT('Ctrl Pts',(-3.54313435341931,2.20255201733462,5.2));
#18741=CARTESIAN_POINT('Ctrl Pts',(-3.5443736619696,2.20206364018726,5.2));
#18742=CARTESIAN_POINT('Ctrl Pts',(-3.54561840623672,2.20158850319392,5.2));
#18743=CARTESIAN_POINT('Ctrl Pts',(-3.54686839490754,2.2011265482535,5.2));
#18744=CARTESIAN_POINT('Ctrl Pts',(-3.76673280722786,2.39986996770474,5.08714803633902));
#18745=CARTESIAN_POINT('Ctrl Pts',(-3.76680595967625,2.39134538779314,5.08771939403666));
#18746=CARTESIAN_POINT('Ctrl Pts',(-3.76620865205667,2.38283109327188,5.08829075173431));
#18747=CARTESIAN_POINT('Ctrl Pts',(-3.76490523356496,2.37442631092714,5.08886210943196));
#18748=CARTESIAN_POINT('Ctrl Pts',(-3.75645406644185,2.31993098139145,5.09256670578422));
#18749=CARTESIAN_POINT('Ctrl Pts',(-3.71831779890178,2.27003957467425,5.0962713021365));
#18750=CARTESIAN_POINT('Ctrl Pts',(-3.66794964148213,2.24758436209697,5.09997589848877));
#18751=CARTESIAN_POINT('Ctrl Pts',(-3.61758148406248,2.22512914951968,5.10368049484103));
#18752=CARTESIAN_POINT('Ctrl Pts',(-3.55498143676326,2.2301101310823,5.1073850911933));
#18753=CARTESIAN_POINT('Ctrl Pts',(-3.50879890345119,2.26024936189732,5.11108968754557));
#18754=CARTESIAN_POINT('Ctrl Pts',(-3.46261637013913,2.29038859271235,5.11479428389783));
#18755=CARTESIAN_POINT('Ctrl Pts',(-3.43285135081423,2.34568607277977,5.1184988802501));
#18756=CARTESIAN_POINT('Ctrl Pts',(-3.43312570053424,2.40083133397043,5.12220347660237));
#18757=CARTESIAN_POINT('Ctrl Pts',(-3.43340005025424,2.45597659516109,5.12590807295464));
#18758=CARTESIAN_POINT('Ctrl Pts',(-3.46371376901915,2.51096963747498,5.12961266930691));
#18759=CARTESIAN_POINT('Ctrl Pts',(-3.51019416177169,2.54064911632758,5.13331726565918));
#18760=CARTESIAN_POINT('Ctrl Pts',(-3.55667455452423,2.57032859518018,5.13702186201145));
#18761=CARTESIAN_POINT('Ctrl Pts',(-3.61932162126441,2.57469451057149,5.14072645836371));
#18762=CARTESIAN_POINT('Ctrl Pts',(-3.6694634753069,2.55173569482678,5.14443105471598));
#18763=CARTESIAN_POINT('Ctrl Pts',(-3.71960532934939,2.52877687908207,5.14813565106825));
#18764=CARTESIAN_POINT('Ctrl Pts',(-3.75724197069419,2.47849333220135,5.15184024742052));
#18765=CARTESIAN_POINT('Ctrl Pts',(-3.76515097781766,2.42392380920663,5.15554484377278));
#18766=CARTESIAN_POINT('Ctrl Pts',(-3.76629187237323,2.41605201560311,5.15607924129486));
#18767=CARTESIAN_POINT('Ctrl Pts',(-3.76681417046854,2.40809103597041,5.15661363881694));
#18768=CARTESIAN_POINT('Ctrl Pts',(-3.76674783252531,2.40012156540224,5.15714803633902));
#18769=CARTESIAN_POINT('Ctrl Pts',(-3.65301702171886,2.20148256743283,5.2));
#18770=CARTESIAN_POINT('Ctrl Pts',(-3.71902879097456,2.21911198848201,5.19629540364773));
#18771=CARTESIAN_POINT('Ctrl Pts',(-3.83093279751213,2.32515241961692,5.1888862109432));
#18772=CARTESIAN_POINT('Ctrl Pts',(-3.78812294461068,2.55382789975093,5.17777242188639));
#18773=CARTESIAN_POINT('Ctrl Pts',(-3.57278676575927,2.64128531597693,5.16665863282959));
#18774=CARTESIAN_POINT('Ctrl Pts',(-3.38252462806861,2.5080933346037,5.15554484377278));
#18775=CARTESIAN_POINT('Ctrl Pts',(-3.39123766596766,2.27586209704876,5.14443105471597));
#18776=CARTESIAN_POINT('Ctrl Pts',(-3.59107442724388,2.15730569128375,5.13331726565918));
#18777=CARTESIAN_POINT('Ctrl Pts',(-3.79906029518588,2.2608651698129,5.12220347660237));
#18778=CARTESIAN_POINT('Ctrl Pts',(-3.82485429121136,2.49178880612566,5.11108968754556));
#18779=CARTESIAN_POINT('Ctrl Pts',(-3.64483147349944,2.63869087951471,5.09997589848877));
#18780=CARTESIAN_POINT('Ctrl Pts',(-3.42377646220466,2.56711959422357,5.08886210943196));
#18781=CARTESIAN_POINT('Ctrl Pts',(-3.36401957377094,2.34258029572384,5.07774832037515));
#18782=CARTESIAN_POINT('Ctrl Pts',(-3.52025888482579,2.17059867951396,5.06663453131835));
#18783=CARTESIAN_POINT('Ctrl Pts',(-3.74948582371233,2.20859030608788,5.05552074226155));
#18784=CARTESIAN_POINT('Ctrl Pts',(-3.8418868522934,2.42178158973285,5.04440695320474));
#18785=CARTESIAN_POINT('Ctrl Pts',(-3.71288602216703,2.61503584063672,5.03329316414794));
#18786=CARTESIAN_POINT('Ctrl Pts',(-3.48055937550073,2.61146539619723,5.02217937509113));
#18787=CARTESIAN_POINT('Ctrl Pts',(-3.35755806712823,2.4143382523336,5.01106558603433));
#18788=CARTESIAN_POINT('Ctrl Pts',(-3.45646661930996,2.20408715554039,4.99995179697752));
#18789=CARTESIAN_POINT('Ctrl Pts',(-3.68675289766315,2.17315730107164,4.98883800792072));
#18790=CARTESIAN_POINT('Ctrl Pts',(-3.83763326741432,2.34985914450584,4.97772421886391));
#18791=CARTESIAN_POINT('Ctrl Pts',(-3.77100521132112,2.57245548011022,4.96661042980712));
#18792=CARTESIAN_POINT('Ctrl Pts',(-3.54785414659174,2.63720135974049,4.9554966407503));
#18793=CARTESIAN_POINT('Ctrl Pts',(-3.37243277255298,2.48483414437987,4.94438285169351));
#18794=CARTESIAN_POINT('Ctrl Pts',(-3.40530626273826,2.25481727477052,4.9332690626367));
#18795=CARTESIAN_POINT('Ctrl Pts',(-3.61638513853951,2.15768779995451,4.9221552735799));
#18796=CARTESIAN_POINT('Ctrl Pts',(-3.81246651125382,2.28234942989398,4.91104148452309));
#18797=CARTESIAN_POINT('Ctrl Pts',(-3.81407487666422,2.51469796087643,4.89992769546629));
#18798=CARTESIAN_POINT('Ctrl Pts',(-3.6197380796992,2.64206214751696,4.88881390640948));
#18799=CARTESIAN_POINT('Ctrl Pts',(-3.40733479453568,2.54786410535795,4.87770011735268));
#18800=CARTESIAN_POINT('Ctrl Pts',(-3.37128015690807,2.3183243706747,4.86658632829587));
#18801=CARTESIAN_POINT('Ctrl Pts',(-3.54457538552076,2.16354326577609,4.85547253923908));
#18802=CARTESIAN_POINT('Ctrl Pts',(-3.76860139232476,2.2251936913151,4.84435875018226));
#18803=CARTESIAN_POINT('Ctrl Pts',(-3.83830463266378,2.44684631363142,4.83324496112547));
#18804=CARTESIAN_POINT('Ctrl Pts',(-3.68988494016744,2.62561997380774,4.82213117206865));
#18805=CARTESIAN_POINT('Ctrl Pts',(-3.45919254257122,2.59788111325323,4.81101738301186));
#18806=CARTESIAN_POINT('Ctrl Pts',(-3.35738280762477,2.38901942561361,4.79990359395505));
#18807=CARTESIAN_POINT('Ctrl Pts',(-3.47764334032546,2.19020838223802,4.78878980489825));
#18808=CARTESIAN_POINT('Ctrl Pts',(-3.70989831124516,2.18342198579874,4.77767601584144));
#18809=CARTESIAN_POINT('Ctrl Pts',(-3.84156211155055,2.3748719019196,4.76656222678464));
#18810=CARTESIAN_POINT('Ctrl Pts',(-3.75212137165305,2.58932185118547,4.75544843772783));
#18811=CARTESIAN_POINT('Ctrl Pts',(-3.52344221510783,2.63048336300545,4.74433464867103));
#18812=CARTESIAN_POINT('Ctrl Pts',(-3.36483726729874,2.46068083880743,4.73322085961422));
#18813=CARTESIAN_POINT('Ctrl Pts',(-3.42147943565789,2.23533645468145,4.72210707055742));
#18814=CARTESIAN_POINT('Ctrl Pts',(-3.64152350112028,2.16071048099716,4.71099328150062));
#18815=CARTESIAN_POINT('Ctrl Pts',(-3.82356063509873,2.30510891778388,4.69987949244381));
#18816=CARTESIAN_POINT('Ctrl Pts',(-3.80097018442129,2.53636223826109,4.68876570338701));
#18817=CARTESIAN_POINT('Ctrl Pts',(-3.59442944478611,2.64280165560495,4.6776519143302));
#18818=CARTESIAN_POINT('Ctrl Pts',(-3.39298749751263,2.52700196401557,4.6665381252734));
#18819=CARTESIAN_POINT('Ctrl Pts',(-3.38102644144724,2.29495593446246,4.65542433621659));
#18820=CARTESIAN_POINT('Ctrl Pts',(-3.56949436685434,2.15905792937668,4.64431054715979));
#18821=CARTESIAN_POINT('Ctrl Pts',(-3.7858844442369,2.24369693400118,4.63319675810299));
#18822=CARTESIAN_POINT('Ctrl Pts',(-3.83213238173679,2.47140190753206,4.62208296904618));
#18823=CARTESIAN_POINT('Ctrl Pts',(-3.66590691767206,2.63375190534549,4.61096917998937));
#18824=CARTESIAN_POINT('Ctrl Pts',(-3.43935610442817,2.58214613327058,4.59985539093257));
#18825=CARTESIAN_POINT('Ctrl Pts',(-3.35984447062414,2.36381993973287,4.58874160187577));
#18826=CARTESIAN_POINT('Ctrl Pts',(-3.50014991641224,2.17860976567263,4.57762781281897));
#18827=CARTESIAN_POINT('Ctrl Pts',(-3.73184927607424,2.1960405838179,4.56651402376216));
#18828=CARTESIAN_POINT('Ctrl Pts',(-3.84286549809491,2.40015776867247,4.55540023470536));
#18829=CARTESIAN_POINT('Ctrl Pts',(-3.73158417538336,2.60413054603043,4.54428644564855));
#18830=CARTESIAN_POINT('Ctrl Pts',(-3.49986236476522,2.62126031969194,4.53317265659175));
#18831=CARTESIAN_POINT('Ctrl Pts',(-3.35979766713961,2.43586801331045,4.52205886753494));
#18832=CARTESIAN_POINT('Ctrl Pts',(-3.43959288921302,2.2176453079079,4.51094507847814));
#18833=CARTESIAN_POINT('Ctrl Pts',(-3.66621055822496,2.16633391955349,4.49983128942134));
#18834=CARTESIAN_POINT('Ctrl Pts',(-3.83222495382674,2.32889974592014,4.48871750036453));
#18835=CARTESIAN_POINT('Ctrl Pts',(-3.78568121275365,2.55654443850517,4.47760371130773));
#18836=CARTESIAN_POINT('Ctrl Pts',(-3.56918135753979,2.64090223654315,4.46648992225092));
#18837=CARTESIAN_POINT('Ctrl Pts',(-3.38089014394226,2.50475947474088,4.45537613319412));
#18838=CARTESIAN_POINT('Ctrl Pts',(-3.3931526891646,2.27272919910994,4.44426234413731));
#18839=CARTESIAN_POINT('Ctrl Pts',(-3.59474487835949,2.15719128792351,4.43314855508051));
#18840=CARTESIAN_POINT('Ctrl Pts',(-3.80114723098,2.26389903055612,4.4220347660237));
#18841=CARTESIAN_POINT('Ctrl Pts',(-3.82343705972838,2.49518136177793,4.4109209769669));
#18842=CARTESIAN_POINT('Ctrl Pts',(-3.64121277856108,2.63934345799643,4.3998071879101));
#18843=CARTESIAN_POINT('Ctrl Pts',(-3.4212652433475,2.56443108225311,4.38869339885329));
#18844=CARTESIAN_POINT('Ctrl Pts',(-3.36491712045917,2.33901445477475,4.3775796097965));
#18845=CARTESIAN_POINT('Ctrl Pts',(-3.52374009472539,2.16941582002738,4.36646582073968));
#18846=CARTESIAN_POINT('Ctrl Pts',(-3.75237048890211,2.21087904346051,4.35535203168288));
#18847=CARTESIAN_POINT('Ctrl Pts',(-3.84152270551859,2.42543572391857,4.34423824262608));
#18848=CARTESIAN_POINT('Ctrl Pts',(-3.70962996035205,2.61673302206395,4.33312445356927));
#18849=CARTESIAN_POINT('Ctrl Pts',(-3.47734458963256,2.60960762555316,4.32201066451247));
#18850=CARTESIAN_POINT('Ctrl Pts',(-3.35742145615876,2.41071512444121,4.31089687545567));
#18851=CARTESIAN_POINT('Ctrl Pts',(-3.45934316515028,2.20183612882053,4.29978308639885));
#18852=CARTESIAN_POINT('Ctrl Pts',(-3.69040350703126,2.17470170179864,4.28866929734206));
#18853=CARTESIAN_POINT('Ctrl Pts',(-3.7885754343637,2.29356865430552,4.28126010463752));
#18854=CARTESIAN_POINT('Ctrl Pts',(-3.80166758614466,2.36062792457102,4.27755550828525));
#18855=CARTESIAN_POINT('Ctrl Pts',(-3.64967348970877,2.21400211999972,5.20748149723825));
#18856=CARTESIAN_POINT('Ctrl Pts',(-3.71152220988337,2.2305197371096,5.20377690088598));
#18857=CARTESIAN_POINT('Ctrl Pts',(-3.81636896167925,2.32987270138258,5.19636770818145));
#18858=CARTESIAN_POINT('Ctrl Pts',(-3.7762589230805,2.54412670398045,5.18525391912464));
#18859=CARTESIAN_POINT('Ctrl Pts',(-3.57450297532427,2.62606859592404,5.17414013006784));
#18860=CARTESIAN_POINT('Ctrl Pts',(-3.39623976792153,2.50127640086039,5.16302634101103));
#18861=CARTESIAN_POINT('Ctrl Pts',(-3.404403315861,2.28369088559113,5.15191255195423));
#18862=CARTESIAN_POINT('Ctrl Pts',(-3.59163732076848,2.17261126982347,5.14079876289742));
#18863=CARTESIAN_POINT('Ctrl Pts',(-3.78650650684933,2.26963974340016,5.12968497384063));
#18864=CARTESIAN_POINT('Ctrl Pts',(-3.8106737979302,2.48600012163341,5.11857118478381));
#18865=CARTESIAN_POINT('Ctrl Pts',(-3.64200416517759,2.62363777825967,5.10745739572702));
#18866=CARTESIAN_POINT('Ctrl Pts',(-3.43489004460608,2.55658015434777,5.0963436066702));
#18867=CARTESIAN_POINT('Ctrl Pts',(-3.37890173959752,2.34620148403342,5.0852298176134));
#18868=CARTESIAN_POINT('Ctrl Pts',(-3.52528777861237,2.18506593235721,5.0741160285566));
#18869=CARTESIAN_POINT('Ctrl Pts',(-3.74005846207577,2.22066160730187,5.06300223949979));
#18870=CARTESIAN_POINT('Ctrl Pts',(-3.82663219619914,2.42040792821545,5.05188845044299));
#18871=CARTESIAN_POINT('Ctrl Pts',(-3.70576683635895,2.60147455044772,5.04077466138619));
#18872=CARTESIAN_POINT('Ctrl Pts',(-3.4880919289783,2.59812927699836,5.02966087232938));
#18873=CARTESIAN_POINT('Ctrl Pts',(-3.37284772952088,2.41343400678959,5.01854708327258));
#18874=CARTESIAN_POINT('Ctrl Pts',(-3.46551858860765,2.21644244909332,5.00743329421577));
#18875=CARTESIAN_POINT('Ctrl Pts',(-3.68128180402377,2.18746319379313,4.99631950515897));
#18876=CARTESIAN_POINT('Ctrl Pts',(-3.82264686473641,2.35302129035867,4.98520571610216));
#18877=CARTESIAN_POINT('Ctrl Pts',(-3.76022072401106,2.56157953122871,4.97409192704537));
#18878=CARTESIAN_POINT('Ctrl Pts',(-3.55114273814991,2.6222421954303,4.96297813798855));
#18879=CARTESIAN_POINT('Ctrl Pts',(-3.38678435785046,2.47948405740616,4.95186434893176));
#18880=CARTESIAN_POINT('Ctrl Pts',(-3.41758467298453,2.26397326040267,4.94075055987495));
#18881=CARTESIAN_POINT('Ctrl Pts',(-3.61535180559434,2.17296928071335,4.92963677081814));
#18882=CARTESIAN_POINT('Ctrl Pts',(-3.79906725647832,2.28976909313423,4.91852298176134));
#18883=CARTESIAN_POINT('Ctrl Pts',(-3.80057418991348,2.50746450469106,4.90740919270453));
#18884=CARTESIAN_POINT('Ctrl Pts',(-3.61849329266379,2.62679643638467,4.89629540364773));
#18885=CARTESIAN_POINT('Ctrl Pts',(-3.41948527490624,2.53853901780343,4.88518161459093));
#18886=CARTESIAN_POINT('Ctrl Pts',(-3.38570443220547,2.32347526509011,4.87406782553412));
#18887=CARTESIAN_POINT('Ctrl Pts',(-3.54807075298295,2.17845547008797,4.86295403647732));
#18888=CARTESIAN_POINT('Ctrl Pts',(-3.7579685024734,2.23621789580084,4.85184024742051));
#18889=CARTESIAN_POINT('Ctrl Pts',(-3.82327589016501,2.44389193890226,4.84072645836371));
#18890=CARTESIAN_POINT('Ctrl Pts',(-3.6842163234679,2.61139119255816,4.8296126693069));
#18891=CARTESIAN_POINT('Ctrl Pts',(-3.4680726008225,2.58540169032632,4.8184988802501));
#18892=CARTESIAN_POINT('Ctrl Pts',(-3.37268352280275,2.38971191834066,4.8073850911933));
#18893=CARTESIAN_POINT('Ctrl Pts',(-3.48535979430583,2.20343894417256,4.79627130213649));
#18894=CARTESIAN_POINT('Ctrl Pts',(-3.70296754618914,2.19708053355731,4.78515751307969));
#18895=CARTESIAN_POINT('Ctrl Pts',(-3.82632793531414,2.37645661184032,4.77404372402288));
#18896=CARTESIAN_POINT('Ctrl Pts',(-3.74252779851275,2.57738222030606,4.76292993496608));
#18897=CARTESIAN_POINT('Ctrl Pts',(-3.52827035135747,2.61594787087447,4.75181614590928));
#18898=CARTESIAN_POINT('Ctrl Pts',(-3.37966786507423,2.45685398621605,4.74070235685247));
#18899=CARTESIAN_POINT('Ctrl Pts',(-3.43273788062492,2.24572100320602,4.72958856779567));
#18900=CARTESIAN_POINT('Ctrl Pts',(-3.63890481092106,2.17580133560435,4.71847477873887));
#18901=CARTESIAN_POINT('Ctrl Pts',(-3.80946172657059,2.31109324810979,4.70736098968206));
#18902=CARTESIAN_POINT('Ctrl Pts',(-3.78829594843252,2.5277625188915,4.69624720062526));
#18903=CARTESIAN_POINT('Ctrl Pts',(-3.59478075327286,2.62748930720629,4.68513341156845));
#18904=CARTESIAN_POINT('Ctrl Pts',(-3.40604279383286,2.51899255273097,4.67401962251165));
#18905=CARTESIAN_POINT('Ctrl Pts',(-3.39483606482192,2.30158056527362,4.66290583345485));
#18906=CARTESIAN_POINT('Ctrl Pts',(-3.57141821239684,2.17425300257371,4.65179204439804));
#18907=CARTESIAN_POINT('Ctrl Pts',(-3.77416159430429,2.253554226763,4.64067825534124));
#18908=CARTESIAN_POINT('Ctrl Pts',(-3.81749289381852,2.46689892800445,4.62956446628442));
#18909=CARTESIAN_POINT('Ctrl Pts',(-3.66175048108285,2.61901028175737,4.61845067722763));
#18910=CARTESIAN_POINT('Ctrl Pts',(-3.44948715271524,2.57065904087346,4.60733688817082));
#18911=CARTESIAN_POINT('Ctrl Pts',(-3.37498994039659,2.36610164447049,4.59622309911403));
#18912=CARTESIAN_POINT('Ctrl Pts',(-3.50644698742571,2.19257179732202,4.58510931005721));
#18913=CARTESIAN_POINT('Ctrl Pts',(-3.72353416781713,2.20890333647083,4.57399552100042));
#18914=CARTESIAN_POINT('Ctrl Pts',(-3.82754912345333,2.40014781895086,4.5628817319436));
#18915=CARTESIAN_POINT('Ctrl Pts',(-3.723285785769,2.59125700102993,4.55176794288681));
#18916=CARTESIAN_POINT('Ctrl Pts',(-3.50617757029671,2.60730648114219,4.54065415382999));
#18917=CARTESIAN_POINT('Ctrl Pts',(-3.37494608858577,2.43360598789383,4.52954036477319));
#18918=CARTESIAN_POINT('Ctrl Pts',(-3.44970900460718,2.22914555312034,4.51842657571639));
#18919=CARTESIAN_POINT('Ctrl Pts',(-3.66203497246676,2.18107013057245,4.50731278665959));
#18920=CARTESIAN_POINT('Ctrl Pts',(-3.81757962782599,2.33338370159577,4.49619899760278));
#18921=CARTESIAN_POINT('Ctrl Pts',(-3.77397117966642,2.54667192352462,4.48508520854598));
#18922=CARTESIAN_POINT('Ctrl Pts',(-3.57112494309463,2.62570967549255,4.47397141948917));
#18923=CARTESIAN_POINT('Ctrl Pts',(-3.3947083629539,2.49815279172096,4.46285763043237));
#18924=CARTESIAN_POINT('Ctrl Pts',(-3.40619756763113,2.28075556466066,4.45174384137556));
#18925=CARTESIAN_POINT('Ctrl Pts',(-3.59507629394739,2.17250408134035,4.44063005231876));
#18926=CARTESIAN_POINT('Ctrl Pts',(-3.78846182950481,2.27248227294105,4.42951626326195));
#18927=CARTESIAN_POINT('Ctrl Pts',(-3.80934594451251,2.48917872489734,4.41840247420516));
#18928=CARTESIAN_POINT('Ctrl Pts',(-3.63861368415939,2.62424920171285,4.40728868514834));
#18929=CARTESIAN_POINT('Ctrl Pts',(-3.43253719640727,2.55406119407111,4.39617489609155));
#18930=CARTESIAN_POINT('Ctrl Pts',(-3.37974268227471,2.34286052375416,4.38506110703474));
#18931=CARTESIAN_POINT('Ctrl Pts',(-3.5285494451209,2.18395767020613,4.37394731797793));
#18932=CARTESIAN_POINT('Ctrl Pts',(-3.74276120511889,2.22280600486777,4.36283352892113));
#18933=CARTESIAN_POINT('Ctrl Pts',(-3.82629101443365,2.42383161349583,4.35171973986432));
#18934=CARTESIAN_POINT('Ctrl Pts',(-3.70271611891361,2.60306469869495,4.34060595080752));
#18935=CARTESIAN_POINT('Ctrl Pts',(-3.48507988440164,2.59638866713425,4.32949216175072));
#18936=CARTESIAN_POINT('Ctrl Pts',(-3.37271973395708,2.41003937238272,4.31837837269391));
#18937=CARTESIAN_POINT('Ctrl Pts',(-3.46821372435015,2.21433338394825,4.30726458363711));
#18938=CARTESIAN_POINT('Ctrl Pts',(-3.68470218678007,2.18891019649399,4.2961507945803));
#18939=CARTESIAN_POINT('Ctrl Pts',(-3.77668287645173,2.30028077429396,4.28874160187577));
#18940=CARTESIAN_POINT('Ctrl Pts',(-3.78894936833816,2.36311093455975,4.2850370055235));
#18941=CARTESIAN_POINT('Ctrl Pts',(-3.64632995769868,2.22652167256662,5.2149629944765));
#18942=CARTESIAN_POINT('Ctrl Pts',(-3.70401562879218,2.24192748573719,5.21125839812423));
#18943=CARTESIAN_POINT('Ctrl Pts',(-3.80180512584637,2.33459298314823,5.2038492054197));
#18944=CARTESIAN_POINT('Ctrl Pts',(-3.76439490155032,2.53442550820997,5.19273541636289));
#18945=CARTESIAN_POINT('Ctrl Pts',(-3.57621918488928,2.61085187587115,5.18162162730609));
#18946=CARTESIAN_POINT('Ctrl Pts',(-3.40995490777444,2.49445946711708,5.17050783824928));
#18947=CARTESIAN_POINT('Ctrl Pts',(-3.41756896575436,2.2915196741335,5.15939404919248));
#18948=CARTESIAN_POINT('Ctrl Pts',(-3.59220021429306,2.18791684836318,5.14828026013568));
#18949=CARTESIAN_POINT('Ctrl Pts',(-3.7739527185128,2.27841431698741,5.13716647107887));
#18950=CARTESIAN_POINT('Ctrl Pts',(-3.79649330464903,2.48021143714115,5.12605268202206));
#18951=CARTESIAN_POINT('Ctrl Pts',(-3.63917685685576,2.60858467700464,5.11493889296527));
#18952=CARTESIAN_POINT('Ctrl Pts',(-3.44600362700749,2.54604071447196,5.10382510390845));
#18953=CARTESIAN_POINT('Ctrl Pts',(-3.39378390542411,2.349822672343,5.09271131485166));
#18954=CARTESIAN_POINT('Ctrl Pts',(-3.53031667239896,2.19953318520045,5.08159752579485));
#18955=CARTESIAN_POINT('Ctrl Pts',(-3.73063110043921,2.23273290851586,5.07048373673805));
#18956=CARTESIAN_POINT('Ctrl Pts',(-3.81137754010487,2.41903426669804,5.05936994768123));
#18957=CARTESIAN_POINT('Ctrl Pts',(-3.69864765055087,2.58791326025872,5.04825615862444));
#18958=CARTESIAN_POINT('Ctrl Pts',(-3.49562448245587,2.58479315779948,5.03714236956762));
#18959=CARTESIAN_POINT('Ctrl Pts',(-3.38813739191354,2.41252976124558,5.02602858051083));
#18960=CARTESIAN_POINT('Ctrl Pts',(-3.47457055790533,2.22879774264625,5.01491479145402));
#18961=CARTESIAN_POINT('Ctrl Pts',(-3.67581071038439,2.20176908651461,5.00380100239723));
#18962=CARTESIAN_POINT('Ctrl Pts',(-3.8076604620585,2.35618343621151,4.99268721334041));
#18963=CARTESIAN_POINT('Ctrl Pts',(-3.74943623670099,2.5507035823472,4.98157342428361));
#18964=CARTESIAN_POINT('Ctrl Pts',(-3.55443132970808,2.6072830311201,4.97045963522681));
#18965=CARTESIAN_POINT('Ctrl Pts',(-3.40113594314794,2.47413397043246,4.95934584617));
#18966=CARTESIAN_POINT('Ctrl Pts',(-3.42986308323079,2.27312924603482,4.9482320571132));
#18967=CARTESIAN_POINT('Ctrl Pts',(-3.61431847264918,2.18825076147219,4.93711826805639));
#18968=CARTESIAN_POINT('Ctrl Pts',(-3.78566800170281,2.29718875637448,4.92600447899959));
#18969=CARTESIAN_POINT('Ctrl Pts',(-3.78707350316275,2.50023104850568,4.91489068994278));
#18970=CARTESIAN_POINT('Ctrl Pts',(-3.61724850562837,2.61153072525238,4.90377690088598));
#18971=CARTESIAN_POINT('Ctrl Pts',(-3.43163575527681,2.52921393024892,4.89266311182917));
#18972=CARTESIAN_POINT('Ctrl Pts',(-3.40012870750287,2.32862615950552,4.88154932277238));
#18973=CARTESIAN_POINT('Ctrl Pts',(-3.55156612044514,2.19336767439986,4.87043553371556));
#18974=CARTESIAN_POINT('Ctrl Pts',(-3.74733561262204,2.24724210028659,4.85932174465877));
#18975=CARTESIAN_POINT('Ctrl Pts',(-3.80824714766624,2.4409375641731,4.84820795560196));
#18976=CARTESIAN_POINT('Ctrl Pts',(-3.67854770676838,2.59716241130857,4.83709416654516));
#18977=CARTESIAN_POINT('Ctrl Pts',(-3.47695265907377,2.57292226739941,4.82598037748835));
#18978=CARTESIAN_POINT('Ctrl Pts',(-3.38798423798073,2.39040441106771,4.81486658843155));
#18979=CARTESIAN_POINT('Ctrl Pts',(-3.49307624828619,2.2166695061071,4.80375279937474));
#18980=CARTESIAN_POINT('Ctrl Pts',(-3.69603678113312,2.21073908131588,4.79263901031794));
#18981=CARTESIAN_POINT('Ctrl Pts',(-3.81109375907773,2.37804132176103,4.78152522126113));
#18982=CARTESIAN_POINT('Ctrl Pts',(-3.73293422537244,2.56544258942666,4.77041143220433));
#18983=CARTESIAN_POINT('Ctrl Pts',(-3.5330984876071,2.6014123787435,4.75929764314753));
#18984=CARTESIAN_POINT('Ctrl Pts',(-3.39449846284973,2.45302713362467,4.74818385409072));
#18985=CARTESIAN_POINT('Ctrl Pts',(-3.44399632559195,2.2561055517306,4.73707006503392));
#18986=CARTESIAN_POINT('Ctrl Pts',(-3.63628612072185,2.19089219021153,4.72595627597712));
#18987=CARTESIAN_POINT('Ctrl Pts',(-3.79536281804244,2.31707757843571,4.7148424869203));
#18988=CARTESIAN_POINT('Ctrl Pts',(-3.77562171244375,2.5191627995219,4.70372869786351));
#18989=CARTESIAN_POINT('Ctrl Pts',(-3.5951320617596,2.61217695880763,4.6926149088067));
#18990=CARTESIAN_POINT('Ctrl Pts',(-3.41909809015308,2.51098314144638,4.6815011197499));
#18991=CARTESIAN_POINT('Ctrl Pts',(-3.40864568819661,2.30820519608479,4.67038733069309));
#18992=CARTESIAN_POINT('Ctrl Pts',(-3.57334205793934,2.18944807577074,4.65927354163629));
#18993=CARTESIAN_POINT('Ctrl Pts',(-3.76243874437168,2.26341151952482,4.64815975257949));
#18994=CARTESIAN_POINT('Ctrl Pts',(-3.80285340590026,2.46239594847684,4.63704596352267));
#18995=CARTESIAN_POINT('Ctrl Pts',(-3.65759404449364,2.60426865816925,4.62593217446588));
#18996=CARTESIAN_POINT('Ctrl Pts',(-3.45961820100231,2.55917194847634,4.61481838540907));
#18997=CARTESIAN_POINT('Ctrl Pts',(-3.39013541016905,2.3683833492081,4.60370459635227));
#18998=CARTESIAN_POINT('Ctrl Pts',(-3.51274405843916,2.20653382897141,4.59259080729546));
#18999=CARTESIAN_POINT('Ctrl Pts',(-3.71521905956003,2.22176608912375,4.58147701823867));
#19000=CARTESIAN_POINT('Ctrl Pts',(-3.81223274881174,2.40013786922925,4.57036322918185));
#19001=CARTESIAN_POINT('Ctrl Pts',(-3.71498739615465,2.57838345602943,4.55924944012506));
#19002=CARTESIAN_POINT('Ctrl Pts',(-3.51249277582821,2.59335264259245,4.54813565106824));
#19003=CARTESIAN_POINT('Ctrl Pts',(-3.39009451003192,2.4313439624772,4.53702186201144));
#19004=CARTESIAN_POINT('Ctrl Pts',(-3.45982512000134,2.24064579833279,4.52590807295464));
#19005=CARTESIAN_POINT('Ctrl Pts',(-3.65785938670857,2.1958063415914,4.51479428389783));
#19006=CARTESIAN_POINT('Ctrl Pts',(-3.80293430182523,2.33786765727141,4.50368049484103));
#19007=CARTESIAN_POINT('Ctrl Pts',(-3.76226114657918,2.53679940854407,4.49256670578423));
#19008=CARTESIAN_POINT('Ctrl Pts',(-3.57306852864947,2.61051711444195,4.48145291672742));
#19009=CARTESIAN_POINT('Ctrl Pts',(-3.40852658196552,2.49154610870105,4.47033912767061));
#19010=CARTESIAN_POINT('Ctrl Pts',(-3.41924244609765,2.28878193021138,4.45922533861382));
#19011=CARTESIAN_POINT('Ctrl Pts',(-3.5954077095353,2.18781687475719,4.44811154955701));
#19012=CARTESIAN_POINT('Ctrl Pts',(-3.77577642802961,2.28106551532598,4.43699776050021));
#19013=CARTESIAN_POINT('Ctrl Pts',(-3.79525482929664,2.48317608801675,4.4258839714434));
#19014=CARTESIAN_POINT('Ctrl Pts',(-3.6360145897577,2.60915494542926,4.4147701823866));
#19015=CARTESIAN_POINT('Ctrl Pts',(-3.44380914946703,2.54369130588911,4.40365639332979));
#19016=CARTESIAN_POINT('Ctrl Pts',(-3.39456824409026,2.34670659273357,4.39254260427299));
#19017=CARTESIAN_POINT('Ctrl Pts',(-3.53335879551641,2.19849952038487,4.38142881521618));
#19018=CARTESIAN_POINT('Ctrl Pts',(-3.73315192133567,2.23473296627504,4.37031502615938));
#19019=CARTESIAN_POINT('Ctrl Pts',(-3.81105932334871,2.4222275030731,4.35920123710257));
#19020=CARTESIAN_POINT('Ctrl Pts',(-3.69580227747518,2.58939637532595,4.34808744804577));
#19021=CARTESIAN_POINT('Ctrl Pts',(-3.49281517917073,2.58316970871533,4.33697365898897));
#19022=CARTESIAN_POINT('Ctrl Pts',(-3.38801801175539,2.40936362032424,4.32585986993216));
#19023=CARTESIAN_POINT('Ctrl Pts',(-3.47708428355003,2.22683063907596,4.31474608087536));
#19024=CARTESIAN_POINT('Ctrl Pts',(-3.67900086652888,2.20311869118934,4.30363229181856));
#19025=CARTESIAN_POINT('Ctrl Pts',(-3.76479031853975,2.3069928942824,4.29622309911402));
#19026=CARTESIAN_POINT('Ctrl Pts',(-3.77623115053166,2.36559394454847,4.29251850276175));
#19027=CARTESIAN_POINT('Ctrl Pts',(-3.64298642568859,2.23904122513352,5.22244449171475));
#19028=CARTESIAN_POINT('Ctrl Pts',(-3.69650904770099,2.25333523436478,5.21873989536248));
#19029=CARTESIAN_POINT('Ctrl Pts',(-3.78724129001348,2.33931326491388,5.21133070265794));
#19030=CARTESIAN_POINT('Ctrl Pts',(-3.75253088002014,2.52472431243949,5.20021691360114));
#19031=CARTESIAN_POINT('Ctrl Pts',(-3.57793539445428,2.59563515581826,5.18910312454433));
#19032=CARTESIAN_POINT('Ctrl Pts',(-3.42367004762736,2.48764253337377,5.17798933548753));
#19033=CARTESIAN_POINT('Ctrl Pts',(-3.4307346156477,2.29934846267587,5.16687554643072));
#19034=CARTESIAN_POINT('Ctrl Pts',(-3.59276310781765,2.2032224269029,5.15576175737392));
#19035=CARTESIAN_POINT('Ctrl Pts',(-3.76139893017626,2.28718889057467,5.14464796831712));
#19036=CARTESIAN_POINT('Ctrl Pts',(-3.78231281136787,2.47442275264891,5.13353417926031));
#19037=CARTESIAN_POINT('Ctrl Pts',(-3.63634954853391,2.5935315757496,5.12242039020352));
#19038=CARTESIAN_POINT('Ctrl Pts',(-3.45711720940891,2.53550127459616,5.1113066011467));
#19039=CARTESIAN_POINT('Ctrl Pts',(-3.4086660712507,2.35344386065259,5.1001928120899));
#19040=CARTESIAN_POINT('Ctrl Pts',(-3.53534556618555,2.21400043804369,5.0890790230331));
#19041=CARTESIAN_POINT('Ctrl Pts',(-3.72120373880265,2.24480420972985,5.07796523397629));
#19042=CARTESIAN_POINT('Ctrl Pts',(-3.79612288401061,2.41766060518064,5.06685144491949));
#19043=CARTESIAN_POINT('Ctrl Pts',(-3.6915284647428,2.57435197006973,5.05573765586269));
#19044=CARTESIAN_POINT('Ctrl Pts',(-3.50315703593343,2.5714570386006,5.04462386680588));
#19045=CARTESIAN_POINT('Ctrl Pts',(-3.40342705430619,2.41162551570156,5.03351007774908));
#19046=CARTESIAN_POINT('Ctrl Pts',(-3.48362252720301,2.24115303619919,5.02239628869227));
#19047=CARTESIAN_POINT('Ctrl Pts',(-3.67033961674501,2.21607497923609,5.01128249963547));
#19048=CARTESIAN_POINT('Ctrl Pts',(-3.79267405938058,2.35934558206435,5.00016871057866));
#19049=CARTESIAN_POINT('Ctrl Pts',(-3.73865174939092,2.53982763346569,4.98905492152186));
#19050=CARTESIAN_POINT('Ctrl Pts',(-3.55771992126626,2.59232386680991,4.97794113246505));
#19051=CARTESIAN_POINT('Ctrl Pts',(-3.41548752844543,2.46878388345875,4.96682734340825));
#19052=CARTESIAN_POINT('Ctrl Pts',(-3.44214149347704,2.28228523166696,4.95571355435145));
#19053=CARTESIAN_POINT('Ctrl Pts',(-3.61328513970402,2.20353224223104,4.94459976529464));
#19054=CARTESIAN_POINT('Ctrl Pts',(-3.7722687469273,2.30460841961473,4.93348597623784));
#19055=CARTESIAN_POINT('Ctrl Pts',(-3.77357281641202,2.4929975923203,4.92237218718104));
#19056=CARTESIAN_POINT('Ctrl Pts',(-3.61600371859295,2.59626501412009,4.91125839812423));
#19057=CARTESIAN_POINT('Ctrl Pts',(-3.44378623564737,2.51988884269441,4.90014460906743));
#19058=CARTESIAN_POINT('Ctrl Pts',(-3.41455298280027,2.33377705392094,4.88903082001062));
#19059=CARTESIAN_POINT('Ctrl Pts',(-3.55506148790733,2.20827987871175,4.87791703095382));
#19060=CARTESIAN_POINT('Ctrl Pts',(-3.73670272277068,2.25826630477233,4.86680324189701));
#19061=CARTESIAN_POINT('Ctrl Pts',(-3.79321840516747,2.43798318944394,4.85568945284021));
#19062=CARTESIAN_POINT('Ctrl Pts',(-3.67287909006884,2.58293363005899,4.8445756637834));
#19063=CARTESIAN_POINT('Ctrl Pts',(-3.48583271732505,2.5604428444725,4.8334618747266));
#19064=CARTESIAN_POINT('Ctrl Pts',(-3.40328495315871,2.39109690379476,4.8223480856698));
#19065=CARTESIAN_POINT('Ctrl Pts',(-3.50079270226656,2.22990006804163,4.81123429661299));
#19066=CARTESIAN_POINT('Ctrl Pts',(-3.68910601607711,2.22439762907444,4.80012050755619));
#19067=CARTESIAN_POINT('Ctrl Pts',(-3.79585958284132,2.37962603168174,4.78900671849938));
#19068=CARTESIAN_POINT('Ctrl Pts',(-3.72334065223214,2.55350295854726,4.77789292944258));
#19069=CARTESIAN_POINT('Ctrl Pts',(-3.53792662385674,2.58687688661252,4.76677914038578));
#19070=CARTESIAN_POINT('Ctrl Pts',(-3.40932906062523,2.4492002810333,4.75566535132897));
#19071=CARTESIAN_POINT('Ctrl Pts',(-3.45525477055898,2.26649010025516,4.74455156227217));
#19072=CARTESIAN_POINT('Ctrl Pts',(-3.63366743052263,2.20598304481872,4.73343777321536));
#19073=CARTESIAN_POINT('Ctrl Pts',(-3.7812639095143,2.32306190876162,4.72232398415856));
#19074=CARTESIAN_POINT('Ctrl Pts',(-3.76294747645498,2.51056308015232,4.71121019510176));
#19075=CARTESIAN_POINT('Ctrl Pts',(-3.59548337024634,2.59686461040897,4.70009640604495));
#19076=CARTESIAN_POINT('Ctrl Pts',(-3.43215338647331,2.50297373016179,4.68898261698815));
#19077=CARTESIAN_POINT('Ctrl Pts',(-3.42245531157129,2.31482982689595,4.67786882793134));
#19078=CARTESIAN_POINT('Ctrl Pts',(-3.57526590348185,2.20464314896778,4.66675503887454));
#19079=CARTESIAN_POINT('Ctrl Pts',(-3.75071589443907,2.27326881228664,4.65564124981773));
#19080=CARTESIAN_POINT('Ctrl Pts',(-3.78821391798199,2.45789296894922,4.64452746076093));
#19081=CARTESIAN_POINT('Ctrl Pts',(-3.65343760790444,2.58952703458114,4.63341367170412));
#19082=CARTESIAN_POINT('Ctrl Pts',(-3.46974924928937,2.54768485607922,4.62229988264733));
#19083=CARTESIAN_POINT('Ctrl Pts',(-3.40528087994151,2.37066505394572,4.61118609359051));
#19084=CARTESIAN_POINT('Ctrl Pts',(-3.51904112945263,2.2204958606208,4.60007230453372));
#19085=CARTESIAN_POINT('Ctrl Pts',(-3.70690395130293,2.23462884177668,4.58895851547691));
#19086=CARTESIAN_POINT('Ctrl Pts',(-3.79691637417015,2.40012791950764,4.57784472642011));
#19087=CARTESIAN_POINT('Ctrl Pts',(-3.7066890065403,2.56550991102893,4.5667309373633));
#19088=CARTESIAN_POINT('Ctrl Pts',(-3.5188079813597,2.57939880404271,4.55561714830649));
#19089=CARTESIAN_POINT('Ctrl Pts',(-3.40524293147808,2.42908193706057,4.54450335924969));
#19090=CARTESIAN_POINT('Ctrl Pts',(-3.4699412353955,2.25214604354523,4.53338957019289));
#19091=CARTESIAN_POINT('Ctrl Pts',(-3.65368380095038,2.21054255261035,4.52227578113608));
#19092=CARTESIAN_POINT('Ctrl Pts',(-3.78828897582448,2.34235161294705,4.51116199207928));
#19093=CARTESIAN_POINT('Ctrl Pts',(-3.75055111349195,2.52692689356351,4.50004820302248));
#19094=CARTESIAN_POINT('Ctrl Pts',(-3.57501211420431,2.59532455339135,4.48893441396567));
#19095=CARTESIAN_POINT('Ctrl Pts',(-3.42234480097716,2.48493942568113,4.47782062490887));
#19096=CARTESIAN_POINT('Ctrl Pts',(-3.43228732456417,2.29680829576209,4.46670683585206));
#19097=CARTESIAN_POINT('Ctrl Pts',(-3.5957391251232,2.20312966817403,4.45559304679526));
#19098=CARTESIAN_POINT('Ctrl Pts',(-3.76309102655441,2.2896487577109,4.44447925773845));
#19099=CARTESIAN_POINT('Ctrl Pts',(-3.78116371408077,2.47717345113617,4.43336546868165));
#19100=CARTESIAN_POINT('Ctrl Pts',(-3.63341549535601,2.59406068914566,4.42225167962485));
#19101=CARTESIAN_POINT('Ctrl Pts',(-3.4550811025268,2.53332141770711,4.41113789056804));
#19102=CARTESIAN_POINT('Ctrl Pts',(-3.40939380590581,2.35055266171297,4.40002410151124));
#19103=CARTESIAN_POINT('Ctrl Pts',(-3.53816814591191,2.21304137056363,4.38891031245443));
#19104=CARTESIAN_POINT('Ctrl Pts',(-3.72354263755246,2.2466599276823,4.37779652339763));
#19105=CARTESIAN_POINT('Ctrl Pts',(-3.79582763226376,2.42062339265036,4.36668273434082));
#19106=CARTESIAN_POINT('Ctrl Pts',(-3.68888843603675,2.57572805195694,4.35556894528402));
#19107=CARTESIAN_POINT('Ctrl Pts',(-3.50055047393982,2.56995075029642,4.34445515622722));
#19108=CARTESIAN_POINT('Ctrl Pts',(-3.40331628955371,2.40868786826575,4.33334136717041));
#19109=CARTESIAN_POINT('Ctrl Pts',(-3.4859548427499,2.23932789420368,4.32222757811361));
#19110=CARTESIAN_POINT('Ctrl Pts',(-3.67329954627769,2.21732718588468,4.3111137890568));
#19111=CARTESIAN_POINT('Ctrl Pts',(-3.75289776062778,2.31370501427084,4.30370459635227));
#19112=CARTESIAN_POINT('Ctrl Pts',(-3.76351293272515,2.3680769545372,4.3));
#19113=CARTESIAN_POINT('Ctrl Pts',(-3.76638442018051,2.4000942147675,5.13785196366098));
#19114=CARTESIAN_POINT('Ctrl Pts',(-3.76649613151981,2.42168271873493,5.13641270219409));
#19115=CARTESIAN_POINT('Ctrl Pts',(-3.76259704654914,2.44323253526348,5.1349734407272));
#19116=CARTESIAN_POINT('Ctrl Pts',(-3.75449995403028,2.46306857948665,5.13353417926031));
#19117=CARTESIAN_POINT('Ctrl Pts',(-3.73365839042322,2.51412569368247,5.12982958290804));
#19118=CARTESIAN_POINT('Ctrl Pts',(-3.68500396947857,2.55382863471604,5.12612498655578));
#19119=CARTESIAN_POINT('Ctrl Pts',(-3.63080470248541,2.56400838837391,5.12242039020351));
#19120=CARTESIAN_POINT('Ctrl Pts',(-3.57660543549225,2.57418814203179,5.11871579385124));
#19121=CARTESIAN_POINT('Ctrl Pts',(-3.51686132245058,2.55484470831398,5.11501119749897));
#19122=CARTESIAN_POINT('Ctrl Pts',(-3.47891407623671,2.51483008913114,5.1113066011467));
#19123=CARTESIAN_POINT('Ctrl Pts',(-3.44096683002284,2.47481546994831,5.10760200479444));
#19124=CARTESIAN_POINT('Ctrl Pts',(-3.42481645063677,2.41412966530045,5.10389740844217));
#19125=CARTESIAN_POINT('Ctrl Pts',(-3.43785451009954,2.3605461925417,5.1001928120899));
#19126=CARTESIAN_POINT('Ctrl Pts',(-3.45089256956232,2.30696271978295,5.09648821573763));
#19127=CARTESIAN_POINT('Ctrl Pts',(-3.49311906787393,2.26048157891332,5.09278361938537));
#19128=CARTESIAN_POINT('Ctrl Pts',(-3.54520867913259,2.2423749704262,5.0890790230331));
#19129=CARTESIAN_POINT('Ctrl Pts',(-3.59729829039125,2.22426836193908,5.08537442668083));
#19130=CARTESIAN_POINT('Ctrl Pts',(-3.65925101459695,2.23453628583446,5.08166983032856));
#19131=CARTESIAN_POINT('Ctrl Pts',(-3.70271390090113,2.26847964702395,5.07796523397629));
#19132=CARTESIAN_POINT('Ctrl Pts',(-3.74226404132859,2.29936725748381,5.07459414387119));
#19133=CARTESIAN_POINT('Ctrl Pts',(-3.76650358790754,2.34985942080815,5.07122305376608));
#19134=CARTESIAN_POINT('Ctrl Pts',(-3.76682061973634,2.40008640134019,5.06785196366098));
#19135=CARTESIAN_POINT('Ctrl Pts',(-3.65301702171886,2.20148256743283,5.2));
#19136=CARTESIAN_POINT('Ctrl Pts',(-3.66542047547214,2.20607510650608,5.2));
#19137=CARTESIAN_POINT('Ctrl Pts',(-3.67726977303962,2.21193437262237,5.2));
#19138=CARTESIAN_POINT('Ctrl Pts',(-3.688447163997,2.21889712590693,5.2));
#19139=CARTESIAN_POINT('Ctrl Pts',(-3.69411334108481,2.22242676831449,5.2));
#19140=CARTESIAN_POINT('Ctrl Pts',(-3.69960641439008,2.22624073198774,5.2));
#19141=CARTESIAN_POINT('Ctrl Pts',(-3.70490760860864,2.23032132776193,5.2));
#19142=CARTESIAN_POINT('Ctrl Pts',(-3.70949455661916,2.2338521323121,5.2));
#19143=CARTESIAN_POINT('Ctrl Pts',(-3.71393782222619,2.23758261370384,5.2));
#19144=CARTESIAN_POINT('Ctrl Pts',(-3.71822343533123,2.24150219834368,5.2));
#19145=CARTESIAN_POINT('Ctrl Pts',(-3.72133392659836,2.24434702672511,5.2));
#19146=CARTESIAN_POINT('Ctrl Pts',(-3.72435518261367,2.24728605527231,5.2));
#19147=CARTESIAN_POINT('Ctrl Pts',(-3.72727779974184,2.25030906336475,5.2));
#19148=CARTESIAN_POINT('Ctrl Pts',(-3.73622279642463,2.25956131782473,5.2));
#19149=CARTESIAN_POINT('Ctrl Pts',(-3.74426351405243,2.26961342426582,5.2));
#19150=CARTESIAN_POINT('Ctrl Pts',(-3.75126091239845,2.28033434366482,5.2));
#19151=CARTESIAN_POINT('Ctrl Pts',(-3.75579176664188,2.28727619844431,5.2));
#19152=CARTESIAN_POINT('Ctrl Pts',(-3.75988435832116,2.29449904020269,5.2));
#19153=CARTESIAN_POINT('Ctrl Pts',(-3.76348920729151,2.30196994667654,5.2));
#19154=CARTESIAN_POINT('Ctrl Pts',(-3.76515597383801,2.30542425421759,5.2));
#19155=CARTESIAN_POINT('Ctrl Pts',(-3.76671433719502,2.30892350560647,5.2));
#19156=CARTESIAN_POINT('Ctrl Pts',(-3.76815916520543,2.31246074610162,5.2));
#19157=CARTESIAN_POINT('Ctrl Pts',(-3.77216128940432,2.32225878135629,5.2));
#19158=CARTESIAN_POINT('Ctrl Pts',(-3.77529844536059,2.33235630265294,5.2));
#19159=CARTESIAN_POINT('Ctrl Pts',(-3.77747651815115,2.34267992422407,5.2));
#19160=CARTESIAN_POINT('Ctrl Pts',(-3.77933030902448,2.35146651553144,5.2));
#19161=CARTESIAN_POINT('Ctrl Pts',(-3.78048860368035,2.36041737528633,5.2));
#19162=CARTESIAN_POINT('Ctrl Pts',(-3.78096403138949,2.36945420421056,5.2));
#19163=CARTESIAN_POINT('Ctrl Pts',(-3.781133173515,2.37266922180987,5.2));
#19164=CARTESIAN_POINT('Ctrl Pts',(-3.78121552286205,2.37589368165894,5.2));
#19165=CARTESIAN_POINT('Ctrl Pts',(-3.78121200959806,2.37911434872485,5.2));
#19166=CARTESIAN_POINT('Ctrl Pts',(-3.78119923720175,2.3908230151512,5.2));
#19167=CARTESIAN_POINT('Ctrl Pts',(-3.78005717470715,2.40251790081025,5.2));
#19168=CARTESIAN_POINT('Ctrl Pts',(-3.77783120806398,2.41402669258654,5.2));
#19169=CARTESIAN_POINT('Ctrl Pts',(-3.77668819949671,2.41993632633585,5.2));
#19170=CARTESIAN_POINT('Ctrl Pts',(-3.77525870411221,2.42579670928221,5.2));
#19171=CARTESIAN_POINT('Ctrl Pts',(-3.77354493887783,2.43158224657623,5.2));
#19172=CARTESIAN_POINT('Ctrl Pts',(-3.77185769889076,2.43727823671147,5.2));
#19173=CARTESIAN_POINT('Ctrl Pts',(-3.7698921652597,2.44290711736645,5.2));
#19174=CARTESIAN_POINT('Ctrl Pts',(-3.76766231085216,2.44841156899725,5.2));
#19175=CARTESIAN_POINT('Ctrl Pts',(-3.76420558690842,2.45694457890368,5.2));
#19176=CARTESIAN_POINT('Ctrl Pts',(-3.7601120066452,2.46519219654187,5.2));
#19177=CARTESIAN_POINT('Ctrl Pts',(-3.75539091261074,2.47305855746262,5.2));
#19178=CARTESIAN_POINT('Ctrl Pts',(-3.75297690030925,2.47708082261811,5.2));
#19179=CARTESIAN_POINT('Ctrl Pts',(-3.75039789825265,2.48100349927224,5.2));
#19180=CARTESIAN_POINT('Ctrl Pts',(-3.74766394598163,2.48480007876844,5.2));
#19181=CARTESIAN_POINT('Ctrl Pts',(-3.74222934299289,2.49234699262488,5.2));
#19182=CARTESIAN_POINT('Ctrl Pts',(-3.73617584476421,2.49941040205976,5.2));
#19183=CARTESIAN_POINT('Ctrl Pts',(-3.7295081017749,2.50587917960273,5.2));
#19184=CARTESIAN_POINT('Ctrl Pts',(-3.72872963243595,2.50663441941712,5.2));
#19185=CARTESIAN_POINT('Ctrl Pts',(-3.72794277607053,2.50738152833223,5.2));
#19186=CARTESIAN_POINT('Ctrl Pts',(-3.72714768981588,2.50812044061668,5.2));
#19187=CARTESIAN_POINT('Origin',(-3.6,2.4,4.7));
#19188=CARTESIAN_POINT('Origin',(3.6,2.4,4.3));
#19189=CARTESIAN_POINT('Ctrl Pts',(3.43648706727485,2.36807695453719,4.3));
#19190=CARTESIAN_POINT('Ctrl Pts',(3.43713128683271,2.3597806326638,4.3));
#19191=CARTESIAN_POINT('Ctrl Pts',(3.43844439010238,2.35157023568352,4.3));
#19192=CARTESIAN_POINT('Ctrl Pts',(3.44036779366958,2.34349709838219,4.3));
#19193=CARTESIAN_POINT('Ctrl Pts',(3.44142971905211,2.33903985936946,4.3));
#19194=CARTESIAN_POINT('Ctrl Pts',(3.44267796535882,2.33462439474099,4.3));
#19195=CARTESIAN_POINT('Ctrl Pts',(3.44410466805123,2.33025917432088,4.3));
#19196=CARTESIAN_POINT('Ctrl Pts',(3.44564438355751,2.32554817349018,4.3));
#19197=CARTESIAN_POINT('Ctrl Pts',(3.44738955334548,2.3209035962062,4.3));
#19198=CARTESIAN_POINT('Ctrl Pts',(3.4493265481332,2.31634215395336,4.3));
#19199=CARTESIAN_POINT('Ctrl Pts',(3.45254731917628,2.30875753823018,4.3));
#19200=CARTESIAN_POINT('Ctrl Pts',(3.45629959311852,2.30139710694769,4.3));
#19201=CARTESIAN_POINT('Ctrl Pts',(3.46054037353588,2.29430908064149,4.3));
#19202=CARTESIAN_POINT('Ctrl Pts',(3.46239353776121,2.29121170810954,4.3));
#19203=CARTESIAN_POINT('Ctrl Pts',(3.46433984867298,2.28816727138872,4.3));
#19204=CARTESIAN_POINT('Ctrl Pts',(3.46636983737831,2.28518826034786,4.3));
#19205=CARTESIAN_POINT('Ctrl Pts',(3.47324583140019,2.27509773026055,4.3));
#19206=CARTESIAN_POINT('Ctrl Pts',(3.48109365784268,2.26572974302294,4.3));
#19207=CARTESIAN_POINT('Ctrl Pts',(3.48977951837809,2.25723278343533,4.3));
#19208=CARTESIAN_POINT('Ctrl Pts',(3.49400932884437,2.25309496330239,4.3));
#19209=CARTESIAN_POINT('Ctrl Pts',(3.49843865454892,2.24916389122995,4.3));
#19210=CARTESIAN_POINT('Ctrl Pts',(3.50305598018317,2.24545876796073,4.3));
#19211=CARTESIAN_POINT('Ctrl Pts',(3.50696193979743,2.24232447269942,4.3));
#19212=CARTESIAN_POINT('Ctrl Pts',(3.51100698863209,2.23934939909905,4.3));
#19213=CARTESIAN_POINT('Ctrl Pts',(3.51515874429581,2.23656266075085,4.3));
#19214=CARTESIAN_POINT('Ctrl Pts',(3.52023402885856,2.23315603202204,4.3));
#19215=CARTESIAN_POINT('Ctrl Pts',(3.52547424287705,2.23002554171617,4.3));
#19216=CARTESIAN_POINT('Ctrl Pts',(3.53086412680946,2.22718930631114,4.3));
#19217=CARTESIAN_POINT('Ctrl Pts',(3.53843721702836,2.22320423596943,4.3));
#19218=CARTESIAN_POINT('Ctrl Pts',(3.54630546669305,2.21979946806346,4.3));
#19219=CARTESIAN_POINT('Ctrl Pts',(3.55440208317939,2.21695927394856,4.3));
#19220=CARTESIAN_POINT('Ctrl Pts',(3.56031223293849,2.21488606564082,4.3));
#19221=CARTESIAN_POINT('Ctrl Pts',(3.56634429400461,2.21311389140606,4.3));
#19222=CARTESIAN_POINT('Ctrl Pts',(3.57247452264395,2.21164027909917,4.3));
#19223=CARTESIAN_POINT('Ctrl Pts',(3.57600246534631,2.21079221614916,4.3));
#19224=CARTESIAN_POINT('Ctrl Pts',(3.57955843058062,2.21004433773534,4.3));
#19225=CARTESIAN_POINT('Ctrl Pts',(3.58312961367547,2.20939690917763,4.3));
#19226=CARTESIAN_POINT('Ctrl Pts',(3.59464652648698,2.20730897975681,4.3));
#19227=CARTESIAN_POINT('Ctrl Pts',(3.60634454881448,2.20625732608158,4.3));
#19228=CARTESIAN_POINT('Ctrl Pts',(3.61806689528204,2.2062086557371,4.3));
#19229=CARTESIAN_POINT('Ctrl Pts',(3.62473122101744,2.20618098593309,4.3));
#19230=CARTESIAN_POINT('Ctrl Pts',(3.63140379711974,2.20647808078856,4.3));
#19231=CARTESIAN_POINT('Ctrl Pts',(3.63805748358195,2.20709863975089,4.3));
#19232=CARTESIAN_POINT('Ctrl Pts',(3.64215439115276,2.20748073961769,4.3));
#19233=CARTESIAN_POINT('Ctrl Pts',(3.64624620849006,2.20798586737994,4.3));
#19234=CARTESIAN_POINT('Ctrl Pts',(3.65032009844121,2.20861337585159,4.3));
#19235=CARTESIAN_POINT('Ctrl Pts',(3.66357602962435,2.2106552103677,4.3));
#19236=CARTESIAN_POINT('Ctrl Pts',(3.67655558408475,2.21397441829708,4.3));
#19237=CARTESIAN_POINT('Ctrl Pts',(3.68904456814691,2.21853837010126,4.3));
#19238=CARTESIAN_POINT('Ctrl Pts',(3.69937753051516,2.22231442922732,4.3));
#19239=CARTESIAN_POINT('Ctrl Pts',(3.7093756794575,2.22694342372598,4.3));
#19240=CARTESIAN_POINT('Ctrl Pts',(3.71891590137671,2.23243384744346,4.3));
#19241=CARTESIAN_POINT('Ctrl Pts',(3.72007018093634,2.23309813847615,4.3));
#19242=CARTESIAN_POINT('Ctrl Pts',(3.72121774557788,2.23377506987061,4.3));
#19243=CARTESIAN_POINT('Ctrl Pts',(3.72235851517116,2.23446447326396,4.3));
#19244=CARTESIAN_POINT('Ctrl Pts',(3.78826275096636,2.31767678198967,4.3));
#19245=CARTESIAN_POINT('Ctrl Pts',(3.79091867322995,2.32572936860323,4.3));
#19246=CARTESIAN_POINT('Ctrl Pts',(3.79302804064853,2.33393960507108,4.3));
#19247=CARTESIAN_POINT('Ctrl Pts',(3.79460323981381,2.34225613442594,4.3));
#19248=CARTESIAN_POINT('Ctrl Pts',(3.79578956453863,2.34851953566168,4.3));
#19249=CARTESIAN_POINT('Ctrl Pts',(3.79667271897105,2.35484328449916,4.3));
#19250=CARTESIAN_POINT('Ctrl Pts',(3.79725488312451,2.36120517356094,4.3));
#19251=CARTESIAN_POINT('Ctrl Pts',(3.7976908683603,2.36596961961323,4.3));
#19252=CARTESIAN_POINT('Ctrl Pts',(3.79795758133253,2.37075408813906,4.3));
#19253=CARTESIAN_POINT('Ctrl Pts',(3.79805590956906,2.3755369878883,4.3));
#19254=CARTESIAN_POINT('Ctrl Pts',(3.79826159173226,2.3855418166282,4.3));
#19255=CARTESIAN_POINT('Ctrl Pts',(3.79773306912215,2.39555473221079,4.3));
#19256=CARTESIAN_POINT('Ctrl Pts',(3.79647804098653,2.40548740413607,4.3));
#19257=CARTESIAN_POINT('Ctrl Pts',(3.79582247707096,2.41067573507037,4.3));
#19258=CARTESIAN_POINT('Ctrl Pts',(3.79496739950913,2.41584508273998,4.3));
#19259=CARTESIAN_POINT('Ctrl Pts',(3.79391843118089,2.42095777287915,4.3));
#19260=CARTESIAN_POINT('Ctrl Pts',(3.79135148096571,2.43346913351755,4.3));
#19261=CARTESIAN_POINT('Ctrl Pts',(3.78762422716575,2.44567369959671,4.3));
#19262=CARTESIAN_POINT('Ctrl Pts',(3.78275033841106,2.45738291584384,4.3));
#19263=CARTESIAN_POINT('Ctrl Pts',(3.78051276867504,2.46275853872441,4.3));
#19264=CARTESIAN_POINT('Ctrl Pts',(3.77803290925375,2.46802940870032,4.3));
#19265=CARTESIAN_POINT('Ctrl Pts',(3.77530915968311,2.47317482247228,4.3));
#19266=CARTESIAN_POINT('Ctrl Pts',(3.7735285304889,2.4765385950002,4.3));
#19267=CARTESIAN_POINT('Ctrl Pts',(3.77164255910733,2.47985045045176,4.3));
#19268=CARTESIAN_POINT('Ctrl Pts',(3.76965384065618,2.48309856403818,4.3));
#19269=CARTESIAN_POINT('Ctrl Pts',(3.76538142018115,2.49007657894212,4.3));
#19270=CARTESIAN_POINT('Ctrl Pts',(3.76065254798511,2.4967339395313,4.3));
#19271=CARTESIAN_POINT('Ctrl Pts',(3.75546934621649,2.50301830246242,4.3));
#19272=CARTESIAN_POINT('Ctrl Pts',(3.7497639943478,2.5099357452696,4.3));
#19273=CARTESIAN_POINT('Ctrl Pts',(3.74350797317419,2.51640155748529,4.3));
#19274=CARTESIAN_POINT('Ctrl Pts',(3.73677354924283,2.52238273959095,4.3));
#19275=CARTESIAN_POINT('Ctrl Pts',(3.73252952287629,2.52615207380843,4.3));
#19276=CARTESIAN_POINT('Ctrl Pts',(3.72809532803267,2.52972869286917,4.3));
#19277=CARTESIAN_POINT('Ctrl Pts',(3.72348818609076,2.53310156466662,4.3));
#19278=CARTESIAN_POINT('Ctrl Pts',(3.72067461067475,2.53516137295782,4.3));
#19279=CARTESIAN_POINT('Ctrl Pts',(3.71779994290363,2.53714246961825,4.3));
#19280=CARTESIAN_POINT('Ctrl Pts',(3.71487521534485,2.53903869288715,4.3));
#19281=CARTESIAN_POINT('Ctrl Pts',(3.70626340571031,2.54462208945595,4.3));
#19282=CARTESIAN_POINT('Ctrl Pts',(3.69720115342902,2.54948407839451,4.3));
#19283=CARTESIAN_POINT('Ctrl Pts',(3.68779739443943,2.55357358531277,4.3));
#19284=CARTESIAN_POINT('Ctrl Pts',(3.67897143105616,2.55741182046492,4.3));
#19285=CARTESIAN_POINT('Ctrl Pts',(3.66984396791867,2.56056952878093,4.3));
#19286=CARTESIAN_POINT('Ctrl Pts',(3.66050457512214,2.56298263453418,4.3));
#19287=CARTESIAN_POINT('Ctrl Pts',(3.657017355811,2.56388365981129,4.3));
#19288=CARTESIAN_POINT('Ctrl Pts',(3.65350912975721,2.56467838913094,4.3));
#19289=CARTESIAN_POINT('Ctrl Pts',(3.64998789179307,2.5653638764114,4.3));
#19290=CARTESIAN_POINT('Ctrl Pts',(3.63890668202576,2.56752108033372,4.3));
#19291=CARTESIAN_POINT('Ctrl Pts',(3.62768560566387,2.56860271836266,4.3));
#19292=CARTESIAN_POINT('Ctrl Pts',(3.61647526972934,2.56851225659508,4.3));
#19293=CARTESIAN_POINT('Ctrl Pts',(3.61029339424358,2.56846237197194,4.3));
#19294=CARTESIAN_POINT('Ctrl Pts',(3.60411488972487,2.56805522437202,4.3));
#19295=CARTESIAN_POINT('Ctrl Pts',(3.59796731823988,2.56726810386747,4.3));
#19296=CARTESIAN_POINT('Ctrl Pts',(3.5968916538024,2.56713037833848,4.3));
#19297=CARTESIAN_POINT('Ctrl Pts',(3.59581694274575,2.56698100748364,4.3));
#19298=CARTESIAN_POINT('Ctrl Pts',(3.59474333802771,2.56682006235004,4.3));
#19299=CARTESIAN_POINT('Origin',(3.6,2.4,5.35459252805377));
#19300=CARTESIAN_POINT('Ctrl Pts',(3.39434265438876,2.4001499379742,5.17959252805377));
#19301=CARTESIAN_POINT('Ctrl Pts',(3.3942608381295,2.40997903394326,5.17905813053169));
#19302=CARTESIAN_POINT('Ctrl Pts',(3.39937061019979,2.4878631610827,5.17481913665734));
#19303=CARTESIAN_POINT('Ctrl Pts',(3.4989044460774,2.62084298387434,5.16687554643073));
#19304=CARTESIAN_POINT('Ctrl Pts',(3.73070050850364,2.60468899581803,5.15576175737391));
#19305=CARTESIAN_POINT('Ctrl Pts',(3.84286218134804,2.40121305191012,5.14464796831713));
#19306=CARTESIAN_POINT('Ctrl Pts',(3.73273070961532,2.19661070737624,5.1335341792603));
#19307=CARTESIAN_POINT('Ctrl Pts',(3.50110863285869,2.17818091869864,5.12242039020352));
#19308=CARTESIAN_POINT('Ctrl Pts',(3.39978420373419,2.31073763553012,5.11443983980133));
#19309=CARTESIAN_POINT('Ctrl Pts',(3.39427096205728,2.38932589106744,5.11016388575141));
#19310=CARTESIAN_POINT('Ctrl Pts',(3.39436118415265,2.39983962587988,5.10959252805377));
#19311=CARTESIAN_POINT('Ctrl Pts',(3.39473291096846,2.39977036782444,5.18540747194623));
#19312=CARTESIAN_POINT('Ctrl Pts',(3.39508769603641,2.44679019469361,5.18286245525962));
#19313=CARTESIAN_POINT('Ctrl Pts',(3.43434460318779,2.56295297845058,5.17661284222074));
#19314=CARTESIAN_POINT('Ctrl Pts',(3.62721323264599,2.64128528195604,5.16665863282959));
#19315=CARTESIAN_POINT('Ctrl Pts',(3.81747536314189,2.50809334538988,5.15554484377278));
#19316=CARTESIAN_POINT('Ctrl Pts',(3.80876232811303,2.27586209318291,5.14443105471598));
#19317=CARTESIAN_POINT('Ctrl Pts',(3.60892557137656,2.15730570431671,5.13331726565918));
#19318=CARTESIAN_POINT('Ctrl Pts',(3.42787436374214,2.24745398081386,5.12364273806926));
#19319=CARTESIAN_POINT('Ctrl Pts',(3.39500774851697,2.35820797614884,5.11767280683161));
#19320=CARTESIAN_POINT('Ctrl Pts',(3.39479089114249,2.40011619889285,5.11540747194623));
#19321=CARTESIAN_POINT('Ctrl Pts',(3.72690708798524,2.50793586530485,5.2));
#19322=CARTESIAN_POINT('Ctrl Pts',(3.76279833110066,2.46573623930395,5.19629540364773));
#19323=CARTESIAN_POINT('Ctrl Pts',(3.78852074717293,2.34341311981147,5.1888862109432));
#19324=CARTESIAN_POINT('Ctrl Pts',(3.65451258117961,2.21065853310285,5.17777242188639));
#19325=CARTESIAN_POINT('Ctrl Pts',(3.47057722493071,2.25164322990955,5.16665863282959));
#19326=CARTESIAN_POINT('Ctrl Pts',(3.405121385579,2.4282098150683,5.15554484377278));
#19327=CARTESIAN_POINT('Ctrl Pts',(3.5180312968317,2.57906042639477,5.14443105471598));
#19328=CARTESIAN_POINT('Ctrl Pts',(3.70597252569269,2.56596270448124,5.13331726565917));
#19329=CARTESIAN_POINT('Ctrl Pts',(3.79691368493775,2.4009835476249,5.12220347660237));
#19330=CARTESIAN_POINT('Ctrl Pts',(3.70761862135009,2.23509110037173,5.11108968754557));
#19331=CARTESIAN_POINT('Ctrl Pts',(3.51981846080671,2.22014814967852,5.09997589848877));
#19332=CARTESIAN_POINT('Ctrl Pts',(3.40540964822557,2.3698223862213,5.08886210943195));
#19333=CARTESIAN_POINT('Ctrl Pts',(3.46911145369901,2.54712015828428,5.07774832037516));
#19334=CARTESIAN_POINT('Ctrl Pts',(3.65261709875363,2.58975637037653,5.06663453131834));
#19335=CARTESIAN_POINT('Ctrl Pts',(3.78796168225801,2.4587068294695,5.05552074226155));
#19336=CARTESIAN_POINT('Ctrl Pts',(3.75126282351006,2.27392205963726,5.04440695320474));
#19337=CARTESIAN_POINT('Ctrl Pts',(3.576111378403,2.20453795937386,5.03329316414794));
#19338=CARTESIAN_POINT('Ctrl Pts',(3.42282546383512,2.31406243118482,5.02217937509113));
#19339=CARTESIAN_POINT('Ctrl Pts',(3.43170940937961,2.50224655949829,5.01106558603433));
#19340=CARTESIAN_POINT('Ctrl Pts',(3.59463164213028,2.59684323978071,4.99995179697753));
#19341=CARTESIAN_POINT('Ctrl Pts',(3.762467593188,2.51126707661319,4.98883800792072));
#19342=CARTESIAN_POINT('Ctrl Pts',(3.78159511395878,2.32384689323348,4.97772421886391));
#19343=CARTESIAN_POINT('Ctrl Pts',(3.63450656736167,2.20613051367693,4.96661042980712));
#19344=CARTESIAN_POINT('Ctrl Pts',(3.45583376839362,2.26586507280002,4.95549664075031));
#19345=CARTESIAN_POINT('Ctrl Pts',(3.40911795613805,2.44837485237297,4.94438285169351));
#19346=CARTESIAN_POINT('Ctrl Pts',(3.53711864339547,2.58660658076597,4.9332690626367));
#19347=CARTESIAN_POINT('Ctrl Pts',(3.72267534946784,2.5540351896186,4.9221552735799));
#19348=CARTESIAN_POINT('Ctrl Pts',(3.79594591694334,2.38047364248689,4.91104148452309));
#19349=CARTESIAN_POINT('Ctrl Pts',(3.6898649644607,2.22478479185514,4.89992769546629));
#19350=CARTESIAN_POINT('Ctrl Pts',(3.5015295908702,2.22947240830188,4.88881390640948));
#19351=CARTESIAN_POINT('Ctrl Pts',(3.40332529948609,2.39024586335038,4.87770011735268));
#19352=CARTESIAN_POINT('Ctrl Pts',(3.48513959192542,2.5599473902907,4.86658632829587));
#19353=CARTESIAN_POINT('Ctrl Pts',(3.67208691848091,2.58324725697266,4.85547253923907));
#19354=CARTESIAN_POINT('Ctrl Pts',(3.79305227102963,2.43881883118157,4.84435875018227));
#19355=CARTESIAN_POINT('Ctrl Pts',(3.73731469054324,2.25885908897487,4.83324496112546));
#19356=CARTESIAN_POINT('Ctrl Pts',(3.55589141654812,2.20808722327608,4.82213117206866));
#19357=CARTESIAN_POINT('Ctrl Pts',(3.41484122921187,2.33297529855171,4.81101738301186));
#19358=CARTESIAN_POINT('Ctrl Pts',(3.44326896462127,2.51921184317472,4.79990359395504));
#19359=CARTESIAN_POINT('Ctrl Pts',(3.61515439416365,2.59633243578568,4.78878980489825));
#19360=CARTESIAN_POINT('Ctrl Pts',(3.77316883486553,2.49374772336074,4.77767601584144));
#19361=CARTESIAN_POINT('Ctrl Pts',(3.77267987714682,2.30535465657222,4.76656222678464));
#19362=CARTESIAN_POINT('Ctrl Pts',(3.61413506955264,2.20359154597435,4.75544843772783));
#19363=CARTESIAN_POINT('Ctrl Pts',(3.44265227249432,2.28160332076952,4.74433464867103));
#19364=CARTESIAN_POINT('Ctrl Pts',(3.41519163486656,2.46798491877402,4.73322085961423));
#19365=CARTESIAN_POINT('Ctrl Pts',(3.55688818971484,2.59213914962324,4.72210707055742));
#19366=CARTESIAN_POINT('Ctrl Pts',(3.73804547343831,2.54042623781615,4.71099328150061));
#19367=CARTESIAN_POINT('Ctrl Pts',(3.79284816978155,2.36017959799409,4.69987949244381));
#19368=CARTESIAN_POINT('Ctrl Pts',(3.67113474927674,2.2163810237221,4.68876570338701));
#19369=CARTESIAN_POINT('Ctrl Pts',(3.48431088603601,2.24065098081811,4.67765191433021));
#19370=CARTESIAN_POINT('Ctrl Pts',(3.4033785808103,2.41077490231207,4.6665381252734));
#19371=CARTESIAN_POINT('Ctrl Pts',(3.50241609040748,2.57103643352413,4.65542433621659));
#19372=CARTESIAN_POINT('Ctrl Pts',(3.69077325913151,2.57474637744638,4.64431054715979));
#19373=CARTESIAN_POINT('Ctrl Pts',(3.79604463433366,2.41850898033344,4.63319675810299));
#19374=CARTESIAN_POINT('Ctrl Pts',(3.72187413243292,2.24533010361481,4.62208296904618));
#19375=CARTESIAN_POINT('Ctrl Pts',(3.5361508549695,2.21372233713422,4.61096917998938));
#19376=CARTESIAN_POINT('Ctrl Pts',(3.40886942405137,2.35261662800557,4.59985539093258));
#19377=CARTESIAN_POINT('Ctrl Pts',(3.45653197686655,2.53488145663037,4.58874160187577));
#19378=CARTESIAN_POINT('Ctrl Pts',(3.63551243829507,2.5936877583357,4.57762781281897));
#19379=CARTESIAN_POINT('Ctrl Pts',(3.78198796221116,2.47520945827968,4.56651402376216));
#19380=CARTESIAN_POINT('Ctrl Pts',(3.76188784043654,2.28789108810318,4.55540023470536));
#19381=CARTESIAN_POINT('Ctrl Pts',(3.5936099423673,2.20318727643507,4.54428644564855));
#19382=CARTESIAN_POINT('Ctrl Pts',(3.43118093653762,2.29862838255851,4.53317265659175));
#19383=CARTESIAN_POINT('Ctrl Pts',(3.42327393399308,2.4868560799498,4.52205886753494));
#19384=CARTESIAN_POINT('Ctrl Pts',(3.57712630395541,2.59558342196495,4.51094507847815));
#19385=CARTESIAN_POINT('Ctrl Pts',(3.75191522715083,2.52529104055601,4.49983128942133));
#19386=CARTESIAN_POINT('Ctrl Pts',(3.78765442042343,2.34031834729253,4.48871750036454));
#19387=CARTESIAN_POINT('Ctrl Pts',(3.65163139388737,2.20997295066536,4.47760371130772));
#19388=CARTESIAN_POINT('Ctrl Pts',(3.4683495682865,2.25356146118509,4.46648992225093));
#19389=CARTESIAN_POINT('Ctrl Pts',(3.40556887324678,2.431186839349,4.45537613319411));
#19390=CARTESIAN_POINT('Ctrl Pts',(3.52075319873735,2.58026652505992,4.44426234413732));
#19391=CARTESIAN_POINT('Ctrl Pts',(3.70847300970163,2.56434626551467,4.43314855508051));
#19392=CARTESIAN_POINT('Ctrl Pts',(3.79690626562936,2.39799790621595,4.4220347660237));
#19393=CARTESIAN_POINT('Ctrl Pts',(3.7051089416811,2.23348228455085,4.4109209769669));
#19394=CARTESIAN_POINT('Ctrl Pts',(3.51710429525804,2.22138181878176,4.3998071879101));
#19395=CARTESIAN_POINT('Ctrl Pts',(3.40497485954275,2.37277339597561,4.38869339885329));
#19396=CARTESIAN_POINT('Ctrl Pts',(3.47135448294965,2.54908419847293,4.37757960979649));
#19397=CARTESIAN_POINT('Ctrl Pts',(3.65548413352142,2.58893973580292,4.36646582073968));
#19398=CARTESIAN_POINT('Ctrl Pts',(3.78882987626983,2.45585019704184,4.35535203168288));
#19399=CARTESIAN_POINT('Ctrl Pts',(3.7493347906086,2.27165314263956,4.34423824262608));
#19400=CARTESIAN_POINT('Ctrl Pts',(3.57315728718835,2.20490778239848,4.33312445356927));
#19401=CARTESIAN_POINT('Ctrl Pts',(3.4215383866044,2.31678389237007,4.32201066451247));
#19402=CARTESIAN_POINT('Ctrl Pts',(3.43328916816391,2.50472575846861,4.31089687545566));
#19403=CARTESIAN_POINT('Ctrl Pts',(3.59758812791782,2.59701775419156,4.29978308639886));
#19404=CARTESIAN_POINT('Ctrl Pts',(3.76418967154123,2.50855366821667,4.28866929734205));
#19405=CARTESIAN_POINT('Ctrl Pts',(3.77483953817107,2.38400982617006,4.28126010463752));
#19406=CARTESIAN_POINT('Ctrl Pts',(3.75264423560529,2.33325198627316,4.27755550828525));
#19407=CARTESIAN_POINT('Ctrl Pts',(3.73677806246588,2.51633123698097,5.20748149723825));
#19408=CARTESIAN_POINT('Ctrl Pts',(3.77546096639785,2.47084927712496,5.20377690088598));
#19409=CARTESIAN_POINT('Ctrl Pts',(3.80318410060701,2.33901172932062,5.19636770818144));
#19410=CARTESIAN_POINT('Ctrl Pts',(3.658752630386,2.19593134317562,5.18525391912464));
#19411=CARTESIAN_POINT('Ctrl Pts',(3.46051057751011,2.24010387529317,5.17414013006783));
#19412=CARTESIAN_POINT('Ctrl Pts',(3.3899635101576,2.43040400586618,5.16302634101103));
#19413=CARTESIAN_POINT('Ctrl Pts',(3.5116556799136,2.59298794555462,5.15191255195423));
#19414=CARTESIAN_POINT('Ctrl Pts',(3.71421518662967,2.57887146826017,5.14079876289742));
#19415=CARTESIAN_POINT('Ctrl Pts',(3.81222985040785,2.40106004905331,5.12968497384063));
#19416=CARTESIAN_POINT('Ctrl Pts',(3.7159893174385,2.22226430270657,5.11857118478381));
#19417=CARTESIAN_POINT('Ctrl Pts',(3.5135818514907,2.20615907268523,5.10745739572702));
#19418=CARTESIAN_POINT('Ctrl Pts',(3.3902741941935,2.36747513785065,5.0963436066702));
#19419=CARTESIAN_POINT('Ctrl Pts',(3.45893079696141,2.55856332785872,5.08522981761341));
#19420=CARTESIAN_POINT('Ctrl Pts',(3.65670971522832,2.60451583195793,5.07411602855659));
#19421=CARTESIAN_POINT('Ctrl Pts',(3.80258155100106,2.46327311197376,5.0630022394998));
#19422=CARTESIAN_POINT('Ctrl Pts',(3.76302821419424,2.26411557718108,5.05188845044299));
#19423=CARTESIAN_POINT('Ctrl Pts',(3.57425329484041,2.18933470441319,5.04077466138619));
#19424=CARTESIAN_POINT('Ctrl Pts',(3.40904463131529,2.30737811148155,5.02966087232938));
#19425=CARTESIAN_POINT('Ctrl Pts',(3.41861958002714,2.51019941063974,5.01854708327258));
#19426=CARTESIAN_POINT('Ctrl Pts',(3.59421408528317,2.61215392594813,5.00743329421578));
#19427=CARTESIAN_POINT('Ctrl Pts',(3.77510450332242,2.51992155361066,4.99631950515897));
#19428=CARTESIAN_POINT('Ctrl Pts',(3.79571978393707,2.31792361987304,4.98520571610216));
#19429=CARTESIAN_POINT('Ctrl Pts',(3.63719052655772,2.19105112936158,4.97409192704537));
#19430=CARTESIAN_POINT('Ctrl Pts',(3.44462035852227,2.25543190894468,4.96297813798855));
#19431=CARTESIAN_POINT('Ctrl Pts',(3.3942709384207,2.4521375022049,4.95186434893175));
#19432=CARTESIAN_POINT('Ctrl Pts',(3.53222766152672,2.6011210482075,4.94075055987495));
#19433=CARTESIAN_POINT('Ctrl Pts',(3.73221717461903,2.56601621802281,4.92963677081814));
#19434=CARTESIAN_POINT('Ctrl Pts',(3.81118680834224,2.37895486067752,4.91852298176134));
#19435=CARTESIAN_POINT('Ctrl Pts',(3.69685476136628,2.21115635804835,4.90740919270453));
#19436=CARTESIAN_POINT('Ctrl Pts',(3.49387045290517,2.21620858251703,4.89629540364774));
#19437=CARTESIAN_POINT('Ctrl Pts',(3.38802772249033,2.38948717575083,4.88518161459092));
#19438=CARTESIAN_POINT('Ctrl Pts',(3.47620562160949,2.57238827624017,4.87406782553412));
#19439=CARTESIAN_POINT('Ctrl Pts',(3.67769391919309,2.59750043247249,4.86295403647732));
#19440=CARTESIAN_POINT('Ctrl Pts',(3.80806809143035,2.44183820305468,4.85184024742052));
#19441=CARTESIAN_POINT('Ctrl Pts',(3.74799517992873,2.24788099190383,4.84072645836371));
#19442=CARTESIAN_POINT('Ctrl Pts',(3.55246060185887,2.19316003401009,4.82961266930691));
#19443=CARTESIAN_POINT('Ctrl Pts',(3.40043937404102,2.32776204271177,4.8184988802501));
#19444=CARTESIAN_POINT('Ctrl Pts',(3.43107825033486,2.52848427295347,4.8073850911933));
#19445=CARTESIAN_POINT('Ctrl Pts',(3.61633311980013,2.61160339105013,4.79627130213649));
#19446=CARTESIAN_POINT('Ctrl Pts',(3.78663809948217,2.50103952557292,4.78515751307969));
#19447=CARTESIAN_POINT('Ctrl Pts',(3.78611111008816,2.29799303647267,4.77404372402288));
#19448=CARTESIAN_POINT('Ctrl Pts',(3.61523451098693,2.18831467792663,4.76292993496608));
#19449=CARTESIAN_POINT('Ctrl Pts',(3.43041359120824,2.27239429534918,4.75181614590927));
#19450=CARTESIAN_POINT('Ctrl Pts',(3.40081703463734,2.47327286138574,4.74070235685248));
#19451=CARTESIAN_POINT('Ctrl Pts',(3.55353490515134,2.60708394642517,4.72958856779567));
#19452=CARTESIAN_POINT('Ctrl Pts',(3.74878280393034,2.55134874680995,4.71847477873887));
#19453=CARTESIAN_POINT('Ctrl Pts',(3.80784811496013,2.35708232282806,4.70736098968206));
#19454=CARTESIAN_POINT('Ctrl Pts',(3.67666768920898,2.2020989354812,4.69624720062525));
#19455=CARTESIAN_POINT('Ctrl Pts',(3.47531245805411,2.22825663683913,4.68513341156846));
#19456=CARTESIAN_POINT('Ctrl Pts',(3.38808514809522,2.41161298620039,4.67401962251165));
#19457=CARTESIAN_POINT('Ctrl Pts',(3.49482590536264,2.58433983759226,4.66290583345484));
#19458=CARTESIAN_POINT('Ctrl Pts',(3.69783370420702,2.58833834507989,4.65179204439804));
#19459=CARTESIAN_POINT('Ctrl Pts',(3.811293204081,2.419948629414,4.64067825534124));
#19460=CARTESIAN_POINT('Ctrl Pts',(3.73135363803182,2.23329970701222,4.62956446628443));
#19461=CARTESIAN_POINT('Ctrl Pts',(3.53118459744037,2.19923345329287,4.61845067722763));
#19462=CARTESIAN_POINT('Ctrl Pts',(3.39400307523184,2.34893109662045,4.60733688817082));
#19463=CARTESIAN_POINT('Ctrl Pts',(3.44537287442694,2.54537268637529,4.59622309911402));
#19464=CARTESIAN_POINT('Ctrl Pts',(3.6382746352513,2.60875300764603,4.58510931005721));
#19465=CARTESIAN_POINT('Ctrl Pts',(3.79614318836354,2.48105933361106,4.57399552100041));
#19466=CARTESIAN_POINT('Ctrl Pts',(3.77447965675701,2.27917113222085,4.56288173194361));
#19467=CARTESIAN_POINT('Ctrl Pts',(3.59311291657604,2.18787896385287,4.5517679428868));
#19468=CARTESIAN_POINT('Ctrl Pts',(3.4180500019796,2.29074358538356,4.54065415383));
#19469=CARTESIAN_POINT('Ctrl Pts',(3.40952798398103,2.4936118424709,4.5295403647732));
#19470=CARTESIAN_POINT('Ctrl Pts',(3.57534716243134,2.61079611810118,4.51842657571639));
#19471=CARTESIAN_POINT('Ctrl Pts',(3.76373136251596,2.53503631706984,4.50731278665959));
#19472=CARTESIAN_POINT('Ctrl Pts',(3.80225038999918,2.33567624195239,4.49619899760278));
#19473=CARTESIAN_POINT('Ctrl Pts',(3.65564734114102,2.19519243537347,4.48508520854597));
#19474=CARTESIAN_POINT('Ctrl Pts',(3.45810965125396,2.24217130873125,4.47397141948918));
#19475=CARTESIAN_POINT('Ctrl Pts',(3.39044580391398,2.4336125864072,4.46285763043236));
#19476=CARTESIAN_POINT('Ctrl Pts',(3.51458929437743,2.59428785591567,4.45174384137557));
#19477=CARTESIAN_POINT('Ctrl Pts',(3.71691016106647,2.57712930087258,4.44063005231875));
#19478=CARTESIAN_POINT('Ctrl Pts',(3.8122218540174,2.39784218113421,4.42951626326196));
#19479=CARTESIAN_POINT('Ctrl Pts',(3.71328443209297,2.22053035140142,4.41840247420515));
#19480=CARTESIAN_POINT('Ctrl Pts',(3.5106565751263,2.2074886979437,4.40728868514835));
#19481=CARTESIAN_POINT('Ctrl Pts',(3.38980558716325,2.3706556804265,4.39617489609155));
#19482=CARTESIAN_POINT('Ctrl Pts',(3.46134829152241,2.56068013327812,4.38506110703473));
#19483=CARTESIAN_POINT('Ctrl Pts',(3.65979975114976,2.60363567863874,4.37394731797794));
#19484=CARTESIAN_POINT('Ctrl Pts',(3.80351727410895,2.46019428749802,4.36283352892113));
#19485=CARTESIAN_POINT('Ctrl Pts',(3.76095021674888,2.26167018129524,4.35171973986433));
#19486=CARTESIAN_POINT('Ctrl Pts',(3.57106943112482,2.18973329268408,4.34060595080752));
#19487=CARTESIAN_POINT('Ctrl Pts',(3.40765744378577,2.31031125094527,4.32949216175072));
#19488=CARTESIAN_POINT('Ctrl Pts',(3.42032221420706,2.51287144446394,4.31837837269392));
#19489=CARTESIAN_POINT('Ctrl Pts',(3.5974005298242,2.61234201428399,4.30726458363711));
#19490=CARTESIAN_POINT('Ctrl Pts',(3.77696052684568,2.51699709329055,4.29615079458031));
#19491=CARTESIAN_POINT('Ctrl Pts',(3.78843875194939,2.38276609266138,4.28874160187577));
#19492=CARTESIAN_POINT('Ctrl Pts',(3.76451707405898,2.328060251512,4.2850370055235));
#19493=CARTESIAN_POINT('Ctrl Pts',(3.74664903694653,2.52472660865709,5.2149629944765));
#19494=CARTESIAN_POINT('Ctrl Pts',(3.78812360169505,2.47596231494597,5.21125839812423));
#19495=CARTESIAN_POINT('Ctrl Pts',(3.81784745404107,2.33461033882977,5.20384920541969));
#19496=CARTESIAN_POINT('Ctrl Pts',(3.66299267959241,2.1812041532484,5.19273541636289));
#19497=CARTESIAN_POINT('Ctrl Pts',(3.4504439300895,2.22856452067679,5.18162162730609));
#19498=CARTESIAN_POINT('Ctrl Pts',(3.3748056347362,2.43259819666406,5.17050783824928));
#19499=CARTESIAN_POINT('Ctrl Pts',(3.5052800629955,2.60691546471448,5.15939404919248));
#19500=CARTESIAN_POINT('Ctrl Pts',(3.72245784756665,2.5917802320391,5.14828026013567));
#19501=CARTESIAN_POINT('Ctrl Pts',(3.82754601587795,2.40113655048171,5.13716647107887));
#19502=CARTESIAN_POINT('Ctrl Pts',(3.72436001352691,2.2094375050414,5.12605268202206));
#19503=CARTESIAN_POINT('Ctrl Pts',(3.5073452421747,2.19216999569193,5.11493889296526));
#19504=CARTESIAN_POINT('Ctrl Pts',(3.37513874016143,2.36512788948001,5.10382510390846));
#19505=CARTESIAN_POINT('Ctrl Pts',(3.44875014022381,2.57000649743315,5.09271131485165));
#19506=CARTESIAN_POINT('Ctrl Pts',(3.660802331703,2.61927529353934,5.08159752579485));
#19507=CARTESIAN_POINT('Ctrl Pts',(3.81720141974412,2.46783939447801,5.07048373673805));
#19508=CARTESIAN_POINT('Ctrl Pts',(3.77479360487843,2.25430909472489,5.05936994768124));
#19509=CARTESIAN_POINT('Ctrl Pts',(3.57239521127782,2.17413144945252,5.04825615862444));
#19510=CARTESIAN_POINT('Ctrl Pts',(3.39526379879546,2.30069379177829,5.03714236956763));
#19511=CARTESIAN_POINT('Ctrl Pts',(3.40552975067466,2.51815226178119,5.02602858051083));
#19512=CARTESIAN_POINT('Ctrl Pts',(3.59379652843607,2.62746461211554,5.01491479145402));
#19513=CARTESIAN_POINT('Ctrl Pts',(3.78774141345684,2.52857603060814,5.00380100239722));
#19514=CARTESIAN_POINT('Ctrl Pts',(3.80984445391536,2.3120003465126,4.99268721334041));
#19515=CARTESIAN_POINT('Ctrl Pts',(3.63987448575377,2.17597174504624,4.98157342428361));
#19516=CARTESIAN_POINT('Ctrl Pts',(3.43340694865093,2.24499874508934,4.9704596352268));
#19517=CARTESIAN_POINT('Ctrl Pts',(3.37942392070334,2.45590015203683,4.95934584617001));
#19518=CARTESIAN_POINT('Ctrl Pts',(3.52733667965797,2.61563551564903,4.94823205711319));
#19519=CARTESIAN_POINT('Ctrl Pts',(3.74175899977021,2.57799724642702,4.9371182680564));
#19520=CARTESIAN_POINT('Ctrl Pts',(3.82642769974115,2.37743607886815,4.92600447899959));
#19521=CARTESIAN_POINT('Ctrl Pts',(3.70384455827186,2.19752792424157,4.91489068994279));
#19522=CARTESIAN_POINT('Ctrl Pts',(3.48621131494014,2.20294475673219,4.90377690088598));
#19523=CARTESIAN_POINT('Ctrl Pts',(3.37273014549458,2.38872848815129,4.89266311182918));
#19524=CARTESIAN_POINT('Ctrl Pts',(3.46727165129357,2.58482916218966,4.88154932277237));
#19525=CARTESIAN_POINT('Ctrl Pts',(3.68330091990526,2.61175360797231,4.87043553371557));
#19526=CARTESIAN_POINT('Ctrl Pts',(3.82308391183106,2.4448575749278,4.85932174465876));
#19527=CARTESIAN_POINT('Ctrl Pts',(3.75867566931422,2.2369028948328,4.84820795560196));
#19528=CARTESIAN_POINT('Ctrl Pts',(3.54902978716961,2.1782328447441,4.83709416654516));
#19529=CARTESIAN_POINT('Ctrl Pts',(3.38603751887018,2.32254878687183,4.82598037748835));
#19530=CARTESIAN_POINT('Ctrl Pts',(3.41888753604845,2.53775670273222,4.81486658843155));
#19531=CARTESIAN_POINT('Ctrl Pts',(3.61751184543661,2.62687434631457,4.80375279937474));
#19532=CARTESIAN_POINT('Ctrl Pts',(3.80010736409881,2.5083313277851,4.79263901031794));
#19533=CARTESIAN_POINT('Ctrl Pts',(3.79954234302951,2.29063141637312,4.78152522126113));
#19534=CARTESIAN_POINT('Ctrl Pts',(3.61633395242122,2.17303780987892,4.77041143220434));
#19535=CARTESIAN_POINT('Ctrl Pts',(3.41817490992216,2.26318526992884,4.75929764314752));
#19536=CARTESIAN_POINT('Ctrl Pts',(3.38644243440813,2.47856080399747,4.74818385409073));
#19537=CARTESIAN_POINT('Ctrl Pts',(3.55018162058784,2.62202874322709,4.73707006503392));
#19538=CARTESIAN_POINT('Ctrl Pts',(3.75952013442236,2.56227125580376,4.72595627597711));
#19539=CARTESIAN_POINT('Ctrl Pts',(3.82284806013872,2.35398504766203,4.71484248692031));
#19540=CARTESIAN_POINT('Ctrl Pts',(3.68220062914122,2.1878168472403,4.7037286978635));
#19541=CARTESIAN_POINT('Ctrl Pts',(3.46631403007222,2.21586229286015,4.6926149088067));
#19542=CARTESIAN_POINT('Ctrl Pts',(3.37279171538014,2.4124510700887,4.6815011197499));
#19543=CARTESIAN_POINT('Ctrl Pts',(3.48723572031781,2.59764324166039,4.67038733069309));
#19544=CARTESIAN_POINT('Ctrl Pts',(3.70489414928252,2.6019303127134,4.65927354163629));
#19545=CARTESIAN_POINT('Ctrl Pts',(3.82654177382834,2.42138827849455,4.64815975257948));
#19546=CARTESIAN_POINT('Ctrl Pts',(3.74083314363071,2.22126931040964,4.63704596352268));
#19547=CARTESIAN_POINT('Ctrl Pts',(3.52621833991124,2.18474456945152,4.62593217446588));
#19548=CARTESIAN_POINT('Ctrl Pts',(3.3791367264123,2.34524556523533,4.61481838540907));
#19549=CARTESIAN_POINT('Ctrl Pts',(3.43421377198734,2.55586391612019,4.60370459635226));
#19550=CARTESIAN_POINT('Ctrl Pts',(3.64103683220752,2.62381825695636,4.59259080729547));
#19551=CARTESIAN_POINT('Ctrl Pts',(3.81029841451592,2.48690920894243,4.58147701823866));
#19552=CARTESIAN_POINT('Ctrl Pts',(3.78707147307748,2.27045117633852,4.57036322918186));
#19553=CARTESIAN_POINT('Ctrl Pts',(3.59261589078479,2.17257065127066,4.55924944012505));
#19554=CARTESIAN_POINT('Ctrl Pts',(3.40491906742157,2.28285878820862,4.54813565106825));
#19555=CARTESIAN_POINT('Ctrl Pts',(3.39578203396899,2.500367604992,4.53702186201145));
#19556=CARTESIAN_POINT('Ctrl Pts',(3.57356802090726,2.62600881423741,4.52590807295463));
#19557=CARTESIAN_POINT('Ctrl Pts',(3.77554749788108,2.54478159358368,4.51479428389784));
#19558=CARTESIAN_POINT('Ctrl Pts',(3.81684635957493,2.33103413661225,4.50368049484102));
#19559=CARTESIAN_POINT('Ctrl Pts',(3.65966328839466,2.18041192008159,4.49256670578423));
#19560=CARTESIAN_POINT('Ctrl Pts',(3.44786973422143,2.23078115627741,4.48145291672742));
#19561=CARTESIAN_POINT('Ctrl Pts',(3.37532273458119,2.43603833346541,4.47033912767062));
#19562=CARTESIAN_POINT('Ctrl Pts',(3.50842539001751,2.60830918677142,4.45922533861381));
#19563=CARTESIAN_POINT('Ctrl Pts',(3.72534731243133,2.58991233623048,4.44811154955701));
#19564=CARTESIAN_POINT('Ctrl Pts',(3.82753744240543,2.39768645605247,4.4369977605002));
#19565=CARTESIAN_POINT('Ctrl Pts',(3.72145992250484,2.20757841825199,4.4258839714434));
#19566=CARTESIAN_POINT('Ctrl Pts',(3.50420885499455,2.19359557710565,4.41477018238659));
#19567=CARTESIAN_POINT('Ctrl Pts',(3.37463631478375,2.36853796487738,4.40365639332979));
#19568=CARTESIAN_POINT('Ctrl Pts',(3.45134210009517,2.57227606808331,4.39254260427299));
#19569=CARTESIAN_POINT('Ctrl Pts',(3.6641153687781,2.61833162147455,4.38142881521619));
#19570=CARTESIAN_POINT('Ctrl Pts',(3.81820467194806,2.46453837795421,4.37031502615938));
#19571=CARTESIAN_POINT('Ctrl Pts',(3.77256564288916,2.25168721995093,4.35920123710258));
#19572=CARTESIAN_POINT('Ctrl Pts',(3.56898157506129,2.17455880296967,4.34808744804577));
#19573=CARTESIAN_POINT('Ctrl Pts',(3.39377650096713,2.30383860952047,4.33697365898897));
#19574=CARTESIAN_POINT('Ctrl Pts',(3.40735526025023,2.52101713045927,4.32585986993216));
#19575=CARTESIAN_POINT('Ctrl Pts',(3.59721293173057,2.62766627437643,4.31474608087536));
#19576=CARTESIAN_POINT('Ctrl Pts',(3.78973138215013,2.52544051836443,4.30363229181856));
#19577=CARTESIAN_POINT('Ctrl Pts',(3.8020379657277,2.3815223591527,4.29622309911402));
#19578=CARTESIAN_POINT('Ctrl Pts',(3.77638991251267,2.32286851675083,4.29251850276175));
#19579=CARTESIAN_POINT('Ctrl Pts',(3.75652001142717,2.53312198033322,5.22244449171475));
#19580=CARTESIAN_POINT('Ctrl Pts',(3.80078623699225,2.48107535276698,5.21873989536248));
#19581=CARTESIAN_POINT('Ctrl Pts',(3.83251080747514,2.33020894833891,5.21133070265794));
#19582=CARTESIAN_POINT('Ctrl Pts',(3.6672327287988,2.16647696332117,5.20021691360114));
#19583=CARTESIAN_POINT('Ctrl Pts',(3.44037728266889,2.21702516606042,5.18910312454433));
#19584=CARTESIAN_POINT('Ctrl Pts',(3.3596477593148,2.43479238746194,5.17798933548753));
#19585=CARTESIAN_POINT('Ctrl Pts',(3.4989044460774,2.62084298387434,5.16687554643073));
#19586=CARTESIAN_POINT('Ctrl Pts',(3.73070050850364,2.60468899581803,5.15576175737391));
#19587=CARTESIAN_POINT('Ctrl Pts',(3.84286218134804,2.40121305191012,5.14464796831713));
#19588=CARTESIAN_POINT('Ctrl Pts',(3.73273070961532,2.19661070737624,5.1335341792603));
#19589=CARTESIAN_POINT('Ctrl Pts',(3.50110863285869,2.17818091869864,5.12242039020352));
#19590=CARTESIAN_POINT('Ctrl Pts',(3.36000328612935,2.36278064110937,5.1113066011467));
#19591=CARTESIAN_POINT('Ctrl Pts',(3.43856948348621,2.58144966700758,5.10019281208991));
#19592=CARTESIAN_POINT('Ctrl Pts',(3.66489494817768,2.63403475512075,5.08907902303309));
#19593=CARTESIAN_POINT('Ctrl Pts',(3.83182128848718,2.47240567698227,5.0779652339763));
#19594=CARTESIAN_POINT('Ctrl Pts',(3.78655899556261,2.24450261226871,5.06685144491949));
#19595=CARTESIAN_POINT('Ctrl Pts',(3.57053712771522,2.15892819449186,5.05573765586269));
#19596=CARTESIAN_POINT('Ctrl Pts',(3.38148296627563,2.29400947207503,5.04462386680588));
#19597=CARTESIAN_POINT('Ctrl Pts',(3.39243992132218,2.52610511292264,5.03351007774908));
#19598=CARTESIAN_POINT('Ctrl Pts',(3.59337897158896,2.64277529828296,5.02239628869227));
#19599=CARTESIAN_POINT('Ctrl Pts',(3.80037832359127,2.53723050760561,5.01128249963547));
#19600=CARTESIAN_POINT('Ctrl Pts',(3.82396912389365,2.30607707315216,5.00016871057866));
#19601=CARTESIAN_POINT('Ctrl Pts',(3.64255844494981,2.16089236073089,4.98905492152186));
#19602=CARTESIAN_POINT('Ctrl Pts',(3.42219353877959,2.234565581234,4.97794113246505));
#19603=CARTESIAN_POINT('Ctrl Pts',(3.36457690298599,2.45966280186876,4.96682734340826));
#19604=CARTESIAN_POINT('Ctrl Pts',(3.52244569778922,2.63014998309056,4.95571355435144));
#19605=CARTESIAN_POINT('Ctrl Pts',(3.7513008249214,2.58997827483123,4.94459976529465));
#19606=CARTESIAN_POINT('Ctrl Pts',(3.84166859114005,2.37591729705878,4.93348597623783));
#19607=CARTESIAN_POINT('Ctrl Pts',(3.71083435517744,2.18389949043478,4.92237218718104));
#19608=CARTESIAN_POINT('Ctrl Pts',(3.47855217697512,2.18968093094735,4.91125839812423));
#19609=CARTESIAN_POINT('Ctrl Pts',(3.35743256849882,2.38796980055174,4.90014460906743));
#19610=CARTESIAN_POINT('Ctrl Pts',(3.45833768097764,2.59727004813914,4.88903082001062));
#19611=CARTESIAN_POINT('Ctrl Pts',(3.68890792061744,2.62600678347214,4.87791703095382));
#19612=CARTESIAN_POINT('Ctrl Pts',(3.83809973223177,2.44787694680091,4.86680324189701));
#19613=CARTESIAN_POINT('Ctrl Pts',(3.76935615869971,2.22592479776177,4.85568945284022));
#19614=CARTESIAN_POINT('Ctrl Pts',(3.54559897248035,2.16330565547811,4.8445756637834));
#19615=CARTESIAN_POINT('Ctrl Pts',(3.37163566369933,2.31733553103189,4.83346187472661));
#19616=CARTESIAN_POINT('Ctrl Pts',(3.40669682176204,2.54702913251096,4.82234808566979));
#19617=CARTESIAN_POINT('Ctrl Pts',(3.61869057107309,2.64214530157901,4.811234296613));
#19618=CARTESIAN_POINT('Ctrl Pts',(3.81357662871545,2.51562312999728,4.80012050755618));
#19619=CARTESIAN_POINT('Ctrl Pts',(3.81297357597085,2.28326979627357,4.78900671849939));
#19620=CARTESIAN_POINT('Ctrl Pts',(3.61743339385551,2.1577609418312,4.77789292944258));
#19621=CARTESIAN_POINT('Ctrl Pts',(3.40593622863608,2.2539762445085,4.76677914038578));
#19622=CARTESIAN_POINT('Ctrl Pts',(3.37206783417891,2.48384874660919,4.75566535132897));
#19623=CARTESIAN_POINT('Ctrl Pts',(3.54682833602434,2.63697354002902,4.74455156227216));
#19624=CARTESIAN_POINT('Ctrl Pts',(3.77025746491439,2.57319376479756,4.73343777321537));
#19625=CARTESIAN_POINT('Ctrl Pts',(3.83784800531731,2.35088777249601,4.72232398415856));
#19626=CARTESIAN_POINT('Ctrl Pts',(3.68773356907346,2.1735347589994,4.71121019510175));
#19627=CARTESIAN_POINT('Ctrl Pts',(3.45731560209032,2.20346794888116,4.70009640604495));
#19628=CARTESIAN_POINT('Ctrl Pts',(3.35749828266505,2.41328915397702,4.68898261698814));
#19629=CARTESIAN_POINT('Ctrl Pts',(3.47964553527297,2.61094664572852,4.67786882793135));
#19630=CARTESIAN_POINT('Ctrl Pts',(3.71195459435803,2.61552228034691,4.66675503887453));
#19631=CARTESIAN_POINT('Ctrl Pts',(3.84179034357568,2.42282792757511,4.65564124981774));
#19632=CARTESIAN_POINT('Ctrl Pts',(3.75031264922961,2.20923891380705,4.64452746076093));
#19633=CARTESIAN_POINT('Ctrl Pts',(3.5212520823821,2.17025568561017,4.63341367170412));
#19634=CARTESIAN_POINT('Ctrl Pts',(3.36427037759277,2.34156003385021,4.62229988264733));
#19635=CARTESIAN_POINT('Ctrl Pts',(3.42305466954774,2.56635514586511,4.61118609359051));
#19636=CARTESIAN_POINT('Ctrl Pts',(3.64379902916374,2.63888350626668,4.60007230453372));
#19637=CARTESIAN_POINT('Ctrl Pts',(3.8244536406683,2.49275908427381,4.5889585154769));
#19638=CARTESIAN_POINT('Ctrl Pts',(3.79966328939795,2.26173122045618,4.57784472642011));
#19639=CARTESIAN_POINT('Ctrl Pts',(3.59211886499353,2.15726233868846,4.56673093736329));
#19640=CARTESIAN_POINT('Ctrl Pts',(3.39178813286355,2.27497399103367,4.55561714830651));
#19641=CARTESIAN_POINT('Ctrl Pts',(3.38203608395695,2.50712336751311,4.54450335924968));
#19642=CARTESIAN_POINT('Ctrl Pts',(3.57178887938318,2.64122151037363,4.5333895701929));
#19643=CARTESIAN_POINT('Ctrl Pts',(3.78736363324621,2.55452687009752,4.52227578113608));
#19644=CARTESIAN_POINT('Ctrl Pts',(3.83144232915068,2.3263920312721,4.51116199207928));
#19645=CARTESIAN_POINT('Ctrl Pts',(3.66367923564831,2.1656314047897,4.50004820302247));
#19646=CARTESIAN_POINT('Ctrl Pts',(3.43762981718889,2.21939100382357,4.48893441396567));
#19647=CARTESIAN_POINT('Ctrl Pts',(3.36019966524839,2.43846408052362,4.47782062490886));
#19648=CARTESIAN_POINT('Ctrl Pts',(3.5022614856576,2.62233051762717,4.46670683585207));
#19649=CARTESIAN_POINT('Ctrl Pts',(3.73378446379617,2.60269537158839,4.45559304679526));
#19650=CARTESIAN_POINT('Ctrl Pts',(3.84285303079348,2.39753073097072,4.44447925773845));
#19651=CARTESIAN_POINT('Ctrl Pts',(3.72963541291671,2.19462648510256,4.43336546868165));
#19652=CARTESIAN_POINT('Ctrl Pts',(3.49776113486282,2.17970245626759,4.42225167962485));
#19653=CARTESIAN_POINT('Ctrl Pts',(3.35946704240424,2.36642024932827,4.41113789056804));
#19654=CARTESIAN_POINT('Ctrl Pts',(3.44133590866794,2.5838720028885,4.40002410151124));
#19655=CARTESIAN_POINT('Ctrl Pts',(3.66843098640644,2.63302756431036,4.38891031245443));
#19656=CARTESIAN_POINT('Ctrl Pts',(3.83289206978718,2.4688824684104,4.37779652339763));
#19657=CARTESIAN_POINT('Ctrl Pts',(3.78418106902943,2.24170425860662,4.36668273434082));
#19658=CARTESIAN_POINT('Ctrl Pts',(3.56689371899776,2.15938431325527,4.35556894528402));
#19659=CARTESIAN_POINT('Ctrl Pts',(3.37989555814849,2.29736596809567,4.34445515622721));
#19660=CARTESIAN_POINT('Ctrl Pts',(3.39438830629339,2.5291628164546,4.33334136717041));
#19661=CARTESIAN_POINT('Ctrl Pts',(3.59702533363695,2.64299053446886,4.32222757811361));
#19662=CARTESIAN_POINT('Ctrl Pts',(3.80250223745458,2.5338839434383,4.3111137890568));
#19663=CARTESIAN_POINT('Ctrl Pts',(3.81563717950601,2.38027862564402,4.30370459635227));
#19664=CARTESIAN_POINT('Ctrl Pts',(3.78826275096636,2.31767678198967,4.3));
#19665=CARTESIAN_POINT('Ctrl Pts',(3.72690708798524,2.50793586530485,5.2));
#19666=CARTESIAN_POINT('Ctrl Pts',(3.7351188943469,2.50027512151453,5.2));
#19667=CARTESIAN_POINT('Ctrl Pts',(3.74243605781657,2.49177396851828,5.2));
#19668=CARTESIAN_POINT('Ctrl Pts',(3.74885415042291,2.48262661237479,5.2));
#19669=CARTESIAN_POINT('Ctrl Pts',(3.75362491760652,2.47582709900174,5.2));
#19670=CARTESIAN_POINT('Ctrl Pts',(3.75789857135109,2.46866923842676,5.2));
#19671=CARTESIAN_POINT('Ctrl Pts',(3.7616631109362,2.46121836915243,5.2));
#19672=CARTESIAN_POINT('Ctrl Pts',(3.76388040997986,2.45682983638691,5.2));
#19673=CARTESIAN_POINT('Ctrl Pts',(3.76592247954252,2.45233444011456,5.2));
#19674=CARTESIAN_POINT('Ctrl Pts',(3.76777440855395,2.44777396604178,5.2));
#19675=CARTESIAN_POINT('Ctrl Pts',(3.77233273486399,2.43654884411541,5.2));
#19676=CARTESIAN_POINT('Ctrl Pts',(3.77575805024602,2.42490557824884,5.2));
#19677=CARTESIAN_POINT('Ctrl Pts',(3.77802226640697,2.41304266545579,5.2));
#19678=CARTESIAN_POINT('Ctrl Pts',(3.7794611438358,2.4055039517268,5.2));
#19679=CARTESIAN_POINT('Ctrl Pts',(3.78043038990374,2.39787565429666,5.2));
#19680=CARTESIAN_POINT('Ctrl Pts',(3.78091323142362,2.39020359559663,5.2));
#19681=CARTESIAN_POINT('Ctrl Pts',(3.78113855699256,2.38662330906275,5.2));
#19682=CARTESIAN_POINT('Ctrl Pts',(3.78125741264451,2.38303694149785,5.2));
#19683=CARTESIAN_POINT('Ctrl Pts',(3.78126865224829,2.37945929304311,5.2));
#19684=CARTESIAN_POINT('Ctrl Pts',(3.7813036985799,2.36830378822358,5.2));
#19685=CARTESIAN_POINT('Ctrl Pts',(3.78029680360483,2.3572059009501,5.2));
#19686=CARTESIAN_POINT('Ctrl Pts',(3.77821424861763,2.34630678216484,5.2));
#19687=CARTESIAN_POINT('Ctrl Pts',(3.77705386628862,2.34023388376937,5.2));
#19688=CARTESIAN_POINT('Ctrl Pts',(3.77555898983988,2.33422245704814,5.2));
#19689=CARTESIAN_POINT('Ctrl Pts',(3.77374834890996,2.32828864283844,5.2));
#19690=CARTESIAN_POINT('Ctrl Pts',(3.7726157055599,2.32457675546527,5.2));
#19691=CARTESIAN_POINT('Ctrl Pts',(3.77135884755536,2.32089372066286,5.2));
#19692=CARTESIAN_POINT('Ctrl Pts',(3.76998347568685,2.31724835341447,5.2));
#19693=CARTESIAN_POINT('Ctrl Pts',(3.76560168937412,2.30563460684914,5.2));
#19694=CARTESIAN_POINT('Ctrl Pts',(3.76005258957863,2.29448378034876,5.2));
#19695=CARTESIAN_POINT('Ctrl Pts',(3.75350159415067,2.28391841534468,5.2));
#19696=CARTESIAN_POINT('Ctrl Pts',(3.74916061754095,2.27691734155978,5.2));
#19697=CARTESIAN_POINT('Ctrl Pts',(3.74437851970176,2.27017319623005,5.2));
#19698=CARTESIAN_POINT('Ctrl Pts',(3.73919188354146,2.26372385230471,5.2));
#19699=CARTESIAN_POINT('Ctrl Pts',(3.73648175856153,2.26035393632525,5.2));
#19700=CARTESIAN_POINT('Ctrl Pts',(3.73365978483958,2.25706319070089,5.2));
#19701=CARTESIAN_POINT('Ctrl Pts',(3.73073434111394,2.25386182215374,5.2));
#19702=CARTESIAN_POINT('Ctrl Pts',(3.72446791350779,2.24700435158764,5.2));
#19703=CARTESIAN_POINT('Ctrl Pts',(3.71775194552741,2.24058263588329,5.2));
#19704=CARTESIAN_POINT('Ctrl Pts',(3.71064052052299,2.23464742809312,5.2));
#19705=CARTESIAN_POINT('Ctrl Pts',(3.70611387191905,2.23086947922341,5.2));
#19706=CARTESIAN_POINT('Ctrl Pts',(3.70142674452504,2.22728872352275,5.2));
#19707=CARTESIAN_POINT('Ctrl Pts',(3.69659089091882,2.22391966825811,5.2));
#19708=CARTESIAN_POINT('Ctrl Pts',(3.69251851777989,2.22108251658222,5.2));
#19709=CARTESIAN_POINT('Ctrl Pts',(3.68834767342073,2.21840053637087,5.2));
#19710=CARTESIAN_POINT('Ctrl Pts',(3.68408917108174,2.21588334611703,5.2));
#19711=CARTESIAN_POINT('Ctrl Pts',(3.67536611602187,2.21072716973562,5.2));
#19712=CARTESIAN_POINT('Ctrl Pts',(3.66627202526677,2.20625880103906,5.2));
#19713=CARTESIAN_POINT('Ctrl Pts',(3.65686566645047,2.20255201748434,5.2));
#19714=CARTESIAN_POINT('Ctrl Pts',(3.65562635833217,2.2020636407339,5.2));
#19715=CARTESIAN_POINT('Ctrl Pts',(3.65438161447105,2.20158850411268,5.2));
#19716=CARTESIAN_POINT('Ctrl Pts',(3.65313162618094,2.20112654952031,5.2));
#19717=CARTESIAN_POINT('Ctrl Pts',(3.43326717741735,2.39986996798437,5.08714803633902));
#19718=CARTESIAN_POINT('Ctrl Pts',(3.43319402496042,2.39134538728232,5.08771939403666));
#19719=CARTESIAN_POINT('Ctrl Pts',(3.43379133263065,2.38283109195966,5.08829075173431));
#19720=CARTESIAN_POINT('Ctrl Pts',(3.43509475123467,2.374426308808,5.08886210943196));
#19721=CARTESIAN_POINT('Ctrl Pts',(3.44354591908595,2.31993097404037,5.09256670578422));
#19722=CARTESIAN_POINT('Ctrl Pts',(3.48168218994633,2.27003956185944,5.0962713021365));
#19723=CARTESIAN_POINT('Ctrl Pts',(3.53205035213375,2.24758434755118,5.09997589848876));
#19724=CARTESIAN_POINT('Ctrl Pts',(3.58241851432117,2.22512913324292,5.10368049484103));
#19725=CARTESIAN_POINT('Ctrl Pts',(3.64501856783563,2.23011011680733,5.1073850911933));
#19726=CARTESIAN_POINT('Ctrl Pts',(3.69120110519081,2.26024934979839,5.11108968754557));
#19727=CARTESIAN_POINT('Ctrl Pts',(3.73738364254598,2.29038858278945,5.11479428389783));
#19728=CARTESIAN_POINT('Ctrl Pts',(3.76714866374187,2.34568606520718,5.1184988802501));
#19729=CARTESIAN_POINT('Ctrl Pts',(3.76687431446563,2.40083133255876,5.12220347660237));
#19730=CARTESIAN_POINT('Ctrl Pts',(3.7665999651894,2.45597659991035,5.12590807295464));
#19731=CARTESIAN_POINT('Ctrl Pts',(3.73628624544104,2.51096965219579,5.12961266930691));
#19732=CARTESIAN_POINT('Ctrl Pts',(3.68980584742337,2.54064913199077,5.13331726565917));
#19733=CARTESIAN_POINT('Ctrl Pts',(3.6433254494057,2.57032861178575,5.13702186201144));
#19734=CARTESIAN_POINT('Ctrl Pts',(3.5806783731187,2.57469451909026,5.14072645836371));
#19735=CARTESIAN_POINT('Ctrl Pts',(3.53053651643308,2.5517357041881,5.14443105471598));
#19736=CARTESIAN_POINT('Ctrl Pts',(3.48039465974747,2.52877688928595,5.14813565106825));
#19737=CARTESIAN_POINT('Ctrl Pts',(3.44275802266323,2.47849335217712,5.15184024742051));
#19738=CARTESIAN_POINT('Ctrl Pts',(3.43484901067973,2.42392381942959,5.15554484377278));
#19739=CARTESIAN_POINT('Ctrl Pts',(3.43370811542309,2.41605202441919,5.15607924129486));
#19740=CARTESIAN_POINT('Ctrl Pts',(3.43318581643692,2.40809104297335,5.15661363881694));
#19741=CARTESIAN_POINT('Ctrl Pts',(3.43325215340634,2.40012157034435,5.15714803633902));
#19742=CARTESIAN_POINT('Ctrl Pts',(3.54698297828114,2.20148256743283,5.2));
#19743=CARTESIAN_POINT('Ctrl Pts',(3.48097120902544,2.21911198848201,5.19629540364773));
#19744=CARTESIAN_POINT('Ctrl Pts',(3.36906718698604,2.32515231990061,5.1888862109432));
#19745=CARTESIAN_POINT('Ctrl Pts',(3.41187706889408,2.55382793971174,5.17777242188639));
#19746=CARTESIAN_POINT('Ctrl Pts',(3.62721323264599,2.64128528195604,5.16665863282959));
#19747=CARTESIAN_POINT('Ctrl Pts',(3.81747536314189,2.50809334538988,5.15554484377278));
#19748=CARTESIAN_POINT('Ctrl Pts',(3.80876232811303,2.27586209318291,5.14443105471598));
#19749=CARTESIAN_POINT('Ctrl Pts',(3.60892557137656,2.15730570431671,5.13331726565918));
#19750=CARTESIAN_POINT('Ctrl Pts',(3.40093971248811,2.26086517215761,5.12220347660237));
#19751=CARTESIAN_POINT('Ctrl Pts',(3.37514571617861,2.4917888042929,5.11108968754557));
#19752=CARTESIAN_POINT('Ctrl Pts',(3.55516852834243,2.63869087044012,5.09997589848876));
#19753=CARTESIAN_POINT('Ctrl Pts',(3.77622353148193,2.56711958879047,5.08886210943196));
#19754=CARTESIAN_POINT('Ctrl Pts',(3.8359804180852,2.34258029751366,5.07774832037515));
#19755=CARTESIAN_POINT('Ctrl Pts',(3.6797411123384,2.17059868763558,5.06663453131835));
#19756=CARTESIAN_POINT('Ctrl Pts',(3.45051418153466,2.2085903127083,5.05552074226155));
#19757=CARTESIAN_POINT('Ctrl Pts',(3.3581131561336,2.4217815890047,5.04440695320474));
#19758=CARTESIAN_POINT('Ctrl Pts',(3.48711398178203,2.61503583311392,5.03329316414794));
#19759=CARTESIAN_POINT('Ctrl Pts',(3.71944062032543,2.61146538882495,5.02217937509113));
#19760=CARTESIAN_POINT('Ctrl Pts',(3.84244192441188,2.41433825182845,5.01106558603433));
#19761=CARTESIAN_POINT('Ctrl Pts',(3.74353337567863,2.20408716238119,4.99995179697753));
#19762=CARTESIAN_POINT('Ctrl Pts',(3.51324710536571,2.17315730898832,4.98883800792072));
#19763=CARTESIAN_POINT('Ctrl Pts',(3.36236674087989,2.34985914625667,4.97772421886392));
#19764=CARTESIAN_POINT('Ctrl Pts',(3.42899479464802,2.5724554740903,4.96661042980711));
#19765=CARTESIAN_POINT('Ctrl Pts',(3.652145851588,2.63720135146115,4.95549664075031));
#19766=CARTESIAN_POINT('Ctrl Pts',(3.82756721950384,2.48483414141864,4.9443828516935));
#19767=CARTESIAN_POINT('Ctrl Pts',(3.79469373046592,2.25481727983819,4.9332690626367));
#19768=CARTESIAN_POINT('Ctrl Pts',(3.58361486203243,2.15768780841241,4.9221552735799));
#19769=CARTESIAN_POINT('Ctrl Pts',(3.38753349616232,2.28234943400059,4.91104148452309));
#19770=CARTESIAN_POINT('Ctrl Pts',(3.38592513080807,2.51469795687288,4.89992769546629));
#19771=CARTESIAN_POINT('Ctrl Pts',(3.58026192098975,2.64206213906777,4.88881390640948));
#19772=CARTESIAN_POINT('Ctrl Pts',(3.79266519873933,2.54786410019675,4.87770011735268));
#19773=CARTESIAN_POINT('Ctrl Pts',(3.82871983510845,2.3183243735256,4.86658632829587));
#19774=CARTESIAN_POINT('Ctrl Pts',(3.65542461254465,2.16354327402962,4.85547253923907));
#19775=CARTESIAN_POINT('Ctrl Pts',(3.43139861356028,2.22519369741672,4.84435875018226));
#19776=CARTESIAN_POINT('Ctrl Pts',(3.36169537565425,2.44684631199623,4.83324496112547));
#19777=CARTESIAN_POINT('Ctrl Pts',(3.51011506296999,2.62561996593247,4.82213117206865));
#19778=CARTESIAN_POINT('Ctrl Pts',(3.74080745251389,2.59788110634618,4.81101738301186));
#19779=CARTESIAN_POINT('Ctrl Pts',(3.84261718390667,2.38901942599691,4.79990359395504));
#19780=CARTESIAN_POINT('Ctrl Pts',(3.72235665540369,2.19020838956081,4.78878980489825));
#19781=CARTESIAN_POINT('Ctrl Pts',(3.49010169259086,2.18342199335841,4.77767601584144));
#19782=CARTESIAN_POINT('Ctrl Pts',(3.35843789688119,2.37487190279669,4.76656222678464));
#19783=CARTESIAN_POINT('Ctrl Pts',(3.44787863365674,2.58932184457717,4.75544843772783));
#19784=CARTESIAN_POINT('Ctrl Pts',(3.67655778221991,2.63048335496042,4.74433464867103));
#19785=CARTESIAN_POINT('Ctrl Pts',(3.8351627244929,2.46068083668937,4.73322085961423));
#19786=CARTESIAN_POINT('Ctrl Pts',(3.77852055811084,2.23533646042905,4.72210707055742));
#19787=CARTESIAN_POINT('Ctrl Pts',(3.55847650032912,2.16071048934957,4.71099328150062));
#19788=CARTESIAN_POINT('Ctrl Pts',(3.37643937270466,2.30510892109605,4.69987949244382));
#19789=CARTESIAN_POINT('Ctrl Pts',(3.39902982259358,2.53636223350135,4.68876570338701));
#19790=CARTESIAN_POINT('Ctrl Pts',(3.60557055501943,2.64280164712995,4.67765191433021));
#19791=CARTESIAN_POINT('Ctrl Pts',(3.80701249526159,2.52700195958257,4.6665381252734));
#19792=CARTESIAN_POINT('Ctrl Pts',(3.81897355090948,2.29495593812904,4.65542433621659));
#19793=CARTESIAN_POINT('Ctrl Pts',(3.63050563208088,2.15905793778677,4.6443105471598));
#19794=CARTESIAN_POINT('Ctrl Pts',(3.41411556225142,2.24369693945694,4.63319675810298));
#19795=CARTESIAN_POINT('Ctrl Pts',(3.3678676263658,2.47140190503977,4.62208296904619));
#19796=CARTESIAN_POINT('Ctrl Pts',(3.53409308462842,2.63375189718637,4.61096917998938));
#19797=CARTESIAN_POINT('Ctrl Pts',(3.76064388996454,2.58214612691277,4.59985539093257));
#19798=CARTESIAN_POINT('Ctrl Pts',(3.84015552099323,2.36381994099575,4.58874160187577));
#19799=CARTESIAN_POINT('Ctrl Pts',(3.6998500801025,2.17860977340027,4.57762781281896));
#19800=CARTESIAN_POINT('Ctrl Pts',(3.46815072852799,2.1960405909371,4.56651402376216));
#19801=CARTESIAN_POINT('Ctrl Pts',(3.3571345103823,2.40015776866696,4.55540023470536));
#19802=CARTESIAN_POINT('Ctrl Pts',(3.46841582920963,2.6041305389052,4.54428644564855));
#19803=CARTESIAN_POINT('Ctrl Pts',(3.70013763173937,2.6212603119689,4.53317265659175));
#19804=CARTESIAN_POINT('Ctrl Pts',(3.84020232447629,2.43586801205837,4.52205886753494));
#19805=CARTESIAN_POINT('Ctrl Pts',(3.76040710518764,2.21764531427324,4.51094507847815));
#19806=CARTESIAN_POINT('Ctrl Pts',(3.53378944408678,2.16633392770918,4.49983128942133));
#19807=CARTESIAN_POINT('Ctrl Pts',(3.36777505427786,2.32889974840269,4.48871750036454));
#19808=CARTESIAN_POINT('Ctrl Pts',(3.4143187937299,2.55654443303944,4.47760371130772));
#19809=CARTESIAN_POINT('Ctrl Pts',(3.63081864137997,2.64090222813732,4.46648992225093));
#19810=CARTESIAN_POINT('Ctrl Pts',(3.81910984841827,2.50475947107891,4.45537613319412));
#19811=CARTESIAN_POINT('Ctrl Pts',(3.80684730359907,2.27272920356226,4.44426234413732));
#19812=CARTESIAN_POINT('Ctrl Pts',(3.60525512148808,2.15719129638054,4.43314855508051));
#19813=CARTESIAN_POINT('Ctrl Pts',(3.39885277598246,2.26389903533996,4.42203476602371));
#19814=CARTESIAN_POINT('Ctrl Pts',(3.3765629481812,2.49518135839549,4.4109209769669));
#19815=CARTESIAN_POINT('Ctrl Pts',(3.55878722266986,2.63934344974957,4.3998071879101));
#19816=CARTESIAN_POINT('Ctrl Pts',(3.77873475080197,2.56443107632444,4.38869339885329));
#19817=CARTESIAN_POINT('Ctrl Pts',(3.8350828706128,2.33901445723046,4.37757960979649));
#19818=CARTESIAN_POINT('Ctrl Pts',(3.67625990394949,2.16941582752504,4.36646582073968));
#19819=CARTESIAN_POINT('Ctrl Pts',(3.44762951395987,2.21087905095695,4.35535203168288));
#19820=CARTESIAN_POINT('Ctrl Pts',(3.35847730739013,2.42543572165447,4.34423824262608));
#19821=CARTESIAN_POINT('Ctrl Pts',(3.49037003538787,2.61673301642169,4.33312445356927));
#19822=CARTESIAN_POINT('Ctrl Pts',(3.72265542052987,2.60960761604941,4.32201066451248));
#19823=CARTESIAN_POINT('Ctrl Pts',(3.84257850979074,2.41071512516748,4.31089687545566));
#19824=CARTESIAN_POINT('Ctrl Pts',(3.7406568756376,2.20183613957205,4.29978308639887));
#19825=CARTESIAN_POINT('Ctrl Pts',(3.50959639242813,2.17470169312488,4.28866929734205));
#19826=CARTESIAN_POINT('Ctrl Pts',(3.41142456563631,2.29356865430551,4.28126010463752));
#19827=CARTESIAN_POINT('Ctrl Pts',(3.39833241385534,2.360627924571,4.27755550828525));
#19828=CARTESIAN_POINT('Ctrl Pts',(3.55032651029123,2.21400211999972,5.20748149723825));
#19829=CARTESIAN_POINT('Ctrl Pts',(3.48847779011663,2.2305197371096,5.20377690088598));
#19830=CARTESIAN_POINT('Ctrl Pts',(3.38363102379655,2.32987260795489,5.19636770818144));
#19831=CARTESIAN_POINT('Ctrl Pts',(3.42374108957258,2.54412674142112,5.18525391912464));
#19832=CARTESIAN_POINT('Ctrl Pts',(3.62549702318155,2.62606856404868,5.17414013006783));
#19833=CARTESIAN_POINT('Ctrl Pts',(3.8037602238433,2.50127641096634,5.16302634101103));
#19834=CARTESIAN_POINT('Ctrl Pts',(3.79559667859298,2.28369088196908,5.15191255195422));
#19835=CARTESIAN_POINT('Ctrl Pts',(3.60836267793897,2.1726112820345,5.14079876289743));
#19836=CARTESIAN_POINT('Ctrl Pts',(3.41349350034069,2.269639745597,5.12968497384062));
#19837=CARTESIAN_POINT('Ctrl Pts',(3.38932620899373,2.48600011991624,5.11857118478381));
#19838=CARTESIAN_POINT('Ctrl Pts',(3.55799583654811,2.62363776975738,5.10745739572701));
#19839=CARTESIAN_POINT('Ctrl Pts',(3.76510994947867,2.55658014925731,5.0963436066702));
#19840=CARTESIAN_POINT('Ctrl Pts',(3.82109825277221,2.34620148571036,5.08522981761341));
#19841=CARTESIAN_POINT('Ctrl Pts',(3.67471221873066,2.18506593996663,5.0741160285566));
#19842=CARTESIAN_POINT('Ctrl Pts',(3.45994154284032,2.22066161350478,5.0630022394998));
#19843=CARTESIAN_POINT('Ctrl Pts',(3.37336781169642,2.42040792753322,5.05188845044299));
#19844=CARTESIAN_POINT('Ctrl Pts',(3.49423316734106,2.60147454339935,5.04077466138619));
#19845=CARTESIAN_POINT('Ctrl Pts',(3.71190806711109,2.59812927009101,5.02966087232938));
#19846=CARTESIAN_POINT('Ctrl Pts',(3.82715226255275,2.41343400631629,5.01854708327258));
#19847=CARTESIAN_POINT('Ctrl Pts',(3.73448140669699,2.21644245550271,5.00743329421577));
#19848=CARTESIAN_POINT('Ctrl Pts',(3.51871819881407,2.18746320121053,4.99631950515897));
#19849=CARTESIAN_POINT('Ctrl Pts',(3.37735314303472,2.35302129199909,4.98520571610216));
#19850=CARTESIAN_POINT('Ctrl Pts',(3.43977928158165,2.56157952558844,4.97409192704536));
#19851=CARTESIAN_POINT('Ctrl Pts',(3.64885726014462,2.62224218767309,4.96297813798855));
#19852=CARTESIAN_POINT('Ctrl Pts',(3.81321563470729,2.47948405463168,4.95186434893176));
#19853=CARTESIAN_POINT('Ctrl Pts',(3.78241532064824,2.26397326515074,4.94075055987495));
#19854=CARTESIAN_POINT('Ctrl Pts',(3.58464819494153,2.17296928863785,4.92963677081815));
#19855=CARTESIAN_POINT('Ctrl Pts',(3.40093275047013,2.28976909698186,4.91852298176134));
#19856=CARTESIAN_POINT('Ctrl Pts',(3.39942581708757,2.50746450093999,4.90740919270454));
#19857=CARTESIAN_POINT('Ctrl Pts',(3.58150670798172,2.62679642846834,4.89629540364773));
#19858=CARTESIAN_POINT('Ctrl Pts',(3.78051471879288,2.53853901296773,4.88518161459093));
#19859=CARTESIAN_POINT('Ctrl Pts',(3.81429556031454,2.32347526776122,4.87406782553412));
#19860=CARTESIAN_POINT('Ctrl Pts',(3.65192924520447,2.17845547782099,4.86295403647733));
#19861=CARTESIAN_POINT('Ctrl Pts',(3.4420315030405,2.23621790151766,4.85184024742051));
#19862=CARTESIAN_POINT('Ctrl Pts',(3.37672411762845,2.4438919373702,4.84072645836372));
#19863=CARTESIAN_POINT('Ctrl Pts',(3.51578367947165,2.61139118517954,4.8296126693069));
#19864=CARTESIAN_POINT('Ctrl Pts',(3.73192739457257,2.58540168385487,4.81849888025011));
#19865=CARTESIAN_POINT('Ctrl Pts',(3.82731646926276,2.38971191869978,4.8073850911933));
#19866=CARTESIAN_POINT('Ctrl Pts',(3.71464020169267,2.20343895103354,4.7962713021365));
#19867=CARTESIAN_POINT('Ctrl Pts',(3.49703245740495,2.19708054064022,4.78515751307969));
#19868=CARTESIAN_POINT('Ctrl Pts',(3.37367207258585,2.37645661266209,4.77404372402289));
#19869=CARTESIAN_POINT('Ctrl Pts',(3.45747220646219,2.57738221411453,4.76292993496608));
#19870=CARTESIAN_POINT('Ctrl Pts',(3.6717296461388,2.6159478633368,4.75181614590928));
#19871=CARTESIAN_POINT('Ctrl Pts',(3.82033212723505,2.45685398423157,4.74070235685248));
#19872=CARTESIAN_POINT('Ctrl Pts',(3.7672621135368,2.24572100859114,4.72958856779567));
#19873=CARTESIAN_POINT('Ctrl Pts',(3.56109519043692,2.17580134343001,4.71847477873887));
#19874=CARTESIAN_POINT('Ctrl Pts',(3.39053828074069,2.31109325121307,4.70736098968206));
#19875=CARTESIAN_POINT('Ctrl Pts',(3.41170405813995,2.52776251443194,4.69624720062526));
#19876=CARTESIAN_POINT('Ctrl Pts',(3.60521924654496,2.62748929926577,4.68513341156846));
#19877=CARTESIAN_POINT('Ctrl Pts',(3.79395719939706,2.51899254857754,4.67401962251165));
#19878=CARTESIAN_POINT('Ctrl Pts',(3.80516392801682,2.30158056870897,4.66290583345484));
#19879=CARTESIAN_POINT('Ctrl Pts',(3.62858178660552,2.17425301045342,4.65179204439804));
#19880=CARTESIAN_POINT('Ctrl Pts',(3.42583841177484,2.25355423187469,4.64067825534123));
#19881=CARTESIAN_POINT('Ctrl Pts',(3.38250711377307,2.46689892566933,4.62956446628444));
#19882=CARTESIAN_POINT('Ctrl Pts',(3.53824952107254,2.61901027411281,4.61845067722762));
#19883=CARTESIAN_POINT('Ctrl Pts',(3.7505128420311,2.57065903491661,4.60733688817083));
#19884=CARTESIAN_POINT('Ctrl Pts',(3.82501005174943,2.36610164565372,4.59622309911402));
#19885=CARTESIAN_POINT('Ctrl Pts',(3.69355300930883,2.19257180456232,4.58510931005721));
#19886=CARTESIAN_POINT('Ctrl Pts',(3.47646583649485,2.20890334314105,4.57399552100041));
#19887=CARTESIAN_POINT('Ctrl Pts',(3.37245088448926,2.4001478189457,4.5628817319436));
#19888=CARTESIAN_POINT('Ctrl Pts',(3.47671421853432,2.59125699435405,4.55176794288681));
#19889=CARTESIAN_POINT('Ctrl Pts',(3.69382242642831,2.60730647390622,4.54065415382999));
#19890=CARTESIAN_POINT('Ctrl Pts',(3.82505390355888,2.43360598672071,4.5295403647732));
#19891=CARTESIAN_POINT('Ctrl Pts',(3.75029099014661,2.22914555908425,4.51842657571639));
#19892=CARTESIAN_POINT('Ctrl Pts',(3.53796502969918,2.18107013821379,4.50731278665959));
#19893=CARTESIAN_POINT('Ctrl Pts',(3.3824203797675,2.33338370392177,4.49619899760278));
#19894=CARTESIAN_POINT('Ctrl Pts',(3.42602882640825,2.54667191840358,4.48508520854598));
#19895=CARTESIAN_POINT('Ctrl Pts',(3.62887505589326,2.62570966761684,4.47397141948917));
#19896=CARTESIAN_POINT('Ctrl Pts',(3.80529162988842,2.49815278828994,4.46285763043237));
#19897=CARTESIAN_POINT('Ctrl Pts',(3.79380242558891,2.28075556883219,4.45174384137556));
#19898=CARTESIAN_POINT('Ctrl Pts',(3.60492370590979,2.17250408926403,4.44063005231877));
#19899=CARTESIAN_POINT('Ctrl Pts',(3.41153817701856,2.2724822774232,4.42951626326195));
#19900=CARTESIAN_POINT('Ctrl Pts',(3.39065406289825,2.48917872172821,4.41840247420516));
#19901=CARTESIAN_POINT('Ctrl Pts',(3.56138631699392,2.62424919398607,4.40728868514835));
#19902=CARTESIAN_POINT('Ctrl Pts',(3.76746279811117,2.55406118851634,4.39617489609155));
#19903=CARTESIAN_POINT('Ctrl Pts',(3.82025730936029,2.342860526055,4.38506110703474));
#19904=CARTESIAN_POINT('Ctrl Pts',(3.67145055363756,2.18395767723095,4.37394731797794));
#19905=CARTESIAN_POINT('Ctrl Pts',(3.4572387975626,2.22280601189145,4.36283352892113));
#19906=CARTESIAN_POINT('Ctrl Pts',(3.37370899766098,2.42383161137452,4.35171973986432));
#19907=CARTESIAN_POINT('Ctrl Pts',(3.49728387709496,2.60306469340852,4.34060595080753));
#19908=CARTESIAN_POINT('Ctrl Pts',(3.71492012511989,2.59638865822985,4.32949216175072));
#19909=CARTESIAN_POINT('Ctrl Pts',(3.82728023413982,2.4100393730632,4.31837837269392));
#19910=CARTESIAN_POINT('Ctrl Pts',(3.73178631386543,2.21433339402172,4.30726458363711));
#19911=CARTESIAN_POINT('Ctrl Pts',(3.51529771901994,2.18891018836724,4.29615079458031));
#19912=CARTESIAN_POINT('Ctrl Pts',(3.42331712354828,2.30028077429395,4.28874160187577));
#19913=CARTESIAN_POINT('Ctrl Pts',(3.41105063166184,2.36311093455973,4.2850370055235));
#19914=CARTESIAN_POINT('Ctrl Pts',(3.55367004230132,2.22652167256662,5.2149629944765));
#19915=CARTESIAN_POINT('Ctrl Pts',(3.49598437120782,2.24192748573719,5.21125839812423));
#19916=CARTESIAN_POINT('Ctrl Pts',(3.39819486060706,2.33459289600918,5.20384920541969));
#19917=CARTESIAN_POINT('Ctrl Pts',(3.43560511025108,2.5344255431305,5.19273541636289));
#19918=CARTESIAN_POINT('Ctrl Pts',(3.62378081371712,2.61085184614133,5.18162162730608));
#19919=CARTESIAN_POINT('Ctrl Pts',(3.79004508454469,2.4944594765428,5.17050783824928));
#19920=CARTESIAN_POINT('Ctrl Pts',(3.78243102907294,2.29151967075525,5.15939404919247));
#19921=CARTESIAN_POINT('Ctrl Pts',(3.60779978450139,2.18791685975229,5.14828026013568));
#19922=CARTESIAN_POINT('Ctrl Pts',(3.42604728819327,2.27841431903638,5.13716647107886));
#19923=CARTESIAN_POINT('Ctrl Pts',(3.40350670180884,2.48021143553957,5.12605268202207));
#19924=CARTESIAN_POINT('Ctrl Pts',(3.56082314475379,2.60858466907463,5.11493889296526));
#19925=CARTESIAN_POINT('Ctrl Pts',(3.75399636747541,2.54604070972415,5.10382510390846));
#19926=CARTESIAN_POINT('Ctrl Pts',(3.80621608745921,2.34982267390707,5.09271131485165));
#19927=CARTESIAN_POINT('Ctrl Pts',(3.66968332512291,2.19953319229768,5.08159752579485));
#19928=CARTESIAN_POINT('Ctrl Pts',(3.46936890414598,2.23273291430124,5.07048373673804));
#19929=CARTESIAN_POINT('Ctrl Pts',(3.38862246725923,2.41903426606174,5.05936994768124));
#19930=CARTESIAN_POINT('Ctrl Pts',(3.50135235290009,2.58791325368478,5.04825615862443));
#19931=CARTESIAN_POINT('Ctrl Pts',(3.70437551389675,2.58479315135706,5.03714236956764));
#19932=CARTESIAN_POINT('Ctrl Pts',(3.81186260069363,2.41252976080414,5.02602858051082));
#19933=CARTESIAN_POINT('Ctrl Pts',(3.72542943771535,2.22879774862422,5.01491479145403));
#19934=CARTESIAN_POINT('Ctrl Pts',(3.52418929226243,2.20176909343275,5.00380100239722));
#19935=CARTESIAN_POINT('Ctrl Pts',(3.39233954518956,2.35618343774151,4.99268721334042));
#19936=CARTESIAN_POINT('Ctrl Pts',(3.45056376851527,2.55070357708658,4.98157342428361));
#19937=CARTESIAN_POINT('Ctrl Pts',(3.64556866870124,2.60728302388504,4.9704596352268));
#19938=CARTESIAN_POINT('Ctrl Pts',(3.79886404991074,2.47413396784473,4.95934584617));
#19939=CARTESIAN_POINT('Ctrl Pts',(3.77013691083056,2.27312925046329,4.9482320571132));
#19940=CARTESIAN_POINT('Ctrl Pts',(3.58568152785062,2.18825076886329,4.93711826805639));
#19941=CARTESIAN_POINT('Ctrl Pts',(3.41433200477794,2.29718875996312,4.92600447899959));
#19942=CARTESIAN_POINT('Ctrl Pts',(3.41292650336706,2.5002310450071,4.91489068994278));
#19943=CARTESIAN_POINT('Ctrl Pts',(3.58275149497368,2.61153071786889,4.90377690088598));
#19944=CARTESIAN_POINT('Ctrl Pts',(3.76836423884643,2.52921392573871,4.89266311182918));
#19945=CARTESIAN_POINT('Ctrl Pts',(3.79987128552062,2.32862616199684,4.88154932277237));
#19946=CARTESIAN_POINT('Ctrl Pts',(3.64843387786428,2.19336768161237,4.87043553371557));
#19947=CARTESIAN_POINT('Ctrl Pts',(3.45266439252072,2.24724210561861,4.85932174465876));
#19948=CARTESIAN_POINT('Ctrl Pts',(3.39175285960263,2.44093756274417,4.84820795560197));
#19949=CARTESIAN_POINT('Ctrl Pts',(3.52145229597333,2.59716240442661,4.83709416654515));
#19950=CARTESIAN_POINT('Ctrl Pts',(3.72304733663125,2.57292226136356,4.82598037748836));
#19951=CARTESIAN_POINT('Ctrl Pts',(3.81201575461885,2.39040441140265,4.81486658843155));
#19952=CARTESIAN_POINT('Ctrl Pts',(3.70692374798164,2.21666951250626,4.80375279937475));
#19953=CARTESIAN_POINT('Ctrl Pts',(3.50396322221905,2.21073908792203,4.79263901031794));
#19954=CARTESIAN_POINT('Ctrl Pts',(3.3889062482905,2.37804132252749,4.78152522126113));
#19955=CARTESIAN_POINT('Ctrl Pts',(3.46706577926762,2.56544258365188,4.77041143220433));
#19956=CARTESIAN_POINT('Ctrl Pts',(3.66690151005769,2.60141237171319,4.75929764314753));
#19957=CARTESIAN_POINT('Ctrl Pts',(3.80550152997722,2.45302713177377,4.74818385409072));
#19958=CARTESIAN_POINT('Ctrl Pts',(3.75600366896275,2.25610555675324,4.73707006503392));
#19959=CARTESIAN_POINT('Ctrl Pts',(3.56371388054473,2.19089219751045,4.72595627597711));
#19960=CARTESIAN_POINT('Ctrl Pts',(3.40463718877671,2.31707758133011,4.71484248692031));
#19961=CARTESIAN_POINT('Ctrl Pts',(3.42437829368633,2.51916279536252,4.7037286978635));
#19962=CARTESIAN_POINT('Ctrl Pts',(3.60486793807048,2.61217695140159,4.69261490880671));
#19963=CARTESIAN_POINT('Ctrl Pts',(3.78090190353252,2.51098313757252,4.6815011197499));
#19964=CARTESIAN_POINT('Ctrl Pts',(3.79135430512417,2.3082051992889,4.67038733069309));
#19965=CARTESIAN_POINT('Ctrl Pts',(3.62665794113017,2.18944808312007,4.65927354163629));
#19966=CARTESIAN_POINT('Ctrl Pts',(3.43756126129826,2.26341152429244,4.64815975257949));
#19967=CARTESIAN_POINT('Ctrl Pts',(3.39714660118035,2.46239594629889,4.63704596352268));
#19968=CARTESIAN_POINT('Ctrl Pts',(3.54240595751667,2.60426865103925,4.62593217446588));
#19969=CARTESIAN_POINT('Ctrl Pts',(3.74038179409766,2.55917194292045,4.61481838540907));
#19970=CARTESIAN_POINT('Ctrl Pts',(3.80986458250562,2.36838335031169,4.60370459635227));
#19971=CARTESIAN_POINT('Ctrl Pts',(3.68725593851517,2.20653383572437,4.59259080729547));
#19972=CARTESIAN_POINT('Ctrl Pts',(3.48478094446172,2.221766095345,4.58147701823866));
#19973=CARTESIAN_POINT('Ctrl Pts',(3.38776725859624,2.40013786922444,4.57036322918186));
#19974=CARTESIAN_POINT('Ctrl Pts',(3.48501260785902,2.57838344980291,4.55924944012505));
#19975=CARTESIAN_POINT('Ctrl Pts',(3.68750722111726,2.59335263584353,4.54813565106824));
#19976=CARTESIAN_POINT('Ctrl Pts',(3.80990548264146,2.43134396138305,4.53702186201145));
#19977=CARTESIAN_POINT('Ctrl Pts',(3.74017487510557,2.24064580389526,4.52590807295464));
#19978=CARTESIAN_POINT('Ctrl Pts',(3.54214061531159,2.19580634871841,4.51479428389784));
#19979=CARTESIAN_POINT('Ctrl Pts',(3.39706570525713,2.33786765944084,4.50368049484103));
#19980=CARTESIAN_POINT('Ctrl Pts',(3.4377388590866,2.53679940376773,4.49256670578423));
#19981=CARTESIAN_POINT('Ctrl Pts',(3.62693147040654,2.61051710709635,4.48145291672742));
#19982=CARTESIAN_POINT('Ctrl Pts',(3.79147341135858,2.49154610550097,4.47033912767062));
#19983=CARTESIAN_POINT('Ctrl Pts',(3.78075754757875,2.28878193410212,4.45922533861381));
#19984=CARTESIAN_POINT('Ctrl Pts',(3.60459229033149,2.18781688214753,4.44811154955701));
#19985=CARTESIAN_POINT('Ctrl Pts',(3.42422357805467,2.28106551950643,4.43699776050021));
#19986=CARTESIAN_POINT('Ctrl Pts',(3.4047451776153,2.48317608506094,4.4258839714434));
#19987=CARTESIAN_POINT('Ctrl Pts',(3.56398541131798,2.60915493822257,4.4147701823866));
#19988=CARTESIAN_POINT('Ctrl Pts',(3.75619084542037,2.54369130070823,4.40365639332979));
#19989=CARTESIAN_POINT('Ctrl Pts',(3.80543174810779,2.34670659487954,4.39254260427299));
#19990=CARTESIAN_POINT('Ctrl Pts',(3.66664120332562,2.19849952693685,4.38142881521618));
#19991=CARTESIAN_POINT('Ctrl Pts',(3.46684808116532,2.23473297282595,4.37031502615938));
#19992=CARTESIAN_POINT('Ctrl Pts',(3.38894068793183,2.42222750109457,4.35920123710257));
#19993=CARTESIAN_POINT('Ctrl Pts',(3.50419771880206,2.58939637039535,4.34808744804578));
#19994=CARTESIAN_POINT('Ctrl Pts',(3.70718482970991,2.5831697004103,4.33697365898896));
#19995=CARTESIAN_POINT('Ctrl Pts',(3.81198195848891,2.40936362095891,4.32585986993217));
#19996=CARTESIAN_POINT('Ctrl Pts',(3.72291575209325,2.22683064847139,4.31474608087536));
#19997=CARTESIAN_POINT('Ctrl Pts',(3.52099904561175,2.2031186836096,4.30363229181856));
#19998=CARTESIAN_POINT('Ctrl Pts',(3.43520968146025,2.30699289428239,4.29622309911402));
#19999=CARTESIAN_POINT('Ctrl Pts',(3.42376884946835,2.36559394454846,4.29251850276175));
#20000=CARTESIAN_POINT('Ctrl Pts',(3.55701357431141,2.23904122513352,5.22244449171475));
#20001=CARTESIAN_POINT('Ctrl Pts',(3.50349095229901,2.25333523436478,5.21873989536248));
#20002=CARTESIAN_POINT('Ctrl Pts',(3.41275869741756,2.33931318406347,5.21133070265794));
#20003=CARTESIAN_POINT('Ctrl Pts',(3.44746913092958,2.52472434483988,5.20021691360114));
#20004=CARTESIAN_POINT('Ctrl Pts',(3.62206460425269,2.59563512823397,5.18910312454433));
#20005=CARTESIAN_POINT('Ctrl Pts',(3.77632994524609,2.48764254211926,5.17798933548754));
#20006=CARTESIAN_POINT('Ctrl Pts',(3.76926537955289,2.29934845954141,5.16687554643072));
#20007=CARTESIAN_POINT('Ctrl Pts',(3.60723689106381,2.20322243747008,5.15576175737393));
#20008=CARTESIAN_POINT('Ctrl Pts',(3.43860107604584,2.28718889247577,5.14464796831712));
#20009=CARTESIAN_POINT('Ctrl Pts',(3.41768719462395,2.47442275116291,5.13353417926031));
#20010=CARTESIAN_POINT('Ctrl Pts',(3.56365045295948,2.59353156839189,5.12242039020351));
#20011=CARTESIAN_POINT('Ctrl Pts',(3.74288278547214,2.53550127019098,5.1113066011467));
#20012=CARTESIAN_POINT('Ctrl Pts',(3.79133392214622,2.35344386210378,5.1001928120899));
#20013=CARTESIAN_POINT('Ctrl Pts',(3.66465443151516,2.21400044462873,5.0890790230331));
#20014=CARTESIAN_POINT('Ctrl Pts',(3.47879626545164,2.24480421509772,5.0779652339763));
#20015=CARTESIAN_POINT('Ctrl Pts',(3.40387712282204,2.41766060459026,5.06685144491948));
#20016=CARTESIAN_POINT('Ctrl Pts',(3.50847153845911,2.57435196397021,5.05573765586269));
#20017=CARTESIAN_POINT('Ctrl Pts',(3.69684296068241,2.57145703262312,5.04462386680587));
#20018=CARTESIAN_POINT('Ctrl Pts',(3.7965729388345,2.41162551529198,5.03351007774909));
#20019=CARTESIAN_POINT('Ctrl Pts',(3.71637746873371,2.24115304174574,5.02239628869227));
#20020=CARTESIAN_POINT('Ctrl Pts',(3.5296603857108,2.21607498565497,5.01128249963547));
#20021=CARTESIAN_POINT('Ctrl Pts',(3.40732594734439,2.35934558348393,5.00016871057866));
#20022=CARTESIAN_POINT('Ctrl Pts',(3.46134825544889,2.53982762858472,4.98905492152187));
#20023=CARTESIAN_POINT('Ctrl Pts',(3.64228007725786,2.59232386009698,4.97794113246505));
#20024=CARTESIAN_POINT('Ctrl Pts',(3.7845124651142,2.46878388105777,4.96682734340826));
#20025=CARTESIAN_POINT('Ctrl Pts',(3.75785850101288,2.28228523577585,4.95571355435144));
#20026=CARTESIAN_POINT('Ctrl Pts',(3.58671486075972,2.20353224908873,4.94459976529465));
#20027=CARTESIAN_POINT('Ctrl Pts',(3.42773125908574,2.30460842294439,4.93348597623783));
#20028=CARTESIAN_POINT('Ctrl Pts',(3.42642718964655,2.4929975890742,4.92237218718104));
#20029=CARTESIAN_POINT('Ctrl Pts',(3.58399628196565,2.59626500726946,4.91125839812423));
#20030=CARTESIAN_POINT('Ctrl Pts',(3.75621375889998,2.51988883850969,4.90014460906743));
#20031=CARTESIAN_POINT('Ctrl Pts',(3.7854470107267,2.33377705623246,4.88903082001062));
#20032=CARTESIAN_POINT('Ctrl Pts',(3.6449385105241,2.20827988540375,4.87791703095382));
#20033=CARTESIAN_POINT('Ctrl Pts',(3.46329728200094,2.25826630971955,4.86680324189701));
#20034=CARTESIAN_POINT('Ctrl Pts',(3.40678160157682,2.43798318811813,4.85568945284022));
#20035=CARTESIAN_POINT('Ctrl Pts',(3.527120912475,2.58293362367368,4.8445756637834));
#20036=CARTESIAN_POINT('Ctrl Pts',(3.71416727868993,2.56044283887224,4.8334618747266));
#20037=CARTESIAN_POINT('Ctrl Pts',(3.79671503997494,2.39109690410553,4.82234808566979));
#20038=CARTESIAN_POINT('Ctrl Pts',(3.69920729427062,2.22990007397898,4.811234296613));
#20039=CARTESIAN_POINT('Ctrl Pts',(3.51089398703315,2.22439763520385,4.80012050755619));
#20040=CARTESIAN_POINT('Ctrl Pts',(3.40414042399517,2.37962603239289,4.78900671849938));
#20041=CARTESIAN_POINT('Ctrl Pts',(3.47665935207306,2.55350295318923,4.77789292944258));
#20042=CARTESIAN_POINT('Ctrl Pts',(3.66207337397658,2.58687688008957,4.76677914038578));
#20043=CARTESIAN_POINT('Ctrl Pts',(3.79067093271938,2.44920027931597,4.75566535132897));
#20044=CARTESIAN_POINT('Ctrl Pts',(3.7447452243887,2.26649010491534,4.74455156227217));
#20045=CARTESIAN_POINT('Ctrl Pts',(3.56633257065254,2.20598305159089,4.73343777321536));
#20046=CARTESIAN_POINT('Ctrl Pts',(3.41873609681274,2.32306191144714,4.72232398415856));
#20047=CARTESIAN_POINT('Ctrl Pts',(3.4370525292327,2.5105630762931,4.71121019510175));
#20048=CARTESIAN_POINT('Ctrl Pts',(3.604516629596,2.59686460353741,4.70009640604495));
#20049=CARTESIAN_POINT('Ctrl Pts',(3.76784660766799,2.50297372656749,4.68898261698814));
#20050=CARTESIAN_POINT('Ctrl Pts',(3.77754468223151,2.31482982986883,4.67786882793134));
#20051=CARTESIAN_POINT('Ctrl Pts',(3.62473409565482,2.20464315578672,4.66675503887454));
#20052=CARTESIAN_POINT('Ctrl Pts',(3.44928411082169,2.27326881671019,4.65564124981774));
#20053=CARTESIAN_POINT('Ctrl Pts',(3.41178608858762,2.45789296692846,4.64452746076093));
#20054=CARTESIAN_POINT('Ctrl Pts',(3.5465623939608,2.58952702796569,4.63341367170412));
#20055=CARTESIAN_POINT('Ctrl Pts',(3.73025074616421,2.54768485092428,4.62229988264732));
#20056=CARTESIAN_POINT('Ctrl Pts',(3.79471911326182,2.37066505496967,4.61118609359052));
#20057=CARTESIAN_POINT('Ctrl Pts',(3.6809588677215,2.22049586688641,4.60007230453371));
#20058=CARTESIAN_POINT('Ctrl Pts',(3.49309605242859,2.23462884754895,4.58895851547691));
#20059=CARTESIAN_POINT('Ctrl Pts',(3.4030836327032,2.40012791950318,4.5778447264201));
#20060=CARTESIAN_POINT('Ctrl Pts',(3.49331099718372,2.56550990525176,4.56673093736331));
#20061=CARTESIAN_POINT('Ctrl Pts',(3.6811920158062,2.57939879778085,4.55561714830649));
#20062=CARTESIAN_POINT('Ctrl Pts',(3.79475706172405,2.42908193604538,4.5445033592497));
#20063=CARTESIAN_POINT('Ctrl Pts',(3.73005876006454,2.25214604870627,4.53338957019289));
#20064=CARTESIAN_POINT('Ctrl Pts',(3.54631620092399,2.21054255922302,4.52227578113609));
#20065=CARTESIAN_POINT('Ctrl Pts',(3.41171103074677,2.34235161495991,4.51116199207928));
#20066=CARTESIAN_POINT('Ctrl Pts',(3.44944889176494,2.52692688913187,4.50004820302248));
#20067=CARTESIAN_POINT('Ctrl Pts',(3.62498788491984,2.59532454657587,4.48893441396567));
#20068=CARTESIAN_POINT('Ctrl Pts',(3.77765519282873,2.484939422712,4.47782062490886));
#20069=CARTESIAN_POINT('Ctrl Pts',(3.76771266956859,2.29680829937205,4.46670683585207));
#20070=CARTESIAN_POINT('Ctrl Pts',(3.6042608747532,2.20312967503102,4.45559304679526));
#20071=CARTESIAN_POINT('Ctrl Pts',(3.43690897909078,2.28964876158967,4.44447925773845));
#20072=CARTESIAN_POINT('Ctrl Pts',(3.41883629233234,2.47717344839367,4.43336546868165));
#20073=CARTESIAN_POINT('Ctrl Pts',(3.56658450564204,2.59406068245907,4.42225167962485));
#20074=CARTESIAN_POINT('Ctrl Pts',(3.74491889272957,2.53332141290012,4.41113789056804));
#20075=CARTESIAN_POINT('Ctrl Pts',(3.7906061868553,2.35055266370407,4.40002410151124));
#20076=CARTESIAN_POINT('Ctrl Pts',(3.66183185301368,2.21304137664276,4.38891031245443));
#20077=CARTESIAN_POINT('Ctrl Pts',(3.47645736476805,2.24665993376045,4.37779652339763));
#20078=CARTESIAN_POINT('Ctrl Pts',(3.40417237820268,2.42062339081462,4.36668273434083));
#20079=CARTESIAN_POINT('Ctrl Pts',(3.51111156050916,2.57572804738218,4.35556894528402));
#20080=CARTESIAN_POINT('Ctrl Pts',(3.69944953429992,2.56995074259074,4.34445515622722));
#20081=CARTESIAN_POINT('Ctrl Pts',(3.796683682838,2.40868786885462,4.33334136717041));
#20082=CARTESIAN_POINT('Ctrl Pts',(3.71404519032108,2.23932790292106,4.32222757811361));
#20083=CARTESIAN_POINT('Ctrl Pts',(3.52670037220356,2.21732717885196,4.3111137890568));
#20084=CARTESIAN_POINT('Ctrl Pts',(3.44710223937223,2.31370501427082,4.30370459635227));
#20085=CARTESIAN_POINT('Ctrl Pts',(3.43648706727485,2.36807695453719,4.3));
#20086=CARTESIAN_POINT('Ctrl Pts',(3.43361558566414,2.40009421455432,5.13785196366098));
#20087=CARTESIAN_POINT('Ctrl Pts',(3.43350387426567,2.42168271797136,5.13641270219409));
#20088=CARTESIAN_POINT('Ctrl Pts',(3.43740295903752,2.4432325339629,5.1349734407272));
#20089=CARTESIAN_POINT('Ctrl Pts',(3.44550005125019,2.46306857758655,5.13353417926031));
#20090=CARTESIAN_POINT('Ctrl Pts',(3.46634161406913,2.51412569023923,5.12982958290805));
#20091=CARTESIAN_POINT('Ctrl Pts',(3.5149960335143,2.55382862931556,5.12612498655578));
#20092=CARTESIAN_POINT('Ctrl Pts',(3.56919529865567,2.56400838248691,5.12242039020351));
#20093=CARTESIAN_POINT('Ctrl Pts',(3.62339456379703,2.57418813565826,5.11871579385124));
#20094=CARTESIAN_POINT('Ctrl Pts',(3.68313867463459,2.55484470292462,5.11501119749897));
#20095=CARTESIAN_POINT('Ctrl Pts',(3.72108591949905,2.51483008520994,5.1113066011467));
#20096=CARTESIAN_POINT('Ctrl Pts',(3.7590331643635,2.47481546749525,5.10760200479444));
#20097=CARTESIAN_POINT('Ctrl Pts',(3.77518354325486,2.41412966479952,5.10389740844217));
#20098=CARTESIAN_POINT('Ctrl Pts',(3.76214548426203,2.36054619387247,5.1001928120899));
#20099=CARTESIAN_POINT('Ctrl Pts',(3.7491074252692,2.30696272294543,5.09648821573763));
#20100=CARTESIAN_POINT('Ctrl Pts',(3.70688092839218,2.26048158378708,5.09278361938537));
#20101=CARTESIAN_POINT('Ctrl Pts',(3.65479131894308,2.24237497595273,5.0890790230331));
#20102=CARTESIAN_POINT('Ctrl Pts',(3.60270170949399,2.22426836811839,5.08537442668083));
#20103=CARTESIAN_POINT('Ctrl Pts',(3.54074898747281,2.23453629160805,5.08166983032856));
#20104=CARTESIAN_POINT('Ctrl Pts',(3.49728610269062,2.26847965160164,5.0779652339763));
#20105=CARTESIAN_POINT('Ctrl Pts',(3.45773596364813,2.29936726097326,5.07459414387119));
#20106=CARTESIAN_POINT('Ctrl Pts',(3.43349641790554,2.34985942255505,5.07122305376608));
#20107=CARTESIAN_POINT('Ctrl Pts',(3.43317938608394,2.40008640134203,5.06785196366098));
#20108=CARTESIAN_POINT('Ctrl Pts',(3.54698297828114,2.20148256743283,5.2));
#20109=CARTESIAN_POINT('Ctrl Pts',(3.5345795220974,2.20607510740599,5.2));
#20110=CARTESIAN_POINT('Ctrl Pts',(3.52273022202852,2.21193437307052,5.2));
#20111=CARTESIAN_POINT('Ctrl Pts',(3.51155282869243,2.21889712518446,5.2));
#20112=CARTESIAN_POINT('Ctrl Pts',(3.50588663673039,2.22242677551307,5.2));
#20113=CARTESIAN_POINT('Ctrl Pts',(3.50039354941666,2.2262407482932,5.2));
#20114=CARTESIAN_POINT('Ctrl Pts',(3.49509234222245,2.23032135431632,5.2));
#20115=CARTESIAN_POINT('Ctrl Pts',(3.49050523644823,2.2338522805309,5.2));
#20116=CARTESIAN_POINT('Ctrl Pts',(3.48606182302158,2.23758289719759,5.2));
#20117=CARTESIAN_POINT('Ctrl Pts',(3.48177607353762,2.24150262969935,5.2));
#20118=CARTESIAN_POINT('Ctrl Pts',(3.4786657164721,2.24434735212827,5.2));
#20119=CARTESIAN_POINT('Ctrl Pts',(3.47564458925343,2.24728626535177,5.2));
#20120=CARTESIAN_POINT('Ctrl Pts',(3.47272209234032,2.25030915184069,5.2));
#20121=CARTESIAN_POINT('Ctrl Pts',(3.4637771038367,2.25956140622969,5.2));
#20122=CARTESIAN_POINT('Ctrl Pts',(3.45573639448352,2.26961351156597,5.2));
#20123=CARTESIAN_POINT('Ctrl Pts',(3.44873900472013,2.28033442966861,5.2));
#20124=CARTESIAN_POINT('Ctrl Pts',(3.44420815653473,2.28727628284152,5.2));
#20125=CARTESIAN_POINT('Ctrl Pts',(3.44011557094646,2.29449912284867,5.2));
#20126=CARTESIAN_POINT('Ctrl Pts',(3.43651072814608,2.30197002765831,5.2));
#20127=CARTESIAN_POINT('Ctrl Pts',(3.43484397915084,2.30542430396786,5.2));
#20128=CARTESIAN_POINT('Ctrl Pts',(3.43328563163244,2.30892352292903,5.2));
#20129=CARTESIAN_POINT('Ctrl Pts',(3.43184081732517,2.31246073059787,5.2));
#20130=CARTESIAN_POINT('Ctrl Pts',(3.42783869836044,2.3222587550377,5.2));
#20131=CARTESIAN_POINT('Ctrl Pts',(3.42470154623616,2.33235626573064,5.2));
#20132=CARTESIAN_POINT('Ctrl Pts',(3.42252347569321,2.34267987754179,5.2));
#20133=CARTESIAN_POINT('Ctrl Pts',(3.42066968522458,2.35146646769115,5.2));
#20134=CARTESIAN_POINT('Ctrl Pts',(3.41951139095334,2.36041732716722,5.2));
#20135=CARTESIAN_POINT('Ctrl Pts',(3.41903596356978,2.36945415649734,5.2));
#20136=CARTESIAN_POINT('Ctrl Pts',(3.41886682155969,2.37266917424891,5.2));
#20137=CARTESIAN_POINT('Ctrl Pts',(3.41878447232058,2.37589363434567,5.2));
#20138=CARTESIAN_POINT('Ctrl Pts',(3.41878798568376,2.3791143017356,5.2));
#20139=CARTESIAN_POINT('Ctrl Pts',(3.41880075844281,2.39082297128446,5.2));
#20140=CARTESIAN_POINT('Ctrl Pts',(3.41994282155898,2.40251786108517,5.2));
#20141=CARTESIAN_POINT('Ctrl Pts',(3.42216878897262,2.41402665747967,5.2));
#20142=CARTESIAN_POINT('Ctrl Pts',(3.42331180168116,2.41993631296624,5.2));
#20143=CARTESIAN_POINT('Ctrl Pts',(3.42474130312271,2.42579671745434,5.2));
#20144=CARTESIAN_POINT('Ctrl Pts',(3.4264550762976,2.43158227576526,5.2));
#20145=CARTESIAN_POINT('Ctrl Pts',(3.42814231216907,2.43727824630656,5.2));
#20146=CARTESIAN_POINT('Ctrl Pts',(3.43010783958643,2.44290710782216,5.2));
#20147=CARTESIAN_POINT('Ctrl Pts',(3.43233768577066,2.4484115412056,5.2));
#20148=CARTESIAN_POINT('Ctrl Pts',(3.43579440729991,2.4569445483329,5.2));
#20149=CARTESIAN_POINT('Ctrl Pts',(3.43988798414899,2.46519216359733,5.2));
#20150=CARTESIAN_POINT('Ctrl Pts',(3.44460907372922,2.4730585225122,5.2));
#20151=CARTESIAN_POINT('Ctrl Pts',(3.44702309019998,2.47708079738387,5.2));
#20152=CARTESIAN_POINT('Ctrl Pts',(3.44960209705083,2.48100348334585,5.2));
#20153=CARTESIAN_POINT('Ctrl Pts',(3.45233605468006,2.48480007154667,5.2));
#20154=CARTESIAN_POINT('Ctrl Pts',(3.45777065901345,2.49234698978257,5.2));
#20155=CARTESIAN_POINT('Ctrl Pts',(3.46382415870923,2.499410402925,5.2));
#20156=CARTESIAN_POINT('Ctrl Pts',(3.47049190322584,2.5058791831385,5.2));
#20157=CARTESIAN_POINT('Ctrl Pts',(3.47127037259775,2.50663442312367,5.2));
#20158=CARTESIAN_POINT('Ctrl Pts',(3.47205722899383,2.5073815321984,5.2));
#20159=CARTESIAN_POINT('Ctrl Pts',(3.47285231527688,2.50812044463164,5.2));
#20160=CARTESIAN_POINT('Origin',(3.6,2.4,4.7));
#20161=CARTESIAN_POINT('Origin',(3.6,-2.4,4.3));
#20162=CARTESIAN_POINT('Ctrl Pts',(3.43648706727485,-2.43192304546281,4.3));
#20163=CARTESIAN_POINT('Ctrl Pts',(3.43713128683253,-2.44021936733391,4.3));
#20164=CARTESIAN_POINT('Ctrl Pts',(3.43844438912273,-2.44842976439641,4.3));
#20165=CARTESIAN_POINT('Ctrl Pts',(3.44036779101517,-2.45650290183658,4.3));
#20166=CARTESIAN_POINT('Ctrl Pts',(3.44142971550231,-2.46096014104879,4.3));
#20167=CARTESIAN_POINT('Ctrl Pts',(3.44267796071139,-2.46537560589173,4.3));
#20168=CARTESIAN_POINT('Ctrl Pts',(3.44410466214797,-2.4697408265362,4.3));
#20169=CARTESIAN_POINT('Ctrl Pts',(3.44564437628146,-2.47445182755564,4.3));
#20170=CARTESIAN_POINT('Ctrl Pts',(3.44738954450943,-2.47909640503965,4.3));
#20171=CARTESIAN_POINT('Ctrl Pts',(3.44932653760859,-2.48365784749895,4.3));
#20172=CARTESIAN_POINT('Ctrl Pts',(3.45254730792056,-2.49124246845553,4.3));
#20173=CARTESIAN_POINT('Ctrl Pts',(3.45629958145885,-2.49860290469935,4.3));
#20174=CARTESIAN_POINT('Ctrl Pts',(3.460540361967,-2.50569093557372,4.3));
#20175=CARTESIAN_POINT('Ctrl Pts',(3.46239352486579,-2.50878830781843,4.3));
#20176=CARTESIAN_POINT('Ctrl Pts',(3.46433983439221,-2.51183274422802,4.3));
#20177=CARTESIAN_POINT('Ctrl Pts',(3.46636982169588,-2.5148117549636,4.3));
#20178=CARTESIAN_POINT('Ctrl Pts',(3.4732458122516,-2.52490228589753,4.3));
#20179=CARTESIAN_POINT('Ctrl Pts',(3.48109363537456,-2.5342702737356,4.3));
#20180=CARTESIAN_POINT('Ctrl Pts',(3.4897794934809,-2.54276723354547,4.3));
#20181=CARTESIAN_POINT('Ctrl Pts',(3.49400930325249,-2.54690505426423,4.3));
#20182=CARTESIAN_POINT('Ctrl Pts',(3.49843862851918,-2.55083612678489,4.3));
#20183=CARTESIAN_POINT('Ctrl Pts',(3.50305595405548,-2.55454125034048,4.3));
#20184=CARTESIAN_POINT('Ctrl Pts',(3.50696190635494,-2.55767554004086,4.3));
#20185=CARTESIAN_POINT('Ctrl Pts',(3.51100694759131,-2.56065060854479,4.3));
#20186=CARTESIAN_POINT('Ctrl Pts',(3.51515869554757,-2.56343734237232,4.3));
#20187=CARTESIAN_POINT('Ctrl Pts',(3.52023397904373,-2.56684397118314,4.3));
#20188=CARTESIAN_POINT('Ctrl Pts',(3.52547419237578,-2.56997446151731,4.3));
#20189=CARTESIAN_POINT('Ctrl Pts',(3.53086407609141,-2.57281069688687,4.3));
#20190=CARTESIAN_POINT('Ctrl Pts',(3.53843716228638,-2.57679576522158,4.3));
#20191=CARTESIAN_POINT('Ctrl Pts',(3.5463054085634,-2.58020053156405,4.3));
#20192=CARTESIAN_POINT('Ctrl Pts',(3.55440202217605,-2.58304072456499,4.3));
#20193=CARTESIAN_POINT('Ctrl Pts',(3.56031216163472,-2.58511392918216,4.3));
#20194=CARTESIAN_POINT('Ctrl Pts',(3.5663442123363,-2.58688610080112,4.3));
#20195=CARTESIAN_POINT('Ctrl Pts',(3.57247443059928,-2.58835971156752,4.3));
#20196=CARTESIAN_POINT('Ctrl Pts',(3.57600236806727,-2.58920777380822,4.3));
#20197=CARTESIAN_POINT('Ctrl Pts',(3.57955832823423,-2.58995565186198,4.3));
#20198=CARTESIAN_POINT('Ctrl Pts',(3.58312950627136,-2.59060308036101,4.3));
#20199=CARTESIAN_POINT('Ctrl Pts',(3.59464642713376,-2.59269101400921,4.3));
#20200=CARTESIAN_POINT('Ctrl Pts',(3.6063444588111,-2.59374267077427,4.3));
#20201=CARTESIAN_POINT('Ctrl Pts',(3.61806681517941,-2.59379134323091,4.3));
#20202=CARTESIAN_POINT('Ctrl Pts',(3.62473112824741,-2.59381901415975,4.3));
#20203=CARTESIAN_POINT('Ctrl Pts',(3.63140369181744,-2.59352192189353,4.3));
#20204=CARTESIAN_POINT('Ctrl Pts',(3.63805736597901,-2.59290136699938,4.3));
#20205=CARTESIAN_POINT('Ctrl Pts',(3.64215429545284,-2.59251926688834,4.3));
#20206=CARTESIAN_POINT('Ctrl Pts',(3.64624613464129,-2.59201413768455,4.3));
#20207=CARTESIAN_POINT('Ctrl Pts',(3.65032004640889,-2.59138662655135,4.3));
#20208=CARTESIAN_POINT('Ctrl Pts',(3.6635759835922,-2.58934479338508,4.3));
#20209=CARTESIAN_POINT('Ctrl Pts',(3.67655554403262,-2.58602558677096,4.3));
#20210=CARTESIAN_POINT('Ctrl Pts',(3.68904453335804,-2.58146163637399,4.3));
#20211=CARTESIAN_POINT('Ctrl Pts',(3.69937751045428,-2.5776855746214,4.3));
#20212=CARTESIAN_POINT('Ctrl Pts',(3.70937567296629,-2.57305657585047,4.3));
#20213=CARTESIAN_POINT('Ctrl Pts',(3.7189159065364,-2.56756614624894,4.3));
#20214=CARTESIAN_POINT('Ctrl Pts',(3.72007018633274,-2.56690185517936,4.3));
#20215=CARTESIAN_POINT('Ctrl Pts',(3.72121775119647,-2.56622492375,4.3));
#20216=CARTESIAN_POINT('Ctrl Pts',(3.72235852099786,-2.56553552032368,4.3));
#20217=CARTESIAN_POINT('Ctrl Pts',(3.78826275096637,-2.48232321801033,4.3));
#20218=CARTESIAN_POINT('Ctrl Pts',(3.79091867325729,-2.4742706313139,4.3));
#20219=CARTESIAN_POINT('Ctrl Pts',(3.79302804122654,-2.46606039506531,4.3));
#20220=CARTESIAN_POINT('Ctrl Pts',(3.79460324133206,-2.45774386615892,4.3));
#20221=CARTESIAN_POINT('Ctrl Pts',(3.79578956705146,-2.45148046374845,4.3));
#20222=CARTESIAN_POINT('Ctrl Pts',(3.79667272255332,-2.44515671383718,4.3));
#20223=CARTESIAN_POINT('Ctrl Pts',(3.79725488779627,-2.43879482378833,4.3));
#20224=CARTESIAN_POINT('Ctrl Pts',(3.79769087373759,-2.43403037820329,4.3));
#20225=CARTESIAN_POINT('Ctrl Pts',(3.79795758751143,-2.42924591021267,4.3));
#20226=CARTESIAN_POINT('Ctrl Pts',(3.79805591662036,-2.4244630110418,4.3));
#20227=CARTESIAN_POINT('Ctrl Pts',(3.79826160078478,-2.41445817493456,4.3));
#20228=CARTESIAN_POINT('Ctrl Pts',(3.79773307923007,-2.40444525216584,4.3));
#20229=CARTESIAN_POINT('Ctrl Pts',(3.7964780509907,-2.39451257334247,4.3));
#20230=CARTESIAN_POINT('Ctrl Pts',(3.79582248849211,-2.38932425044823,4.3));
#20231=CARTESIAN_POINT('Ctrl Pts',(3.7949674129287,-2.38415491083777,4.3));
#20232=CARTESIAN_POINT('Ctrl Pts',(3.79391844712734,-2.37904222861684,4.3));
#20233=CARTESIAN_POINT('Ctrl Pts',(3.79135149974265,-2.3665308710123,4.3));
#20234=CARTESIAN_POINT('Ctrl Pts',(3.78762424888679,-2.35432630792998,4.3));
#20235=CARTESIAN_POINT('Ctrl Pts',(3.78275036269461,-2.34261709433331,4.3));
#20236=CARTESIAN_POINT('Ctrl Pts',(3.78051279286925,-2.33724146962858,4.3));
#20237=CARTESIAN_POINT('Ctrl Pts',(3.77803293300414,-2.33197059787363,4.3));
#20238=CARTESIAN_POINT('Ctrl Pts',(3.77530918258224,-2.32682518237142,4.3));
#20239=CARTESIAN_POINT('Ctrl Pts',(3.77352855433059,-2.32346141154425,4.3));
#20240=CARTESIAN_POINT('Ctrl Pts',(3.77164258388613,-2.32014955771335,4.3));
#20241=CARTESIAN_POINT('Ctrl Pts',(3.76965386637616,-2.31690144569075,4.3));
#20242=CARTESIAN_POINT('Ctrl Pts',(3.76538144816038,-2.30992343453397,4.3));
#20243=CARTESIAN_POINT('Ctrl Pts',(3.76065257819642,-2.3032660772289,4.3));
#20244=CARTESIAN_POINT('Ctrl Pts',(3.7554693784929,-2.29698171698016,4.3));
#20245=CARTESIAN_POINT('Ctrl Pts',(3.74976402854315,-2.29006427669614,4.3));
#20246=CARTESIAN_POINT('Ctrl Pts',(3.74350800901797,-2.28359846633093,4.3));
#20247=CARTESIAN_POINT('Ctrl Pts',(3.73677358655615,-2.27761728545388,4.3));
#20248=CARTESIAN_POINT('Ctrl Pts',(3.73252958089122,-2.2738479695743,4.3));
#20249=CARTESIAN_POINT('Ctrl Pts',(3.72809540845025,-2.27027136680987,4.3));
#20250=CARTESIAN_POINT('Ctrl Pts',(3.72348829039508,-2.26689850911598,4.3));
#20251=CARTESIAN_POINT('Ctrl Pts',(3.72067474538276,-2.26483872101672,4.3));
#20252=CARTESIAN_POINT('Ctrl Pts',(3.71780010895487,-2.26285764263401,4.3));
#20253=CARTESIAN_POINT('Ctrl Pts',(3.71487541375918,-2.26096143585197,4.3));
#20254=CARTESIAN_POINT('Ctrl Pts',(3.70626359340869,-2.25537801909854,4.3));
#20255=CARTESIAN_POINT('Ctrl Pts',(3.69720132775591,-2.25051601191126,4.3));
#20256=CARTESIAN_POINT('Ctrl Pts',(3.6877975535831,-2.24642648892188,4.3));
#20257=CARTESIAN_POINT('Ctrl Pts',(3.67897161991428,-2.24258825780551,4.3));
#20258=CARTESIAN_POINT('Ctrl Pts',(3.66984418789588,-2.23943054868187,4.3));
#20259=CARTESIAN_POINT('Ctrl Pts',(3.66050482692203,-2.23701743659906,4.3));
#20260=CARTESIAN_POINT('Ctrl Pts',(3.65701754284817,-2.23611638915498,4.3));
#20261=CARTESIAN_POINT('Ctrl Pts',(3.65350925028094,-2.23532164136865,4.3));
#20262=CARTESIAN_POINT('Ctrl Pts',(3.64998794572223,-2.2346361398089,4.3));
#20263=CARTESIAN_POINT('Ctrl Pts',(3.63890673460959,-2.23247893148594,4.3));
#20264=CARTESIAN_POINT('Ctrl Pts',(3.62768565700141,-2.23139728883196,4.3));
#20265=CARTESIAN_POINT('Ctrl Pts',(3.61647532022068,-2.23148774583768,4.3));
#20266=CARTESIAN_POINT('Ctrl Pts',(3.61029342610439,-2.23153762798149,4.3));
#20267=CARTESIAN_POINT('Ctrl Pts',(3.60411490309515,-2.23194477515726,4.3));
#20268=CARTESIAN_POINT('Ctrl Pts',(3.59796731355722,-2.23273189751379,4.3));
#20269=CARTESIAN_POINT('Ctrl Pts',(3.59689164899642,-2.23286962297817,4.3));
#20270=CARTESIAN_POINT('Ctrl Pts',(3.59581693782457,-2.2330189937725,4.3));
#20271=CARTESIAN_POINT('Ctrl Pts',(3.5947433329992,-2.23317993884958,4.3));
#20272=CARTESIAN_POINT('Origin',(3.6,-2.4,5.35459252805377));
#20273=CARTESIAN_POINT('Ctrl Pts',(3.39434265963601,-2.39985006386652,5.17959252805377));
#20274=CARTESIAN_POINT('Ctrl Pts',(3.39426084301402,-2.39002096866549,5.17905813053169));
#20275=CARTESIAN_POINT('Ctrl Pts',(3.39937061245186,-2.31213684688635,5.17481913665734));
#20276=CARTESIAN_POINT('Ctrl Pts',(3.49890445172815,-2.1791570162937,5.16687554643073));
#20277=CARTESIAN_POINT('Ctrl Pts',(3.73070050348011,-2.19531101338576,5.15576175737392));
#20278=CARTESIAN_POINT('Ctrl Pts',(3.84286217522106,-2.398786946145,5.14464796831712));
#20279=CARTESIAN_POINT('Ctrl Pts',(3.73273070558319,-2.60338928804541,5.13353417926031));
#20280=CARTESIAN_POINT('Ctrl Pts',(3.50110863577888,-2.62181907448596,5.12242039020351));
#20281=CARTESIAN_POINT('Ctrl Pts',(3.39978420932204,-2.4892623620427,5.11443983980132));
#20282=CARTESIAN_POINT('Ctrl Pts',(3.3942709677865,-2.41067410874191,5.11016388575141));
#20283=CARTESIAN_POINT('Ctrl Pts',(3.39436118987868,-2.40016037422423,5.10959252805377));
#20284=CARTESIAN_POINT('Ctrl Pts',(3.39473290683218,-2.40022967700174,5.18540747194623));
#20285=CARTESIAN_POINT('Ctrl Pts',(3.39508769549541,-2.35320983503088,5.18286245525962));
#20286=CARTESIAN_POINT('Ctrl Pts',(3.4343446160921,-2.23704698664849,5.17661284222074));
#20287=CARTESIAN_POINT('Ctrl Pts',(3.62721323091929,-2.15871475485289,5.16665863282959));
#20288=CARTESIAN_POINT('Ctrl Pts',(3.81747535364037,-2.29190664293025,5.15554484377279));
#20289=CARTESIAN_POINT('Ctrl Pts',(3.80876232171537,-2.52413791100821,5.14443105471598));
#20290=CARTESIAN_POINT('Ctrl Pts',(3.60892556988421,-2.64269428158759,5.13331726565918));
#20291=CARTESIAN_POINT('Ctrl Pts',(3.42787437077081,-2.55254601515802,5.12364273806926));
#20292=CARTESIAN_POINT('Ctrl Pts',(3.39500775643356,-2.44179202298147,5.11767280683161));
#20293=CARTESIAN_POINT('Ctrl Pts',(3.39479089893477,-2.39988380139174,5.11540747194623));
#20294=CARTESIAN_POINT('Ctrl Pts',(3.72690708798524,-2.29206413469515,5.2));
#20295=CARTESIAN_POINT('Ctrl Pts',(3.76279833110066,-2.33426376069605,5.19629540364773));
#20296=CARTESIAN_POINT('Ctrl Pts',(3.78852079223234,-2.45658683270444,5.18888621094319));
#20297=CARTESIAN_POINT('Ctrl Pts',(3.65451255926051,-2.58934148319728,5.1777724218864));
#20298=CARTESIAN_POINT('Ctrl Pts',(3.47057723832131,-2.54835675254144,5.16665863282959));
#20299=CARTESIAN_POINT('Ctrl Pts',(3.40512138630522,-2.37179019391731,5.15554484377279));
#20300=CARTESIAN_POINT('Ctrl Pts',(3.51803130141336,-2.22093957374148,5.14443105471598));
#20301=CARTESIAN_POINT('Ctrl Pts',(3.7059725216196,-2.23403730298123,5.13331726565917));
#20302=CARTESIAN_POINT('Ctrl Pts',(3.79691367996997,-2.39901645079819,5.12220347660237));
#20303=CARTESIAN_POINT('Ctrl Pts',(3.70761861808084,-2.56490889591613,5.11108968754556));
#20304=CARTESIAN_POINT('Ctrl Pts',(3.5198184631744,-2.57985184479553,5.09997589848876));
#20305=CARTESIAN_POINT('Ctrl Pts',(3.40540965360542,-2.43017761320763,5.08886210943196));
#20306=CARTESIAN_POINT('Ctrl Pts',(3.46911145738791,-2.25287984568082,5.07774832037515));
#20307=CARTESIAN_POINT('Ctrl Pts',(3.65261709726835,-2.21024363500907,5.06663453131835));
#20308=CARTESIAN_POINT('Ctrl Pts',(3.7879616770095,-2.34129317212888,5.05552074226154));
#20309=CARTESIAN_POINT('Ctrl Pts',(3.75126281927757,-2.52607793686066,5.04440695320475));
#20310=CARTESIAN_POINT('Ctrl Pts',(3.57611137907248,-2.59546203514889,5.03329316414793));
#20311=CARTESIAN_POINT('Ctrl Pts',(3.42282546878807,-2.4859375664189,5.02217937509114));
#20312=CARTESIAN_POINT('Ctrl Pts',(3.43170941408529,-2.29775344335704,5.01106558603433));
#20313=CARTESIAN_POINT('Ctrl Pts',(3.59463164228021,-2.20315676572473,4.99995179697753));
#20314=CARTESIAN_POINT('Ctrl Pts',(3.76246758864558,-2.28873292649683,4.98883800792072));
#20315=CARTESIAN_POINT('Ctrl Pts',(3.78159510888145,-2.47615310463782,4.97772421886392));
#20316=CARTESIAN_POINT('Ctrl Pts',(3.63450656639691,-2.59386948090233,4.96661042980711));
#20317=CARTESIAN_POINT('Ctrl Pts',(3.45583377242442,-2.53413492344978,4.95549664075031));
#20318=CARTESIAN_POINT('Ctrl Pts',(3.40911796147502,-2.3516251489795,4.94438285169351));
#20319=CARTESIAN_POINT('Ctrl Pts',(3.53711864515359,-2.21339342445149,4.93326906263669));
#20320=CARTESIAN_POINT('Ctrl Pts',(3.7226753460379,-2.24596481468812,4.9221552735799));
#20321=CARTESIAN_POINT('Ctrl Pts',(3.7959459114648,-2.41952635696717,4.91104148452308));
#20322=CARTESIAN_POINT('Ctrl Pts',(3.68986496194813,-2.57521520324594,4.89992769546629));
#20323=CARTESIAN_POINT('Ctrl Pts',(3.50152959362338,-2.57052758693027,4.88881390640948));
#20324=CARTESIAN_POINT('Ctrl Pts',(3.403325304985,-2.4097541363769,4.87770011735268));
#20325=CARTESIAN_POINT('Ctrl Pts',(3.48513959513685,-2.24005261418135,4.86658632829587));
#20326=CARTESIAN_POINT('Ctrl Pts',(3.6720869164654,-2.21675274815082,4.85547253923907));
#20327=CARTESIAN_POINT('Ctrl Pts',(3.79305226563199,-2.36118116990379,4.84435875018227));
#20328=CARTESIAN_POINT('Ctrl Pts',(3.73731468670399,-2.54114090707891,4.83324496112546));
#20329=CARTESIAN_POINT('Ctrl Pts',(3.55589141778138,-2.59191277135814,4.82213117206866));
#20330=CARTESIAN_POINT('Ctrl Pts',(3.41484123438881,-2.46702469957432,4.81101738301185));
#20331=CARTESIAN_POINT('Ctrl Pts',(3.44326896900338,-2.28078816015838,4.79990359395505));
#20332=CARTESIAN_POINT('Ctrl Pts',(3.61515439373994,-2.20366756970366,4.78878980489824));
#20333=CARTESIAN_POINT('Ctrl Pts',(3.77316883002382,-2.3062522792604,4.77767601584144));
#20334=CARTESIAN_POINT('Ctrl Pts',(3.77267987231879,-2.49464534078155,4.76656222678464));
#20335=CARTESIAN_POINT('Ctrl Pts',(3.61413506915742,-2.59640844853418,4.75544843772783));
#20336=CARTESIAN_POINT('Ctrl Pts',(3.44265227689368,-2.51839667592017,4.74433464867102));
#20337=CARTESIAN_POINT('Ctrl Pts',(3.4151916400337,-2.33201508312681,4.73322085961423));
#20338=CARTESIAN_POINT('Ctrl Pts',(3.55688819092022,-2.20786085574886,4.72210707055742));
#20339=CARTESIAN_POINT('Ctrl Pts',(3.73804546957863,-2.25957376611009,4.71099328150061));
#20340=CARTESIAN_POINT('Ctrl Pts',(3.79284816438962,-2.43982040089255,4.69987949244382));
#20341=CARTESIAN_POINT('Ctrl Pts',(3.67113474728785,-2.58361897114401,4.688765703387));
#20342=CARTESIAN_POINT('Ctrl Pts',(3.48431088927061,-2.55934901472658,4.67765191433021));
#20343=CARTESIAN_POINT('Ctrl Pts',(3.40337858630773,-2.38922509798919,4.66653812527339));
#20344=CARTESIAN_POINT('Ctrl Pts',(3.50241609313587,-2.22896357125796,4.6554243362166));
#20345=CARTESIAN_POINT('Ctrl Pts',(3.69077325659353,-2.22525362743943,4.64431054715978));
#20346=CARTESIAN_POINT('Ctrl Pts',(3.79604462885236,-2.38149102018406,4.63319675810299));
#20347=CARTESIAN_POINT('Ctrl Pts',(3.72187412902538,-2.5546698920607,4.62208296904618));
#20348=CARTESIAN_POINT('Ctrl Pts',(3.53615085675469,-2.58627765765756,4.61096917998938));
#20349=CARTESIAN_POINT('Ctrl Pts',(3.40886942939528,-2.44738337066962,4.59985539093257));
#20350=CARTESIAN_POINT('Ctrl Pts',(3.45653198087784,-2.26511854714084,4.58874160187577));
#20351=CARTESIAN_POINT('Ctrl Pts',(3.63551243730216,-2.20631224707971,4.57762781281896));
#20352=CARTESIAN_POINT('Ctrl Pts',(3.78198795712288,-2.32479054382313,4.56651402376216));
#20353=CARTESIAN_POINT('Ctrl Pts',(3.76188783591025,-2.51210890876234,4.55540023470536));
#20354=CARTESIAN_POINT('Ctrl Pts',(3.59360994254596,-2.59681271806211,4.54428644564855));
#20355=CARTESIAN_POINT('Ctrl Pts',(3.43118094125773,-2.50137161460726,4.53317265659175));
#20356=CARTESIAN_POINT('Ctrl Pts',(3.42327393893419,-2.31314392247853,4.52205886753494));
#20357=CARTESIAN_POINT('Ctrl Pts',(3.57712630459504,-2.2044165835037,4.51094507847814));
#20358=CARTESIAN_POINT('Ctrl Pts',(3.75191522290318,-2.2747089629466,4.49983128942133));
#20359=CARTESIAN_POINT('Ctrl Pts',(3.78765441517707,-2.45968165103968,4.48871750036453));
#20360=CARTESIAN_POINT('Ctrl Pts',(3.6516313924431,-2.59002704401991,4.47760371130773));
#20361=CARTESIAN_POINT('Ctrl Pts',(3.46834957196871,-2.54643853472375,4.46648992225092));
#20362=CARTESIAN_POINT('Ctrl Pts',(3.40556887868038,-2.36881316151698,4.45537613319412));
#20363=CARTESIAN_POINT('Ctrl Pts',(3.52075320095807,-2.21973347999151,4.44426234413732));
#20364=CARTESIAN_POINT('Ctrl Pts',(3.70847300665902,-2.23565373905929,4.43314855508051));
#20365=CARTESIAN_POINT('Ctrl Pts',(3.79690626014289,-2.40200209376731,4.4220347660237));
#20366=CARTESIAN_POINT('Ctrl Pts',(3.70510893870568,-2.56651771072077,4.4109209769669));
#20367=CARTESIAN_POINT('Ctrl Pts',(3.51710429764661,-2.57861817635772,4.3998071879101));
#20368=CARTESIAN_POINT('Ctrl Pts',(3.4049748648587,-2.42722660301959,4.3886933988533));
#20369=CARTESIAN_POINT('Ctrl Pts',(3.47135448681048,-2.25091580613535,4.37757960979649));
#20370=CARTESIAN_POINT('Ctrl Pts',(3.65548413146169,-2.21106026869437,4.36646582073969));
#20371=CARTESIAN_POINT('Ctrl Pts',(3.78882987196794,-2.34414980590083,4.35535203168288));
#20372=CARTESIAN_POINT('Ctrl Pts',(3.74933478455633,-2.5283468513898,4.34423824262608));
#20373=CARTESIAN_POINT('Ctrl Pts',(3.57315729153603,-2.59509221614966,4.33312445356927));
#20374=CARTESIAN_POINT('Ctrl Pts',(3.42153838470822,-2.4832160988167,4.32201066451247));
#20375=CARTESIAN_POINT('Ctrl Pts',(3.43328918604681,-2.2952742544727,4.31089687545567));
#20376=CARTESIAN_POINT('Ctrl Pts',(3.59758810222901,-2.20298223652265,4.29978308639886));
#20377=CARTESIAN_POINT('Ctrl Pts',(3.76418972838082,-2.29144636425406,4.28866929734206));
#20378=CARTESIAN_POINT('Ctrl Pts',(3.77483953817107,-2.41599017382994,4.28126010463752));
#20379=CARTESIAN_POINT('Ctrl Pts',(3.75264423560529,-2.46674801372684,4.27755550828525));
#20380=CARTESIAN_POINT('Ctrl Pts',(3.73677806246588,-2.28366876301903,5.20748149723825));
#20381=CARTESIAN_POINT('Ctrl Pts',(3.77546096639785,-2.32915072287504,5.20377690088598));
#20382=CARTESIAN_POINT('Ctrl Pts',(3.80318414917118,-2.46098821950194,5.19636770818144));
#20383=CARTESIAN_POINT('Ctrl Pts',(3.65875260676202,-2.60406867439235,5.18525391912464));
#20384=CARTESIAN_POINT('Ctrl Pts',(3.46051059194224,-2.55989610579284,5.17414013006784));
#20385=CARTESIAN_POINT('Ctrl Pts',(3.38996351094031,-2.36959600381834,5.16302634101104));
#20386=CARTESIAN_POINT('Ctrl Pts',(3.51165568485162,-2.20701205459222,5.15191255195423));
#20387=CARTESIAN_POINT('Ctrl Pts',(3.71421518223977,-2.22112853978274,5.14079876289742));
#20388=CARTESIAN_POINT('Ctrl Pts',(3.81222984505367,-2.39893994924713,5.12968497384063));
#20389=CARTESIAN_POINT('Ctrl Pts',(3.71598931391495,-2.57773569329255,5.11857118478381));
#20390=CARTESIAN_POINT('Ctrl Pts',(3.51358185404256,-2.59384092135901,5.10745739572702));
#20391=CARTESIAN_POINT('Ctrl Pts',(3.3902741999918,-2.43252486153385,5.0963436066702));
#20392=CARTESIAN_POINT('Ctrl Pts',(3.45893080093723,-2.2414366764148,5.08522981761341));
#20393=CARTESIAN_POINT('Ctrl Pts',(3.65670971362751,-2.19548417384656,5.07411602855659));
#20394=CARTESIAN_POINT('Ctrl Pts',(3.80258154534432,-2.33672688974895,5.0630022394998));
#20395=CARTESIAN_POINT('Ctrl Pts',(3.76302820963254,-2.53588441904446,5.05188845044299));
#20396=CARTESIAN_POINT('Ctrl Pts',(3.57425329556196,-2.61066528968353,5.04077466138618));
#20397=CARTESIAN_POINT('Ctrl Pts',(3.40904463665349,-2.49262188593578,5.02966087232938));
#20398=CARTESIAN_POINT('Ctrl Pts',(3.41861958509882,-2.28980059243768,5.01854708327258));
#20399=CARTESIAN_POINT('Ctrl Pts',(3.59421408544476,-2.18784607998553,5.00743329421577));
#20400=CARTESIAN_POINT('Ctrl Pts',(3.77510449842668,-2.28007844974125,4.99631950515897));
#20401=CARTESIAN_POINT('Ctrl Pts',(3.79571977846481,-2.48207637783269,4.98520571610217));
#20402=CARTESIAN_POINT('Ctrl Pts',(3.63719052551791,-2.60894886479604,4.97409192704536));
#20403=CARTESIAN_POINT('Ctrl Pts',(3.4446203628666,-2.54456808701342,4.96297813798855));
#20404=CARTESIAN_POINT('Ctrl Pts',(3.39427094417278,-2.34786249925276,4.95186434893176));
#20405=CARTESIAN_POINT('Ctrl Pts',(3.53222766342159,-2.19887895741578,4.94075055987495));
#20406=CARTESIAN_POINT('Ctrl Pts',(3.73221717092231,-2.23398378661889,4.92963677081814));
#20407=CARTESIAN_POINT('Ctrl Pts',(3.81118680243757,-2.42104513873408,4.91852298176134));
#20408=CARTESIAN_POINT('Ctrl Pts',(3.69685475865827,-2.58884363667168,4.90740919270454));
#20409=CARTESIAN_POINT('Ctrl Pts',(3.4938704558725,-2.58379141234426,4.89629540364773));
#20410=CARTESIAN_POINT('Ctrl Pts',(3.38802772841696,-2.41051282395524,4.88518161459093));
#20411=CARTESIAN_POINT('Ctrl Pts',(3.47620562507071,-2.22761172857971,4.87406782553412));
#20412=CARTESIAN_POINT('Ctrl Pts',(3.67769391702081,-2.20249957304951,4.86295403647733));
#20413=CARTESIAN_POINT('Ctrl Pts',(3.80806808561287,-2.35816179811509,4.85184024742051));
#20414=CARTESIAN_POINT('Ctrl Pts',(3.74799517579086,-2.552119003843,4.84072645836372));
#20415=CARTESIAN_POINT('Ctrl Pts',(3.55246060318804,-2.60683996020677,4.8296126693069));
#20416=CARTESIAN_POINT('Ctrl Pts',(3.40043937962063,-2.4722379552685,4.8184988802501));
#20417=CARTESIAN_POINT('Ctrl Pts',(3.43107825505782,-2.27151573063888,4.8073850911933));
#20418=CARTESIAN_POINT('Ctrl Pts',(3.61633311934347,-2.18839661486619,4.79627130213649));
#20419=CARTESIAN_POINT('Ctrl Pts',(3.78663809426387,-2.29896047725209,4.78515751307969));
#20420=CARTESIAN_POINT('Ctrl Pts',(3.7861111048846,-2.50200696067527,4.77404372402288));
#20421=CARTESIAN_POINT('Ctrl Pts',(3.61523451056097,-2.61168531615476,4.76292993496608));
#20422=CARTESIAN_POINT('Ctrl Pts',(3.43041359594979,-2.52760570108303,4.75181614590928));
#20423=CARTESIAN_POINT('Ctrl Pts',(3.40081704020639,-2.32672714066293,4.74070235685248));
#20424=CARTESIAN_POINT('Ctrl Pts',(3.55353490645048,-2.19291605936479,4.72958856779566));
#20425=CARTESIAN_POINT('Ctrl Pts',(3.74878279977045,-2.24865125742167,4.71847477873887));
#20426=CARTESIAN_POINT('Ctrl Pts',(3.80784810914882,-2.44291767597198,4.70736098968206));
#20427=CARTESIAN_POINT('Ctrl Pts',(3.67666768706539,-2.59790105898559,4.69624720062525));
#20428=CARTESIAN_POINT('Ctrl Pts',(3.47531246154031,-2.57174335835902,4.68513341156846));
#20429=CARTESIAN_POINT('Ctrl Pts',(3.38808515402025,-2.38838701412431,4.67401962251165));
#20430=CARTESIAN_POINT('Ctrl Pts',(3.49482590830325,-2.21566016756178,4.66290583345484));
#20431=CARTESIAN_POINT('Ctrl Pts',(3.69783370147164,-2.21166166018595,4.65179204439804));
#20432=CARTESIAN_POINT('Ctrl Pts',(3.81129319817336,-2.38005137114376,4.64067825534124));
#20433=CARTESIAN_POINT('Ctrl Pts',(3.73135363435924,-2.56670028832692,4.62956446628443));
#20434=CARTESIAN_POINT('Ctrl Pts',(3.53118459936441,-2.60076654109381,4.61845067722763));
#20435=CARTESIAN_POINT('Ctrl Pts',(3.3940030809914,-2.45106890195169,4.60733688817082));
#20436=CARTESIAN_POINT('Ctrl Pts',(3.44537287875023,-2.25462731768926,4.59622309911402));
#20437=CARTESIAN_POINT('Ctrl Pts',(3.63827463418116,-2.1912469981906,4.58510931005721));
#20438=CARTESIAN_POINT('Ctrl Pts',(3.79614318287948,-2.31894066865531,4.57399552100041));
#20439=CARTESIAN_POINT('Ctrl Pts',(3.77447965187866,-2.52082886440086,4.56288173194361));
#20440=CARTESIAN_POINT('Ctrl Pts',(3.59311291676859,-2.6121210302163,4.55176794288681));
#20441=CARTESIAN_POINT('Ctrl Pts',(3.41805000706685,-2.50925641156176,4.54065415383));
#20442=CARTESIAN_POINT('Ctrl Pts',(3.40952798930647,-2.3063881601463,4.52954036477319));
#20443=CARTESIAN_POINT('Ctrl Pts',(3.57534716312072,-2.18920388779283,4.51842657571639));
#20444=CARTESIAN_POINT('Ctrl Pts',(3.76373135793792,-2.26496368670519,4.50731278665958));
#20445=CARTESIAN_POINT('Ctrl Pts',(3.80225038434475,-2.46432375625011,4.49619899760278));
#20446=CARTESIAN_POINT('Ctrl Pts',(3.65564733958441,-2.60480755889841,4.48508520854597));
#20447=CARTESIAN_POINT('Ctrl Pts',(3.45810965522258,-2.55782868685937,4.47397141948917));
#20448=CARTESIAN_POINT('Ctrl Pts',(3.39044580977021,-2.36638741452612,4.46285763043237));
#20449=CARTESIAN_POINT('Ctrl Pts',(3.51458929677089,-2.20571214952866,4.45174384137556));
#20450=CARTESIAN_POINT('Ctrl Pts',(3.71691015778721,-2.22287070405714,4.44063005231876));
#20451=CARTESIAN_POINT('Ctrl Pts',(3.81222184810419,-2.40215781884775,4.42951626326195));
#20452=CARTESIAN_POINT('Ctrl Pts',(3.71328442888611,-2.57946964350242,4.41840247420515));
#20453=CARTESIAN_POINT('Ctrl Pts',(3.51065657770066,-2.59251129681771,4.40728868514835));
#20454=CARTESIAN_POINT('Ctrl Pts',(3.38980559289267,-2.42934431849055,4.39617489609154));
#20455=CARTESIAN_POINT('Ctrl Pts',(3.46134829568354,-2.23931987168859,4.38506110703474));
#20456=CARTESIAN_POINT('Ctrl Pts',(3.65979974892982,-2.19636432620836,4.37394731797793));
#20457=CARTESIAN_POINT('Ctrl Pts',(3.80351726947246,-2.33980571567353,4.36283352892113));
#20458=CARTESIAN_POINT('Ctrl Pts',(3.76095021022585,-2.5383298122697,4.35171973986433));
#20459=CARTESIAN_POINT('Ctrl Pts',(3.57106943581066,-2.61026670575114,4.34060595080752));
#20460=CARTESIAN_POINT('Ctrl Pts',(3.4076574417421,-2.48968873955599,4.32949216175071));
#20461=CARTESIAN_POINT('Ctrl Pts',(3.42032223348093,-2.28712856948396,4.31837837269392));
#20462=CARTESIAN_POINT('Ctrl Pts',(3.59740050213728,-2.18765797570795,4.30726458363711));
#20463=CARTESIAN_POINT('Ctrl Pts',(3.77696058810632,-2.28300294170579,4.29615079458031));
#20464=CARTESIAN_POINT('Ctrl Pts',(3.78843875194939,-2.41723390733862,4.28874160187577));
#20465=CARTESIAN_POINT('Ctrl Pts',(3.76451707405898,-2.471939748488,4.2850370055235));
#20466=CARTESIAN_POINT('Ctrl Pts',(3.74664903694653,-2.2752733913429,5.2149629944765));
#20467=CARTESIAN_POINT('Ctrl Pts',(3.78812360169505,-2.32403768505403,5.21125839812423));
#20468=CARTESIAN_POINT('Ctrl Pts',(3.81784750611002,-2.46538960629943,5.20384920541969));
#20469=CARTESIAN_POINT('Ctrl Pts',(3.66299265426352,-2.61879586558741,5.19273541636289));
#20470=CARTESIAN_POINT('Ctrl Pts',(3.45044394556317,-2.57143545904423,5.18162162730609));
#20471=CARTESIAN_POINT('Ctrl Pts',(3.37480563557539,-2.36740181371937,5.17050783824928));
#20472=CARTESIAN_POINT('Ctrl Pts',(3.50528006828989,-2.19308453544296,5.15939404919248));
#20473=CARTESIAN_POINT('Ctrl Pts',(3.72245784285994,-2.20821977658425,5.14828026013567));
#20474=CARTESIAN_POINT('Ctrl Pts',(3.82754601013736,-2.39886344769606,5.13716647107887));
#20475=CARTESIAN_POINT('Ctrl Pts',(3.72436000974907,-2.59056249066898,5.12605268202206));
#20476=CARTESIAN_POINT('Ctrl Pts',(3.50734524491072,-2.60782999792249,5.11493889296526));
#20477=CARTESIAN_POINT('Ctrl Pts',(3.37513874637818,-2.43487210986008,5.10382510390845));
#20478=CARTESIAN_POINT('Ctrl Pts',(3.44875014448657,-2.22999350714877,5.09271131485166));
#20479=CARTESIAN_POINT('Ctrl Pts',(3.66080232998667,-2.18072471268405,5.08159752579485));
#20480=CARTESIAN_POINT('Ctrl Pts',(3.81720141367915,-2.33216060736901,5.07048373673804));
#20481=CARTESIAN_POINT('Ctrl Pts',(3.77479359998752,-2.54569090122825,5.05936994768124));
#20482=CARTESIAN_POINT('Ctrl Pts',(3.57239521205144,-2.62586854421817,5.04825615862443));
#20483=CARTESIAN_POINT('Ctrl Pts',(3.39526380451891,-2.49930620545266,5.03714236956763));
#20484=CARTESIAN_POINT('Ctrl Pts',(3.40552975611236,-2.28184774151832,5.02602858051083));
#20485=CARTESIAN_POINT('Ctrl Pts',(3.59379652860931,-2.17253539424633,5.01491479145402));
#20486=CARTESIAN_POINT('Ctrl Pts',(3.78774140820779,-2.27142397298568,5.00380100239722));
#20487=CARTESIAN_POINT('Ctrl Pts',(3.80984444804818,-2.48799965102756,4.99268721334042));
#20488=CARTESIAN_POINT('Ctrl Pts',(3.63987448463892,-2.62402824868975,4.98157342428361));
#20489=CARTESIAN_POINT('Ctrl Pts',(3.43340695330878,-2.55500125057707,4.9704596352268));
#20490=CARTESIAN_POINT('Ctrl Pts',(3.37942392687054,-2.34409984952602,4.95934584617001));
#20491=CARTESIAN_POINT('Ctrl Pts',(3.52733668168959,-2.18436449038006,4.94823205711319));
#20492=CARTESIAN_POINT('Ctrl Pts',(3.74175899580671,-2.22200275854966,4.9371182680564));
#20493=CARTESIAN_POINT('Ctrl Pts',(3.82642769341035,-2.42256392050098,4.92600447899958));
#20494=CARTESIAN_POINT('Ctrl Pts',(3.70384455536842,-2.60247207009742,4.91489068994279));
#20495=CARTESIAN_POINT('Ctrl Pts',(3.48621131812161,-2.59705523775825,4.90377690088598));
#20496=CARTESIAN_POINT('Ctrl Pts',(3.37273015184892,-2.41127151153357,4.89266311182918));
#20497=CARTESIAN_POINT('Ctrl Pts',(3.46727165500458,-2.21517084297807,4.88154932277238));
#20498=CARTESIAN_POINT('Ctrl Pts',(3.68330091757622,-2.1882463979482,4.87043553371556));
#20499=CARTESIAN_POINT('Ctrl Pts',(3.82308390559375,-2.3551424263264,4.85932174465877));
#20500=CARTESIAN_POINT('Ctrl Pts',(3.75867566487773,-2.56309710060709,4.84820795560196));
#20501=CARTESIAN_POINT('Ctrl Pts',(3.54902978859471,-2.62176714905541,4.83709416654515));
#20502=CARTESIAN_POINT('Ctrl Pts',(3.38603752485245,-2.47745121096268,4.82598037748835));
#20503=CARTESIAN_POINT('Ctrl Pts',(3.41888754111225,-2.26224330111939,4.81486658843154));
#20504=CARTESIAN_POINT('Ctrl Pts',(3.61751184494699,-2.17312566002871,4.80375279937474));
#20505=CARTESIAN_POINT('Ctrl Pts',(3.80010735850391,-2.29166867524379,4.79263901031795));
#20506=CARTESIAN_POINT('Ctrl Pts',(3.79954233745042,-2.50936858056899,4.78152522126113));
#20507=CARTESIAN_POINT('Ctrl Pts',(3.61633395196453,-2.62696218377534,4.77041143220433));
#20508=CARTESIAN_POINT('Ctrl Pts',(3.4181749150059,-2.53681472624589,4.75929764314752));
#20509=CARTESIAN_POINT('Ctrl Pts',(3.38644244037908,-2.32143919819905,4.74818385409072));
#20510=CARTESIAN_POINT('Ctrl Pts',(3.55018162198074,-2.1779712629807,4.73707006503392));
#20511=CARTESIAN_POINT('Ctrl Pts',(3.75952012996226,-2.23772874873326,4.72595627597711));
#20512=CARTESIAN_POINT('Ctrl Pts',(3.82284805390801,-2.44601495105141,4.71484248692031));
#20513=CARTESIAN_POINT('Ctrl Pts',(3.68220062684293,-2.61218314682717,4.7037286978635));
#20514=CARTESIAN_POINT('Ctrl Pts',(3.46631403381001,-2.58413770199147,4.69261490880671));
#20515=CARTESIAN_POINT('Ctrl Pts',(3.37279172173275,-2.38754893025942,4.68150111974989));
#20516=CARTESIAN_POINT('Ctrl Pts',(3.48723572347063,-2.20235676386561,4.6703873306931));
#20517=CARTESIAN_POINT('Ctrl Pts',(3.70489414634973,-2.19806969293246,4.65927354163628));
#20518=CARTESIAN_POINT('Ctrl Pts',(3.82654176749436,-2.37861172210345,4.64815975257949));
#20519=CARTESIAN_POINT('Ctrl Pts',(3.7408331396931,-2.57873068459315,4.63704596352267));
#20520=CARTESIAN_POINT('Ctrl Pts',(3.52621834197413,-2.61525542453006,4.62593217446588));
#20521=CARTESIAN_POINT('Ctrl Pts',(3.37913673258752,-2.45475443323377,4.61481838540907));
#20522=CARTESIAN_POINT('Ctrl Pts',(3.43421377662264,-2.24413608823767,4.60370459635227));
#20523=CARTESIAN_POINT('Ctrl Pts',(3.64103683106015,-2.17618174930149,4.59259080729546));
#20524=CARTESIAN_POINT('Ctrl Pts',(3.81029840863609,-2.31309079348749,4.58147701823866));
#20525=CARTESIAN_POINT('Ctrl Pts',(3.78707146784707,-2.52954882003939,4.57036322918186));
#20526=CARTESIAN_POINT('Ctrl Pts',(3.59261589099123,-2.62742934237049,4.55924944012505));
#20527=CARTESIAN_POINT('Ctrl Pts',(3.40491907287596,-2.51714120851626,4.54813565106824));
#20528=CARTESIAN_POINT('Ctrl Pts',(3.39578203967876,-2.29963239781408,4.53702186201144));
#20529=CARTESIAN_POINT('Ctrl Pts',(3.57356802164639,-2.17399119208196,4.52590807295464));
#20530=CARTESIAN_POINT('Ctrl Pts',(3.77554749297266,-2.2552184104638,4.51479428389784));
#20531=CARTESIAN_POINT('Ctrl Pts',(3.81684635351243,-2.46896586146052,4.50368049484103));
#20532=CARTESIAN_POINT('Ctrl Pts',(3.65966328672572,-2.61958807377691,4.49256670578423));
#20533=CARTESIAN_POINT('Ctrl Pts',(3.44786973847645,-2.56921883899499,4.48145291672742));
#20534=CARTESIAN_POINT('Ctrl Pts',(3.37532274086005,-2.36396166753528,4.47033912767061));
#20535=CARTESIAN_POINT('Ctrl Pts',(3.5084253925837,-2.19169081906581,4.45922533861382));
#20536=CARTESIAN_POINT('Ctrl Pts',(3.7253473089154,-2.21008766905501,4.44811154955701));
#20537=CARTESIAN_POINT('Ctrl Pts',(3.82753743606548,-2.40231354392819,4.43699776050021));
#20538=CARTESIAN_POINT('Ctrl Pts',(3.72145991906655,-2.59242157628407,4.4258839714434));
#20539=CARTESIAN_POINT('Ctrl Pts',(3.5042088577547,-2.60640441727771,4.41477018238659));
#20540=CARTESIAN_POINT('Ctrl Pts',(3.37463632092665,-2.43146203396151,4.4036563933298));
#20541=CARTESIAN_POINT('Ctrl Pts',(3.45134210455661,-2.22772393724184,4.39254260427299));
#20542=CARTESIAN_POINT('Ctrl Pts',(3.66411536639796,-2.18166838372235,4.38142881521618));
#20543=CARTESIAN_POINT('Ctrl Pts',(3.81820466697696,-2.33546162544623,4.37031502615938));
#20544=CARTESIAN_POINT('Ctrl Pts',(3.77256563589538,-2.54831277314961,4.35920123710258));
#20545=CARTESIAN_POINT('Ctrl Pts',(3.5689815800853,-2.62544119535262,4.34808744804577));
#20546=CARTESIAN_POINT('Ctrl Pts',(3.39377649877598,-2.49616138029528,4.33697365898897));
#20547=CARTESIAN_POINT('Ctrl Pts',(3.40735528091504,-2.27898288449522,4.32585986993216));
#20548=CARTESIAN_POINT('Ctrl Pts',(3.59721290204555,-2.17233371489326,4.31474608087536));
#20549=CARTESIAN_POINT('Ctrl Pts',(3.78973144783182,-2.27455951915752,4.30363229181856));
#20550=CARTESIAN_POINT('Ctrl Pts',(3.8020379657277,-2.4184776408473,4.29622309911402));
#20551=CARTESIAN_POINT('Ctrl Pts',(3.77638991251267,-2.47713148324917,4.29251850276175));
#20552=CARTESIAN_POINT('Ctrl Pts',(3.75652001142717,-2.26687801966678,5.22244449171475));
#20553=CARTESIAN_POINT('Ctrl Pts',(3.80078623699225,-2.31892464723302,5.21873989536248));
#20554=CARTESIAN_POINT('Ctrl Pts',(3.83251086304886,-2.46979099309691,5.21133070265794));
#20555=CARTESIAN_POINT('Ctrl Pts',(3.66723270176503,-2.63352305678248,5.20021691360114));
#20556=CARTESIAN_POINT('Ctrl Pts',(3.4403772991841,-2.58297481229563,5.18910312454433));
#20557=CARTESIAN_POINT('Ctrl Pts',(3.35964776021048,-2.3652076236204,5.17798933548753));
#20558=CARTESIAN_POINT('Ctrl Pts',(3.49890445172815,-2.1791570162937,5.16687554643073));
#20559=CARTESIAN_POINT('Ctrl Pts',(3.73070050348011,-2.19531101338576,5.15576175737392));
#20560=CARTESIAN_POINT('Ctrl Pts',(3.84286217522106,-2.398786946145,5.14464796831712));
#20561=CARTESIAN_POINT('Ctrl Pts',(3.73273070558319,-2.60338928804541,5.13353417926031));
#20562=CARTESIAN_POINT('Ctrl Pts',(3.50110863577888,-2.62181907448596,5.12242039020351));
#20563=CARTESIAN_POINT('Ctrl Pts',(3.36000329276455,-2.4372193581863,5.1113066011467));
#20564=CARTESIAN_POINT('Ctrl Pts',(3.4385694880359,-2.21855033788275,5.10019281208991));
#20565=CARTESIAN_POINT('Ctrl Pts',(3.66489494634582,-2.16596525152154,5.08907902303309));
#20566=CARTESIAN_POINT('Ctrl Pts',(3.83182128201397,-2.32759432498908,5.07796523397629));
#20567=CARTESIAN_POINT('Ctrl Pts',(3.78655899034249,-2.55549738341204,5.06685144491949));
#20568=CARTESIAN_POINT('Ctrl Pts',(3.57053712854092,-2.64107179875281,5.05573765586268));
#20569=CARTESIAN_POINT('Ctrl Pts',(3.38148297238433,-2.50599052496954,5.04462386680588));
#20570=CARTESIAN_POINT('Ctrl Pts',(3.3924399271259,-2.27389489059897,5.03351007774908));
#20571=CARTESIAN_POINT('Ctrl Pts',(3.59337897177386,-2.15722470850713,5.02239628869227));
#20572=CARTESIAN_POINT('Ctrl Pts',(3.8003783179889,-2.26276949623011,5.01128249963547));
#20573=CARTESIAN_POINT('Ctrl Pts',(3.82396911763155,-2.49392292422242,5.00016871057867));
#20574=CARTESIAN_POINT('Ctrl Pts',(3.64255844375993,-2.63910763258347,4.98905492152186));
#20575=CARTESIAN_POINT('Ctrl Pts',(3.42219354375095,-2.56543441414071,4.97794113246505));
#20576=CARTESIAN_POINT('Ctrl Pts',(3.3645769095683,-2.34033719979929,4.96682734340826));
#20577=CARTESIAN_POINT('Ctrl Pts',(3.52244569995759,-2.16985002334435,4.95571355435144));
#20578=CARTESIAN_POINT('Ctrl Pts',(3.75130082069111,-2.21002173048044,4.94459976529465));
#20579=CARTESIAN_POINT('Ctrl Pts',(3.84166858438312,-2.42408270226789,4.93348597623783));
#20580=CARTESIAN_POINT('Ctrl Pts',(3.71083435207858,-2.61610050352316,4.92237218718104));
#20581=CARTESIAN_POINT('Ctrl Pts',(3.47855218037073,-2.61031906317225,4.91125839812423));
#20582=CARTESIAN_POINT('Ctrl Pts',(3.35743257528088,-2.4120301991119,4.90014460906743));
#20583=CARTESIAN_POINT('Ctrl Pts',(3.45833768493844,-2.20272995737643,4.88903082001062));
#20584=CARTESIAN_POINT('Ctrl Pts',(3.68890791813162,-2.17399322284688,4.87791703095382));
#20585=CARTESIAN_POINT('Ctrl Pts',(3.83809972557463,-2.3521230545377,4.86680324189701));
#20586=CARTESIAN_POINT('Ctrl Pts',(3.76935615396461,-2.57407519737118,4.85568945284021));
#20587=CARTESIAN_POINT('Ctrl Pts',(3.54559897400137,-2.63669433790405,4.8445756637834));
#20588=CARTESIAN_POINT('Ctrl Pts',(3.37163567008428,-2.48266446665686,4.8334618747266));
#20589=CARTESIAN_POINT('Ctrl Pts',(3.40669682716669,-2.25297087159989,4.8223480856698));
#20590=CARTESIAN_POINT('Ctrl Pts',(3.61869057055051,-2.15785470519124,4.81123429661299));
#20591=CARTESIAN_POINT('Ctrl Pts',(3.81357662274397,-2.28437687323548,4.80012050755619));
#20592=CARTESIAN_POINT('Ctrl Pts',(3.81297357001622,-2.51673020046272,4.78900671849938));
#20593=CARTESIAN_POINT('Ctrl Pts',(3.61743339336808,-2.64223905139592,4.77789292944258));
#20594=CARTESIAN_POINT('Ctrl Pts',(3.405936234062,-2.54602375140875,4.76677914038577));
#20595=CARTESIAN_POINT('Ctrl Pts',(3.37206784055177,-2.31615125573517,4.75566535132898));
#20596=CARTESIAN_POINT('Ctrl Pts',(3.546828337511,-2.16302646659663,4.74455156227216));
#20597=CARTESIAN_POINT('Ctrl Pts',(3.77025746015408,-2.22680624004484,4.73343777321537));
#20598=CARTESIAN_POINT('Ctrl Pts',(3.83784799866721,-2.44911222613084,4.72232398415856));
#20599=CARTESIAN_POINT('Ctrl Pts',(3.68773356662048,-2.62646523466876,4.71121019510175));
#20600=CARTESIAN_POINT('Ctrl Pts',(3.4573156060797,-2.59653204562391,4.70009640604496));
#20601=CARTESIAN_POINT('Ctrl Pts',(3.35749828944527,-2.38671084639454,4.68898261698814));
#20602=CARTESIAN_POINT('Ctrl Pts',(3.47964553863801,-2.18905336016944,4.67786882793135));
#20603=CARTESIAN_POINT('Ctrl Pts',(3.71195459122784,-2.18447772567898,4.66675503887453));
#20604=CARTESIAN_POINT('Ctrl Pts',(3.84179033681535,-2.37717207306315,4.65564124981774));
#20605=CARTESIAN_POINT('Ctrl Pts',(3.75031264502696,-2.59076108085938,4.64452746076093));
#20606=CARTESIAN_POINT('Ctrl Pts',(3.52125208458385,-2.6297443079663,4.63341367170413));
#20607=CARTESIAN_POINT('Ctrl Pts',(3.36427038418365,-2.45843996451585,4.62229988264732));
#20608=CARTESIAN_POINT('Ctrl Pts',(3.42305467449503,-2.23364485878609,4.61118609359052));
#20609=CARTESIAN_POINT('Ctrl Pts',(3.64379902793915,-2.16111650041238,4.60007230453371));
#20610=CARTESIAN_POINT('Ctrl Pts',(3.82445363439269,-2.30724091831967,4.58895851547691));
#20611=CARTESIAN_POINT('Ctrl Pts',(3.79966328381548,-2.53826877567792,4.57784472642011));
#20612=CARTESIAN_POINT('Ctrl Pts',(3.59211886521387,-2.64273765452468,4.5667309373633));
#20613=CARTESIAN_POINT('Ctrl Pts',(3.39178813868507,-2.52502600547076,4.5556171483065));
#20614=CARTESIAN_POINT('Ctrl Pts',(3.38203609005104,-2.29287663548185,4.54450335924969));
#20615=CARTESIAN_POINT('Ctrl Pts',(3.57178888017207,-2.15877849637109,4.53338957019289));
#20616=CARTESIAN_POINT('Ctrl Pts',(3.78736362800739,-2.2454731342224,4.52227578113608));
#20617=CARTESIAN_POINT('Ctrl Pts',(3.83144232268012,-2.47360796667095,4.51116199207928));
#20618=CARTESIAN_POINT('Ctrl Pts',(3.66367923386702,-2.6343685886554,4.50004820302247));
#20619=CARTESIAN_POINT('Ctrl Pts',(3.43762982173032,-2.58060899113062,4.48893441396567));
#20620=CARTESIAN_POINT('Ctrl Pts',(3.36019967194989,-2.36153592054442,4.47782062490886));
#20621=CARTESIAN_POINT('Ctrl Pts',(3.50226148839652,-2.17766948860297,4.46670683585206));
#20622=CARTESIAN_POINT('Ctrl Pts',(3.73378446004359,-2.19730463405286,4.45559304679526));
#20623=CARTESIAN_POINT('Ctrl Pts',(3.84285302402677,-2.40246926900864,4.44447925773845));
#20624=CARTESIAN_POINT('Ctrl Pts',(3.72963540924699,-2.60537350906572,4.43336546868165));
#20625=CARTESIAN_POINT('Ctrl Pts',(3.49776113780875,-2.62029753773771,4.42225167962485));
#20626=CARTESIAN_POINT('Ctrl Pts',(3.35946704896063,-2.43357974943247,4.41113789056804));
#20627=CARTESIAN_POINT('Ctrl Pts',(3.44133591342967,-2.21612800279508,4.40002410151124));
#20628=CARTESIAN_POINT('Ctrl Pts',(3.66843098386609,-2.16697244123634,4.38891031245443));
#20629=CARTESIAN_POINT('Ctrl Pts',(3.83289206448147,-2.33111753521892,4.37779652339763));
#20630=CARTESIAN_POINT('Ctrl Pts',(3.7841810615649,-2.55829573402952,4.36668273434082));
#20631=CARTESIAN_POINT('Ctrl Pts',(3.56689372435994,-2.6406156849541,4.35556894528403));
#20632=CARTESIAN_POINT('Ctrl Pts',(3.37989555580985,-2.50263402103458,4.34445515622721));
#20633=CARTESIAN_POINT('Ctrl Pts',(3.39438832834916,-2.27083719950648,4.33334136717041));
#20634=CARTESIAN_POINT('Ctrl Pts',(3.59702530195382,-2.15700945407857,4.32222757811361));
#20635=CARTESIAN_POINT('Ctrl Pts',(3.80250230755732,-2.26611609660926,4.31111378905681));
#20636=CARTESIAN_POINT('Ctrl Pts',(3.81563717950601,-2.41972137435598,4.30370459635227));
#20637=CARTESIAN_POINT('Ctrl Pts',(3.78826275096636,-2.48232321801033,4.3));
#20638=CARTESIAN_POINT('Ctrl Pts',(3.72690708798524,-2.29206413469515,5.2));
#20639=CARTESIAN_POINT('Ctrl Pts',(3.73511889692415,-2.29972488088976,5.2));
#20640=CARTESIAN_POINT('Ctrl Pts',(3.74243606331987,-2.3082260358574,5.2));
#20641=CARTESIAN_POINT('Ctrl Pts',(3.74885415883116,-2.3173733937361,5.2));
#20642=CARTESIAN_POINT('Ctrl Pts',(3.75362492547366,-2.32417290455016,5.2));
#20643=CARTESIAN_POINT('Ctrl Pts',(3.75789857922842,-2.33133076203089,5.2));
#20644=CARTESIAN_POINT('Ctrl Pts',(3.7616631192462,-2.3387816278666,5.2));
#20645=CARTESIAN_POINT('Ctrl Pts',(3.76388041855661,-2.34317015863036,5.2));
#20646=CARTESIAN_POINT('Ctrl Pts',(3.76592248852987,-2.34766555277529,5.2));
#20647=CARTESIAN_POINT('Ctrl Pts',(3.76777441807103,-2.35222602465318,5.2));
#20648=CARTESIAN_POINT('Ctrl Pts',(3.77233274722043,-2.36345114495818,5.2));
#20649=CARTESIAN_POINT('Ctrl Pts',(3.77575806540191,-2.37509440908006,5.2));
#20650=CARTESIAN_POINT('Ctrl Pts',(3.77802228391775,-2.38695732035888,5.2));
#20651=CARTESIAN_POINT('Ctrl Pts',(3.77946116292117,-2.39449603353478,5.2));
#20652=CARTESIAN_POINT('Ctrl Pts',(3.78043041033378,-2.40212433051409,5.2));
#20653=CARTESIAN_POINT('Ctrl Pts',(3.78091325285907,-2.40979638894873,5.2));
#20654=CARTESIAN_POINT('Ctrl Pts',(3.78113857897669,-2.41337667662164,5.2));
#20655=CARTESIAN_POINT('Ctrl Pts',(3.78125743502661,-2.41696304534708,5.2));
#20656=CARTESIAN_POINT('Ctrl Pts',(3.78126867486757,-2.42054069500775,5.2));
#20657=CARTESIAN_POINT('Ctrl Pts',(3.78130372190818,-2.4316961938677,5.2));
#20658=CARTESIAN_POINT('Ctrl Pts',(3.78029682789473,-2.44279407568189,5.2));
#20659=CARTESIAN_POINT('Ctrl Pts',(3.77821427386403,-2.45369318996624,5.2));
#20660=CARTESIAN_POINT('Ctrl Pts',(3.77705389172366,-2.45976608765585,5.2));
#20661=CARTESIAN_POINT('Ctrl Pts',(3.77555901526444,-2.46577751393184,5.2));
#20662=CARTESIAN_POINT('Ctrl Pts',(3.77374837416276,-2.47171132791926,5.2));
#20663=CARTESIAN_POINT('Ctrl Pts',(3.77261573055045,-2.47542321566067,5.2));
#20664=CARTESIAN_POINT('Ctrl Pts',(3.77135887218697,-2.47910625090944,5.2));
#20665=CARTESIAN_POINT('Ctrl Pts',(3.76998349987259,-2.48275161867489,5.2));
#20666=CARTESIAN_POINT('Ctrl Pts',(3.76560171320323,-2.49436536406777,5.2));
#20667=CARTESIAN_POINT('Ctrl Pts',(3.76005261276,-2.50551619028979,5.2));
#20668=CARTESIAN_POINT('Ctrl Pts',(3.75350161664164,-2.51608155564839,5.2));
#20669=CARTESIAN_POINT('Ctrl Pts',(3.74916064083137,-2.52308262764107,5.2));
#20670=CARTESIAN_POINT('Ctrl Pts',(3.7443785440277,-2.5298267716061,5.2));
#20671=CARTESIAN_POINT('Ctrl Pts',(3.73919190918146,-2.53627611456138,5.2));
#20672=CARTESIAN_POINT('Ctrl Pts',(3.73648178297727,-2.53964603241007,5.2));
#20673=CARTESIAN_POINT('Ctrl Pts',(3.73365980796544,-2.54293677988309,5.2));
#20674=CARTESIAN_POINT('Ctrl Pts',(3.73073436285314,-2.54613815029323,5.2));
#20675=CARTESIAN_POINT('Ctrl Pts',(3.72446793550896,-2.55299562131278,5.2));
#20676=CARTESIAN_POINT('Ctrl Pts',(3.71775196798206,-2.55941733778444,5.2));
#20677=CARTESIAN_POINT('Ctrl Pts',(3.71064054370859,-2.56535254658103,5.2));
#20678=CARTESIAN_POINT('Ctrl Pts',(3.70611395375814,-2.56913044752735,5.2));
#20679=CARTESIAN_POINT('Ctrl Pts',(3.70142688925274,-2.57271116046832,5.2));
#20680=CARTESIAN_POINT('Ctrl Pts',(3.69659110235036,-2.57608017868915,5.2));
#20681=CARTESIAN_POINT('Ctrl Pts',(3.69251867261816,-2.57891737773199,5.2));
#20682=CARTESIAN_POINT('Ctrl Pts',(3.68834776817108,-2.58159940125718,5.2));
#20683=CARTESIAN_POINT('Ctrl Pts',(3.68408920348942,-2.58411662981112,5.2));
#20684=CARTESIAN_POINT('Ctrl Pts',(3.67536613625436,-2.58927281635833,5.2));
#20685=CARTESIAN_POINT('Ctrl Pts',(3.6662720325658,-2.59374119323572,5.2));
#20686=CARTESIAN_POINT('Ctrl Pts',(3.65686566045376,-2.59744798255001,5.2));
#20687=CARTESIAN_POINT('Ctrl Pts',(3.6556263522049,-2.59793635942042,5.2));
#20688=CARTESIAN_POINT('Ctrl Pts',(3.65438160822106,-2.59841149615413,5.2));
#20689=CARTESIAN_POINT('Ctrl Pts',(3.65313161981588,-2.59887345085171,5.2));
#20690=CARTESIAN_POINT('Ctrl Pts',(3.43326718206005,-2.40013003210005,5.08714803633902));
#20691=CARTESIAN_POINT('Ctrl Pts',(3.4331940296057,-2.4086546125631,5.08771939403667));
#20692=CARTESIAN_POINT('Ctrl Pts',(3.43379133726061,-2.41716890764345,5.08829075173431));
#20693=CARTESIAN_POINT('Ctrl Pts',(3.43509475583067,-2.42557369055115,5.08886210943196));
#20694=CARTESIAN_POINT('Ctrl Pts',(3.44354592346175,-2.48006902373693,5.09256670578423));
#20695=CARTESIAN_POINT('Ctrl Pts',(3.48168219331808,-2.52996043426623,5.0962713021365));
#20696=CARTESIAN_POINT('Ctrl Pts',(3.53205035406398,-2.55241564805098,5.09997589848876));
#20697=CARTESIAN_POINT('Ctrl Pts',(3.58241851480988,-2.57487086183573,5.10368049484103));
#20698=CARTESIAN_POINT('Ctrl Pts',(3.64501856644536,-2.56988987887593,5.1073850911933));
#20699=CARTESIAN_POINT('Ctrl Pts',(3.69120110257795,-2.53975064654304,5.11108968754557));
#20700=CARTESIAN_POINT('Ctrl Pts',(3.73738363871054,-2.50961141421015,5.11479428389783));
#20701=CARTESIAN_POINT('Ctrl Pts',(3.76714865934026,-2.45431393250417,5.1184988802501));
#20702=CARTESIAN_POINT('Ctrl Pts',(3.76687430993005,-2.39916866701502,5.12220347660237));
#20703=CARTESIAN_POINT('Ctrl Pts',(3.76659996051984,-2.34402340152587,5.12590807295464));
#20704=CARTESIAN_POINT('Ctrl Pts',(3.73628624106972,-2.28903035225355,5.12961266930691));
#20705=CARTESIAN_POINT('Ctrl Pts',(3.68980584464362,-2.2593508727441,5.13331726565917));
#20706=CARTESIAN_POINT('Ctrl Pts',(3.64332544821752,-2.22967139323465,5.13702186201144));
#20707=CARTESIAN_POINT('Ctrl Pts',(3.58067837481544,-2.22530548348806,5.14072645836371));
#20708=CARTESIAN_POINT('Ctrl Pts',(3.53053651892971,-2.24826429864408,5.14443105471598));
#20709=CARTESIAN_POINT('Ctrl Pts',(3.48039466304398,-2.27122311380009,5.14813565106825));
#20710=CARTESIAN_POINT('Ctrl Pts',(3.4427580246746,-2.3215066538587,5.15184024742052));
#20711=CARTESIAN_POINT('Ctrl Pts',(3.43484901415926,-2.37607618365869,5.15554484377278));
#20712=CARTESIAN_POINT('Ctrl Pts',(3.4337081191144,-2.3839479782439,5.15607924129486));
#20713=CARTESIAN_POINT('Ctrl Pts',(3.43318582039731,-2.39190895914184,5.15661363881694));
#20714=CARTESIAN_POINT('Ctrl Pts',(3.43325215766083,-2.39987843114813,5.15714803633902));
#20715=CARTESIAN_POINT('Ctrl Pts',(3.54698297828114,-2.59851743256717,5.2));
#20716=CARTESIAN_POINT('Ctrl Pts',(3.48097120902544,-2.58088801151799,5.19629540364773));
#20717=CARTESIAN_POINT('Ctrl Pts',(3.36906717021742,-2.4748477879482,5.1888862109432));
#20718=CARTESIAN_POINT('Ctrl Pts',(3.41187708350278,-2.24617201703375,5.17777242188639));
#20719=CARTESIAN_POINT('Ctrl Pts',(3.62721323091929,-2.15871475485289,5.16665863282959));
#20720=CARTESIAN_POINT('Ctrl Pts',(3.81747535364037,-2.29190664293025,5.15554484377279));
#20721=CARTESIAN_POINT('Ctrl Pts',(3.80876232171537,-2.52413791100821,5.14443105471598));
#20722=CARTESIAN_POINT('Ctrl Pts',(3.60892556988421,-2.64269428158759,5.13331726565918));
#20723=CARTESIAN_POINT('Ctrl Pts',(3.40093972078443,-2.539134825312,5.12220347660237));
#20724=CARTESIAN_POINT('Ctrl Pts',(3.37514572416652,-2.30821119768585,5.11108968754557));
#20725=CARTESIAN_POINT('Ctrl Pts',(3.55516853033383,-2.16130913937078,5.09997589848876));
#20726=CARTESIAN_POINT('Ctrl Pts',(3.77622352465696,-2.23288041708187,5.08886210943196));
#20727=CARTESIAN_POINT('Ctrl Pts',(3.83598040928192,-2.457419700552,5.07774832037515));
#20728=CARTESIAN_POINT('Ctrl Pts',(3.67974110927284,-2.62940130358481,5.06663453131835));
#20729=CARTESIAN_POINT('Ctrl Pts',(3.45051418720664,-2.59140968013522,5.05552074226155));
#20730=CARTESIAN_POINT('Ctrl Pts',(3.35811316524308,-2.37821841178234,5.04440695320474));
#20731=CARTESIAN_POINT('Ctrl Pts',(3.48711398605093,-2.18496417501817,5.03329316414794));
#20732=CARTESIAN_POINT('Ctrl Pts',(3.71944061581356,-2.18853461914439,5.02217937509113));
#20733=CARTESIAN_POINT('Ctrl Pts',(3.84244191526684,-2.38566174871763,5.01106558603433));
#20734=CARTESIAN_POINT('Ctrl Pts',(3.74353337026135,-2.59591283022398,4.99995179697752));
#20735=CARTESIAN_POINT('Ctrl Pts',(3.51324710863985,-2.62684268245385,4.98883800792072));
#20736=CARTESIAN_POINT('Ctrl Pts',(3.36236674984584,-2.4501408518507,4.97772421886391));
#20737=CARTESIAN_POINT('Ctrl Pts',(3.42899480110061,-2.22754453241715,4.96661042980712));
#20738=CARTESIAN_POINT('Ctrl Pts',(3.65214584962031,-2.16279865748873,4.9554966407503));
#20739=CARTESIAN_POINT('Ctrl Pts',(3.82756721091734,-2.31516586178242,4.94438285169351));
#20740=CARTESIAN_POINT('Ctrl Pts',(3.79469372311971,-2.54518271468373,4.9332690626367));
#20741=CARTESIAN_POINT('Ctrl Pts',(3.58361486265069,-2.64231218244471,4.9221552735799));
#20742=CARTESIAN_POINT('Ctrl Pts',(3.38753350417909,-2.51765056156021,4.91104148452309));
#20743=CARTESIAN_POINT('Ctrl Pts',(3.38592513888554,-2.28530204745491,4.89992769546629));
#20744=CARTESIAN_POINT('Ctrl Pts',(3.5802619217345,-2.1579378700657,4.88881390640948));
#20745=CARTESIAN_POINT('Ctrl Pts',(3.7926651914697,-2.25213590538246,4.87770011735268));
#20746=CARTESIAN_POINT('Ctrl Pts',(3.8287198264784,-2.48167562339262,4.86658632829587));
#20747=CARTESIAN_POINT('Ctrl Pts',(3.65542461045338,-2.63645671704841,4.85547253923907));
#20748=CARTESIAN_POINT('Ctrl Pts',(3.43139861992193,-2.5748062959875,4.84435875018227));
#20749=CARTESIAN_POINT('Ctrl Pts',(3.36169538464595,-2.35315368977137,4.83324496112546));
#20750=CARTESIAN_POINT('Ctrl Pts',(3.51011506636152,-2.17438004258061,4.82213117206865));
#20751=CARTESIAN_POINT('Ctrl Pts',(3.74080744720095,-2.20211890112026,4.81101738301186));
#20752=CARTESIAN_POINT('Ctrl Pts',(3.84261717475225,-2.41098057358878,4.79990359395505));
#20753=CARTESIAN_POINT('Ctrl Pts',(3.72235665078693,-2.60979160252334,4.78878980489825));
#20754=CARTESIAN_POINT('Ctrl Pts',(3.49010169673754,-2.61657799846968,4.77767601584144));
#20755=CARTESIAN_POINT('Ctrl Pts',(3.3584379059958,-2.42512809625518,4.76656222678464));
#20756=CARTESIAN_POINT('Ctrl Pts',(3.44787863939658,-2.21067816256631,4.75544843772783));
#20757=CARTESIAN_POINT('Ctrl Pts',(3.67655777933124,-2.16951665373617,4.74433464867103));
#20758=CARTESIAN_POINT('Ctrl Pts',(3.83516271561975,-2.33931916560024,4.73322085961422));
#20759=CARTESIAN_POINT('Ctrl Pts',(3.77852055137491,-2.56466353335787,4.72210707055742));
#20760=CARTESIAN_POINT('Ctrl Pts',(3.55847650189588,-2.63928950162157,4.71099328150062));
#20761=CARTESIAN_POINT('Ctrl Pts',(3.37643938114003,-2.49489107532353,4.69987949244381));
#20762=CARTESIAN_POINT('Ctrl Pts',(3.39902983017658,-2.26363777164387,4.68876570338701));
#20763=CARTESIAN_POINT('Ctrl Pts',(3.60557055480924,-2.15719836203143,4.6776519143302));
#20764=CARTESIAN_POINT('Ctrl Pts',(3.8070124874506,-2.27299804520947,4.6665381252734));
#20765=CARTESIAN_POINT('Ctrl Pts',(3.81897354264718,-2.50504405790744,4.65542433621659));
#20766=CARTESIAN_POINT('Ctrl Pts',(3.63050563092984,-2.64094205312202,4.64431054715979));
#20767=CARTESIAN_POINT('Ctrl Pts',(3.4141155692652,-2.55630305464544,4.63319675810298));
#20768=CARTESIAN_POINT('Ctrl Pts',(3.3678676351246,-2.32859809765437,4.62208296904619));
#20769=CARTESIAN_POINT('Ctrl Pts',(3.53409308711521,-2.16624811163355,4.61096917998937));
#20770=CARTESIAN_POINT('Ctrl Pts',(3.76064388390312,-2.21785387995996,4.59985539093258));
#20771=CARTESIAN_POINT('Ctrl Pts',(3.8401555119317,-2.4361800576391,4.58874160187577));
#20772=CARTESIAN_POINT('Ctrl Pts',(3.69985007633495,-2.62139021824623,4.57762781281896));
#20773=CARTESIAN_POINT('Ctrl Pts',(3.46815073350293,-2.60395940136712,4.56651402376216));
#20774=CARTESIAN_POINT('Ctrl Pts',(3.35713451954606,-2.39984223133897,4.55540023470536));
#20775=CARTESIAN_POINT('Ctrl Pts',(3.46841583417461,-2.19586946879708,4.54428644564855));
#20776=CARTESIAN_POINT('Ctrl Pts',(3.70013762796088,-2.17873969637961,4.53317265659175));
#20777=CARTESIAN_POINT('Ctrl Pts',(3.84020231541317,-2.36413198929513,4.52205886753494));
#20778=CARTESIAN_POINT('Ctrl Pts',(3.7604070991348,-2.58235467884591,4.51094507847814));
#20779=CARTESIAN_POINT('Ctrl Pts',(3.53378944658573,-2.63366606347461,4.49983128942134));
#20780=CARTESIAN_POINT('Ctrl Pts',(3.36777506303883,-2.47110024891367,4.48871750036453));
#20781=CARTESIAN_POINT('Ctrl Pts',(3.41431880073856,-2.24345557286895,4.47760371130772));
#20782=CARTESIAN_POINT('Ctrl Pts',(3.63081864021225,-2.15909778094929,4.46648992225093));
#20783=CARTESIAN_POINT('Ctrl Pts',(3.81910984016012,-2.29524053287965,4.45537613319411));
#20784=CARTESIAN_POINT('Ctrl Pts',(3.80684729577664,-2.52727079162485,4.44426234413733));
#20785=CARTESIAN_POINT('Ctrl Pts',(3.60525512132335,-2.64280869447754,4.4331485550805));
#20786=CARTESIAN_POINT('Ctrl Pts',(3.39885278350865,-2.53610095948868,4.42203476602371));
#20787=CARTESIAN_POINT('Ctrl Pts',(3.37656295673162,-2.30481864526098,4.4109209769669));
#20788=CARTESIAN_POINT('Ctrl Pts',(3.55878722400007,-2.16065655916503,4.3998071879101));
#20789=CARTESIAN_POINT('Ctrl Pts',(3.77873474447839,-2.23556893008468,4.38869339885329));
#20790=CARTESIAN_POINT('Ctrl Pts',(3.83508286096032,-2.4609855401145,4.37757960979649));
#20791=CARTESIAN_POINT('Ctrl Pts',(3.67625990251943,-2.63058416437082,4.36646582073969));
#20792=CARTESIAN_POINT('Ctrl Pts',(3.44762951704948,-2.58912094093836,4.35535203168288));
#20793=CARTESIAN_POINT('Ctrl Pts',(3.35847732135144,-2.37456428079453,4.34423824262607));
#20794=CARTESIAN_POINT('Ctrl Pts',(3.49037003077072,-2.18326698967564,4.33312445356928));
#20795=CARTESIAN_POINT('Ctrl Pts',(3.72265543153543,-2.19039239422561,4.32201066451247));
#20796=CARTESIAN_POINT('Ctrl Pts',(3.84257847294968,-2.38928487404799,4.31089687545567));
#20797=CARTESIAN_POINT('Ctrl Pts',(3.74065691978671,-2.59816384879942,4.29978308639886));
#20798=CARTESIAN_POINT('Ctrl Pts',(3.50959628368763,-2.62529831625878,4.28866929734206));
#20799=CARTESIAN_POINT('Ctrl Pts',(3.41142456563631,-2.50643134569449,4.28126010463752));
#20800=CARTESIAN_POINT('Ctrl Pts',(3.39833241385534,-2.439372075429,4.27755550828525));
#20801=CARTESIAN_POINT('Ctrl Pts',(3.55032651029123,-2.58599788000028,5.20748149723825));
#20802=CARTESIAN_POINT('Ctrl Pts',(3.48847779011663,-2.5694802628904,5.20377690088598));
#20803=CARTESIAN_POINT('Ctrl Pts',(3.38363100808545,-2.4701274930924,5.19636770818144));
#20804=CARTESIAN_POINT('Ctrl Pts',(3.42374110325997,-2.25587321805223,5.18525391912464));
#20805=CARTESIAN_POINT('Ctrl Pts',(3.62549702156375,-2.17393147043888,5.17414013006783));
#20806=CARTESIAN_POINT('Ctrl Pts',(3.80376021494099,-2.29872357809039,5.16302634101103));
#20807=CARTESIAN_POINT('Ctrl Pts',(3.79559667259879,-2.51630912195772,5.15191255195423));
#20808=CARTESIAN_POINT('Ctrl Pts',(3.60836267654075,-2.62738870475875,5.14079876289742));
#20809=CARTESIAN_POINT('Ctrl Pts',(3.41349350811379,-2.53036025203219,5.12968497384062));
#20810=CARTESIAN_POINT('Ctrl Pts',(3.38932621647788,-2.31399988193773,5.11857118478382));
#20811=CARTESIAN_POINT('Ctrl Pts',(3.55799583841393,-2.17636223943479,5.10745739572701));
#20812=CARTESIAN_POINT('Ctrl Pts',(3.76510994308412,-2.24341985624469,5.09634360667021));
#20813=CARTESIAN_POINT('Ctrl Pts',(3.8210982445241,-2.45379851247728,5.0852298176134));
#20814=CARTESIAN_POINT('Ctrl Pts',(3.67471221585842,-2.61493405180745,5.0741160285566));
#20815=CARTESIAN_POINT('Ctrl Pts',(3.4599415481546,-2.57933837979007,5.0630022394998));
#20816=CARTESIAN_POINT('Ctrl Pts',(3.3733678202314,-2.37959207320419,5.05188845044299));
#20817=CARTESIAN_POINT('Ctrl Pts',(3.49423317134075,-2.19852546421989,5.04077466138618));
#20818=CARTESIAN_POINT('Ctrl Pts',(3.71190806288376,-2.20187073737575,5.02966087232939));
#20819=CARTESIAN_POINT('Ctrl Pts',(3.82715225398445,-2.38656599419535,5.01854708327258));
#20820=CARTESIAN_POINT('Ctrl Pts',(3.73448140162136,-2.58355753756882,5.00743329421578));
#20821=CARTESIAN_POINT('Ctrl Pts',(3.51871820188173,-2.61253679077134,4.99631950515897));
#20822=CARTESIAN_POINT('Ctrl Pts',(3.37735315143523,-2.44697870622763,4.98520571610217));
#20823=CARTESIAN_POINT('Ctrl Pts',(3.4397792876273,-2.23842048050862,4.97409192704536));
#20824=CARTESIAN_POINT('Ctrl Pts',(3.64885725830102,-2.17775782071235,4.96297813798855));
#20825=CARTESIAN_POINT('Ctrl Pts',(3.81321562666231,-2.3205159483675,4.95186434893175));
#20826=CARTESIAN_POINT('Ctrl Pts',(3.78241531376532,-2.53602672971665,4.94075055987495));
#20827=CARTESIAN_POINT('Ctrl Pts',(3.5846481955208,-2.62703070279587,4.92963677081815));
#20828=CARTESIAN_POINT('Ctrl Pts',(3.40093275798132,-2.51023089885891,4.91852298176134));
#20829=CARTESIAN_POINT('Ctrl Pts',(3.39942582465563,-2.29253550311487,4.90740919270454));
#20830=CARTESIAN_POINT('Ctrl Pts',(3.5815067086795,-2.17320358008914,4.89629540364773));
#20831=CARTESIAN_POINT('Ctrl Pts',(3.78051471198171,-2.26146099225962,4.88518161459093));
#20832=CARTESIAN_POINT('Ctrl Pts',(3.81429555222874,-2.47652472935135,4.87406782553412));
#20833=CARTESIAN_POINT('Ctrl Pts',(3.65192924324508,-2.6215445138197,4.86295403647732));
#20834=CARTESIAN_POINT('Ctrl Pts',(3.44203150900096,-2.56378209230252,4.85184024742051));
#20835=CARTESIAN_POINT('Ctrl Pts',(3.37672412605308,-2.35610806428593,4.84072645836371));
#20836=CARTESIAN_POINT('Ctrl Pts',(3.5157836826493,-2.18860882279666,4.8296126693069));
#20837=CARTESIAN_POINT('Ctrl Pts',(3.73192738959469,-2.2145983231407,4.8184988802501));
#20838=CARTESIAN_POINT('Ctrl Pts',(3.82731646068567,-2.41028808091203,4.8073850911933));
#20839=CARTESIAN_POINT('Ctrl Pts',(3.71464019736706,-2.59656104154983,4.79627130213649));
#20840=CARTESIAN_POINT('Ctrl Pts',(3.49703246129012,-2.60291945170324,4.78515751307969));
#20841=CARTESIAN_POINT('Ctrl Pts',(3.37367208112564,-2.42354338644957,4.77404372402289));
#20842=CARTESIAN_POINT('Ctrl Pts',(3.45747221184004,-2.22261779257846,4.76292993496608));
#20843=CARTESIAN_POINT('Ctrl Pts',(3.6717296434323,-2.18405214481133,4.75181614590928));
#20844=CARTESIAN_POINT('Ctrl Pts',(3.8203321189215,-2.34314601791364,4.74070235685247));
#20845=CARTESIAN_POINT('Ctrl Pts',(3.76726210722566,-2.55427898558761,4.72958856779567));
#20846=CARTESIAN_POINT('Ctrl Pts',(3.56109519190488,-2.62419864811054,4.71847477873887));
#20847=CARTESIAN_POINT('Ctrl Pts',(3.39053828864408,-2.4889067454323,4.70736098968206));
#20848=CARTESIAN_POINT('Ctrl Pts',(3.41170406524473,-2.2722374903888,4.69624720062525));
#20849=CARTESIAN_POINT('Ctrl Pts',(3.60521924634802,-2.17251070931785,4.68513341156845));
#20850=CARTESIAN_POINT('Ctrl Pts',(3.79395719207867,-2.28100745591228,4.67401962251165));
#20851=CARTESIAN_POINT('Ctrl Pts',(3.80516392027559,-2.49841942757747,4.66290583345484));
#20852=CARTESIAN_POINT('Ctrl Pts',(3.62858178552708,-2.6257469810287,4.65179204439804));
#20853=CARTESIAN_POINT('Ctrl Pts',(3.4258384183463,-2.54644576259963,4.64067825534124));
#20854=CARTESIAN_POINT('Ctrl Pts',(3.3825071219795,-2.3331010768549,4.62956446628443));
#20855=CARTESIAN_POINT('Ctrl Pts',(3.53824952340251,-2.18098973415088,4.61845067722763));
#20856=CARTESIAN_POINT('Ctrl Pts',(3.75051283635195,-2.22934097152269,4.60733688817082));
#20857=CARTESIAN_POINT('Ctrl Pts',(3.82501004325936,-2.43389835306723,4.59622309911402));
#20858=CARTESIAN_POINT('Ctrl Pts',(3.69355300577889,-2.607428187611,4.58510931005722));
#20859=CARTESIAN_POINT('Ctrl Pts',(3.47646584115605,-2.59109664964851,4.57399552100041));
#20860=CARTESIAN_POINT('Ctrl Pts',(3.37245089307511,-2.39985218105986,4.56288173194361));
#20861=CARTESIAN_POINT('Ctrl Pts',(3.47671422318619,-2.20874301286248,4.5517679428868));
#20862=CARTESIAN_POINT('Ctrl Pts',(3.69382242288812,-2.1926935339158,4.54065415383));
#20863=CARTESIAN_POINT('Ctrl Pts',(3.82505389506733,-2.36639401454743,4.52954036477319));
#20864=CARTESIAN_POINT('Ctrl Pts',(3.75029098447549,-2.57085443446884,4.51842657571639));
#20865=CARTESIAN_POINT('Ctrl Pts',(3.53796503204054,-2.61892985352599,4.50731278665959));
#20866=CARTESIAN_POINT('Ctrl Pts',(3.38242038797595,-2.46661629356384,4.49619899760278));
#20867=CARTESIAN_POINT('Ctrl Pts',(3.42602883297491,-2.25332808713219,4.48508520854598));
#20868=CARTESIAN_POINT('Ctrl Pts',(3.62887505479918,-2.17429034089672,4.47397141948917));
#20869=CARTESIAN_POINT('Ctrl Pts',(3.80529162215107,-2.30184721541898,4.46285763043237));
#20870=CARTESIAN_POINT('Ctrl Pts',(3.7938024182598,-2.51924442665844,4.45174384137557));
#20871=CARTESIAN_POINT('Ctrl Pts',(3.60492370575545,-2.62749590217058,4.44063005231876));
#20872=CARTESIAN_POINT('Ctrl Pts',(3.41153818407012,-2.52751771773158,4.42951626326196));
#20873=CARTESIAN_POINT('Ctrl Pts',(3.39065407090943,-2.31082128169766,4.41840247420515));
#20874=CARTESIAN_POINT('Ctrl Pts',(3.56138631824024,-2.17575081436632,4.40728868514835));
#20875=CARTESIAN_POINT('Ctrl Pts',(3.76746279218639,-2.24593881748859,4.39617489609154));
#20876=CARTESIAN_POINT('Ctrl Pts',(3.82025730031655,-2.4571394714574,4.38506110703474));
#20877=CARTESIAN_POINT('Ctrl Pts',(3.67145055229768,-2.61604231517601,4.37394731797793));
#20878=CARTESIAN_POINT('Ctrl Pts',(3.45723880045736,-2.57719398051498,4.36283352892113));
#20879=CARTESIAN_POINT('Ctrl Pts',(3.37370901074182,-2.37616839092003,4.35171973986433));
#20880=CARTESIAN_POINT('Ctrl Pts',(3.49728387276899,-2.19693531230428,4.34060595080752));
#20881=CARTESIAN_POINT('Ctrl Pts',(3.71492013543138,-2.20361135139717,4.32949216175072));
#20882=CARTESIAN_POINT('Ctrl Pts',(3.82728019962215,-2.38996062620176,4.31837837269391));
#20883=CARTESIAN_POINT('Ctrl Pts',(3.73178635523027,-2.58566659508311,4.30726458363711));
#20884=CARTESIAN_POINT('Ctrl Pts',(3.51529761713718,-2.61108982042464,4.29615079458031));
#20885=CARTESIAN_POINT('Ctrl Pts',(3.42331712354828,-2.49971922570605,4.28874160187577));
#20886=CARTESIAN_POINT('Ctrl Pts',(3.41105063166184,-2.43688906544027,4.2850370055235));
#20887=CARTESIAN_POINT('Ctrl Pts',(3.55367004230132,-2.57347832743338,5.2149629944765));
#20888=CARTESIAN_POINT('Ctrl Pts',(3.49598437120782,-2.55807251426281,5.21125839812423));
#20889=CARTESIAN_POINT('Ctrl Pts',(3.39819484595347,-2.4654071982366,5.2038492054197));
#20890=CARTESIAN_POINT('Ctrl Pts',(3.43560512301717,-2.2655744190707,5.19273541636288));
#20891=CARTESIAN_POINT('Ctrl Pts',(3.62378081220822,-2.18914818602487,5.18162162730609));
#20892=CARTESIAN_POINT('Ctrl Pts',(3.7900450762416,-2.30554051325052,5.17050783824928));
#20893=CARTESIAN_POINT('Ctrl Pts',(3.78243102348222,-2.50848033290724,5.15939404919248));
#20894=CARTESIAN_POINT('Ctrl Pts',(3.60779978319727,-2.6120831279299,5.14828026013567));
#20895=CARTESIAN_POINT('Ctrl Pts',(3.42604729544316,-2.52158567875239,5.13716647107887));
#20896=CARTESIAN_POINT('Ctrl Pts',(3.40350670878923,-2.3197885661896,5.12605268202206));
#20897=CARTESIAN_POINT('Ctrl Pts',(3.56082314649402,-2.19141533949881,5.11493889296526));
#20898=CARTESIAN_POINT('Ctrl Pts',(3.75399636151128,-2.25395929540751,5.10382510390846));
#20899=CARTESIAN_POINT('Ctrl Pts',(3.80621607976629,-2.45017732440257,5.09271131485166));
#20900=CARTESIAN_POINT('Ctrl Pts',(3.66968332244401,-2.60046680003009,5.08159752579485));
#20901=CARTESIAN_POINT('Ctrl Pts',(3.46936890910255,-2.56726707944493,5.07048373673804));
#20902=CARTESIAN_POINT('Ctrl Pts',(3.38862247521972,-2.38096573462603,5.05936994768124));
#20903=CARTESIAN_POINT('Ctrl Pts',(3.50135235663055,-2.21208675342161,5.04825615862443));
#20904=CARTESIAN_POINT('Ctrl Pts',(3.70437550995396,-2.2152068556071,5.03714236956763));
#20905=CARTESIAN_POINT('Ctrl Pts',(3.81186259270206,-2.38747023967307,5.02602858051083));
#20906=CARTESIAN_POINT('Ctrl Pts',(3.72542943298136,-2.57120224491366,5.01491479145402));
#20907=CARTESIAN_POINT('Ctrl Pts',(3.52418929512361,-2.59823089908883,5.00380100239722));
#20908=CARTESIAN_POINT('Ctrl Pts',(3.39233955302463,-2.44381656060457,4.99268721334042));
#20909=CARTESIAN_POINT('Ctrl Pts',(3.45056377415398,-2.24929642860009,4.98157342428361));
#20910=CARTESIAN_POINT('Ctrl Pts',(3.64556866698174,-2.19271698393598,4.97045963522681));
#20911=CARTESIAN_POINT('Ctrl Pts',(3.79886404240727,-2.32586603495258,4.95934584617));
#20912=CARTESIAN_POINT('Ctrl Pts',(3.77013690441093,-2.52687074474958,4.9482320571132));
#20913=CARTESIAN_POINT('Ctrl Pts',(3.58568152839091,-2.61174922314702,4.93711826805639));
#20914=CARTESIAN_POINT('Ctrl Pts',(3.41433201178354,-2.5028112361576,4.92600447899959));
#20915=CARTESIAN_POINT('Ctrl Pts',(3.41292651042572,-2.29976895877483,4.91489068994279));
#20916=CARTESIAN_POINT('Ctrl Pts',(3.58275149562449,-2.18846929011257,4.90377690088598));
#20917=CARTESIAN_POINT('Ctrl Pts',(3.76836423249372,-2.27078607913679,4.89266311182918));
#20918=CARTESIAN_POINT('Ctrl Pts',(3.79987127797908,-2.47137383531008,4.88154932277237));
#20919=CARTESIAN_POINT('Ctrl Pts',(3.64843387603678,-2.60663231059099,4.87043553371557));
#20920=CARTESIAN_POINT('Ctrl Pts',(3.45266439807998,-2.55275788861754,4.85932174465877));
#20921=CARTESIAN_POINT('Ctrl Pts',(3.39175286746021,-2.35906243880049,4.84820795560196));
#20922=CARTESIAN_POINT('Ctrl Pts',(3.52145229893708,-2.20283760301271,4.83709416654516));
#20923=CARTESIAN_POINT('Ctrl Pts',(3.72304733198844,-2.22707774516114,4.82598037748835));
#20924=CARTESIAN_POINT('Ctrl Pts',(3.81201574661908,-2.40959558823528,4.81486658843155));
#20925=CARTESIAN_POINT('Ctrl Pts',(3.7069237439472,-2.58333048057632,4.80375279937474));
#20926=CARTESIAN_POINT('Ctrl Pts',(3.50396322584271,-2.58926090493679,4.79263901031794));
#20927=CARTESIAN_POINT('Ctrl Pts',(3.38890625625548,-2.42195867664397,4.78152522126113));
#20928=CARTESIAN_POINT('Ctrl Pts',(3.46706578428349,-2.2345574225906,4.77041143220433));
#20929=CARTESIAN_POINT('Ctrl Pts',(3.66690150753336,-2.19858763588649,4.75929764314752));
#20930=CARTESIAN_POINT('Ctrl Pts',(3.80550152222325,-2.34697287022705,4.74818385409073));
#20931=CARTESIAN_POINT('Ctrl Pts',(3.75600366307642,-2.54389443781734,4.73707006503391));
#20932=CARTESIAN_POINT('Ctrl Pts',(3.56371388191388,-2.60910779459951,4.72595627597711));
#20933=CARTESIAN_POINT('Ctrl Pts',(3.40463719614813,-2.48292241554106,4.71484248692031));
#20934=CARTESIAN_POINT('Ctrl Pts',(3.42437830031288,-2.28083720913373,4.7037286978635));
#20935=CARTESIAN_POINT('Ctrl Pts',(3.60486793788679,-2.18782305660426,4.6926149088067));
#20936=CARTESIAN_POINT('Ctrl Pts',(3.78090189670674,-2.28901686661509,4.6815011197499));
#20937=CARTESIAN_POINT('Ctrl Pts',(3.79135429790399,-2.4917947972475,4.67038733069309));
#20938=CARTESIAN_POINT('Ctrl Pts',(3.62665794012432,-2.6105519089354,4.65927354163629));
#20939=CARTESIAN_POINT('Ctrl Pts',(3.43756126742739,-2.53658847055381,4.64815975257948));
#20940=CARTESIAN_POINT('Ctrl Pts',(3.3971466088344,-2.33760405605543,4.63704596352268));
#20941=CARTESIAN_POINT('Ctrl Pts',(3.54240595968981,-2.19573135666821,4.62593217446587));
#20942=CARTESIAN_POINT('Ctrl Pts',(3.74038178880077,-2.24082806308542,4.61481838540907));
#20943=CARTESIAN_POINT('Ctrl Pts',(3.80986457458702,-2.43161664849535,4.60370459635227));
#20944=CARTESIAN_POINT('Ctrl Pts',(3.68725593522283,-2.59346615697577,4.59259080729546));
#20945=CARTESIAN_POINT('Ctrl Pts',(3.48478094880917,-2.57823389792989,4.58147701823866));
#20946=CARTESIAN_POINT('Ctrl Pts',(3.38776726660417,-2.39986213078074,4.57036322918185));
#20947=CARTESIAN_POINT('Ctrl Pts',(3.48501261219776,-2.22161655692788,4.55924944012505));
#20948=CARTESIAN_POINT('Ctrl Pts',(3.68750721781536,-2.20664737145198,4.54813565106824));
#20949=CARTESIAN_POINT('Ctrl Pts',(3.80990547472148,-2.36865603979974,4.53702186201144));
#20950=CARTESIAN_POINT('Ctrl Pts',(3.74017486981618,-2.55935419009178,4.52590807295464));
#20951=CARTESIAN_POINT('Ctrl Pts',(3.54214061749534,-2.60419364357738,4.51479428389783));
#20952=CARTESIAN_POINT('Ctrl Pts',(3.39706571291307,-2.46213233821401,4.50368049484103));
#20953=CARTESIAN_POINT('Ctrl Pts',(3.43773886521125,-2.26320060139544,4.49256670578422));
#20954=CARTESIAN_POINT('Ctrl Pts',(3.62693146938611,-2.18948290084415,4.48145291672742));
#20955=CARTESIAN_POINT('Ctrl Pts',(3.79147340414203,-2.30845389795831,4.47033912767061));
#20956=CARTESIAN_POINT('Ctrl Pts',(3.78075754074296,-2.51121806169204,4.45922533861382));
#20957=CARTESIAN_POINT('Ctrl Pts',(3.60459229018754,-2.61218310986363,4.44811154955701));
#20958=CARTESIAN_POINT('Ctrl Pts',(3.42422358463158,-2.51893447597448,4.4369977605002));
#20959=CARTESIAN_POINT('Ctrl Pts',(3.40474518508724,-2.31682391813433,4.4258839714434));
#20960=CARTESIAN_POINT('Ctrl Pts',(3.56398541248042,-2.19084506956762,4.41477018238659));
#20961=CARTESIAN_POINT('Ctrl Pts',(3.75619083989438,-2.25630870489251,4.40365639332979));
#20962=CARTESIAN_POINT('Ctrl Pts',(3.80543173967279,-2.4532934028003,4.39254260427299));
#20963=CARTESIAN_POINT('Ctrl Pts',(3.66664120207593,-2.60150046598119,4.38142881521619));
#20964=CARTESIAN_POINT('Ctrl Pts',(3.46684808386524,-2.5652670200916,4.37031502615938));
#20965=CARTESIAN_POINT('Ctrl Pts',(3.3889407001322,-2.37777250104553,4.35920123710258));
#20966=CARTESIAN_POINT('Ctrl Pts',(3.50419771476727,-2.21060363493292,4.34808744804577));
#20967=CARTESIAN_POINT('Ctrl Pts',(3.70718483932733,-2.21683030856873,4.33697365898897));
#20968=CARTESIAN_POINT('Ctrl Pts',(3.81198192629463,-2.39063637835552,4.32585986993216));
#20969=CARTESIAN_POINT('Ctrl Pts',(3.72291579067381,-2.5731693413668,4.31474608087536));
#20970=CARTESIAN_POINT('Ctrl Pts',(3.52099895058674,-2.5968813245905,4.30363229181856));
#20971=CARTESIAN_POINT('Ctrl Pts',(3.43520968146025,-2.49300710571762,4.29622309911402));
#20972=CARTESIAN_POINT('Ctrl Pts',(3.42376884946835,-2.43440605545154,4.29251850276175));
#20973=CARTESIAN_POINT('Ctrl Pts',(3.55701357431141,-2.56095877486649,5.22244449171475));
#20974=CARTESIAN_POINT('Ctrl Pts',(3.50349095229901,-2.54666476563522,5.21873989536248));
#20975=CARTESIAN_POINT('Ctrl Pts',(3.41275868382149,-2.4606869033808,5.21133070265794));
#20976=CARTESIAN_POINT('Ctrl Pts',(3.44746914277437,-2.27527562008917,5.20021691360114));
#20977=CARTESIAN_POINT('Ctrl Pts',(3.62206460285268,-2.20436490161086,5.18910312454433));
#20978=CARTESIAN_POINT('Ctrl Pts',(3.77632993754221,-2.31235744841065,5.17798933548754));
#20979=CARTESIAN_POINT('Ctrl Pts',(3.76926537436564,-2.50065154385676,5.16687554643072));
#20980=CARTESIAN_POINT('Ctrl Pts',(3.6072368898538,-2.59677755110107,5.15576175737393));
#20981=CARTESIAN_POINT('Ctrl Pts',(3.43860108277253,-2.51281110547259,5.14464796831712));
#20982=CARTESIAN_POINT('Ctrl Pts',(3.41768720110058,-2.32557725044148,5.13353417926032));
#20983=CARTESIAN_POINT('Ctrl Pts',(3.56365045457412,-2.20646843956283,5.12242039020351));
#20984=CARTESIAN_POINT('Ctrl Pts',(3.74288277993844,-2.26449873457034,5.11130660114671));
#20985=CARTESIAN_POINT('Ctrl Pts',(3.79133391500848,-2.44655613632785,5.1001928120899));
#20986=CARTESIAN_POINT('Ctrl Pts',(3.66465442902959,-2.58599954825273,5.0890790230331));
#20987=CARTESIAN_POINT('Ctrl Pts',(3.4787962700505,-2.55519577909978,5.0779652339763));
#20988=CARTESIAN_POINT('Ctrl Pts',(3.40387713020803,-2.38233939604788,5.06685144491948));
#20989=CARTESIAN_POINT('Ctrl Pts',(3.50847154192036,-2.22564804262333,5.05573765586269));
#20990=CARTESIAN_POINT('Ctrl Pts',(3.69684295702416,-2.22854297383845,5.04462386680588));
#20991=CARTESIAN_POINT('Ctrl Pts',(3.79657293141967,-2.38837448515078,5.03351007774908));
#20992=CARTESIAN_POINT('Ctrl Pts',(3.71637746434136,-2.5588469522585,5.02239628869228));
#20993=CARTESIAN_POINT('Ctrl Pts',(3.52966038836549,-2.58392500740631,5.01128249963547));
#20994=CARTESIAN_POINT('Ctrl Pts',(3.40732595461402,-2.44065441498151,5.00016871057866));
#20995=CARTESIAN_POINT('Ctrl Pts',(3.46134826068067,-2.26017237669156,4.98905492152187));
#20996=CARTESIAN_POINT('Ctrl Pts',(3.64228007566245,-2.20767614715961,4.97794113246505));
#20997=CARTESIAN_POINT('Ctrl Pts',(3.78451245815223,-2.33121612153766,4.96682734340826));
#20998=CARTESIAN_POINT('Ctrl Pts',(3.75785849505654,-2.5177147597825,4.95571355435145));
#20999=CARTESIAN_POINT('Ctrl Pts',(3.58671486126101,-2.59646774349818,4.94459976529464));
#21000=CARTESIAN_POINT('Ctrl Pts',(3.42773126558577,-2.49539157345629,4.93348597623784));
#21001=CARTESIAN_POINT('Ctrl Pts',(3.4264271961958,-2.30700241443478,4.92237218718104));
#21002=CARTESIAN_POINT('Ctrl Pts',(3.5839962825695,-2.20373500013601,4.91125839812423));
#21003=CARTESIAN_POINT('Ctrl Pts',(3.75621375300573,-2.28011116601395,4.90014460906743));
#21004=CARTESIAN_POINT('Ctrl Pts',(3.78544700372942,-2.46622294126882,4.88903082001062));
#21005=CARTESIAN_POINT('Ctrl Pts',(3.64493850882848,-2.59172010736228,4.87791703095382));
#21006=CARTESIAN_POINT('Ctrl Pts',(3.463297287159,-2.54173368493256,4.86680324189701));
#21007=CARTESIAN_POINT('Ctrl Pts',(3.40678160886734,-2.36201681331505,4.85568945284021));
#21008=CARTESIAN_POINT('Ctrl Pts',(3.52712091522486,-2.21706638322876,4.8445756637834));
#21009=CARTESIAN_POINT('Ctrl Pts',(3.71416727438218,-2.23955716718158,4.8334618747266));
#21010=CARTESIAN_POINT('Ctrl Pts',(3.7967150325525,-2.40890309555853,4.8223480856698));
#21011=CARTESIAN_POINT('Ctrl Pts',(3.69920729052733,-2.57009991960281,4.81123429661299));
#21012=CARTESIAN_POINT('Ctrl Pts',(3.5108939903953,-2.57560235817033,4.80012050755619));
#21013=CARTESIAN_POINT('Ctrl Pts',(3.40414043138533,-2.42037396683837,4.78900671849938));
#21014=CARTESIAN_POINT('Ctrl Pts',(3.47665935672695,-2.24649705260274,4.77789292944258));
#21015=CARTESIAN_POINT('Ctrl Pts',(3.66207337163443,-2.21312312696165,4.76677914038577));
#21016=CARTESIAN_POINT('Ctrl Pts',(3.790670925525,-2.35079972254045,4.75566535132897));
#21017=CARTESIAN_POINT('Ctrl Pts',(3.74474521892717,-2.53350989004707,4.74455156227217));
#21018=CARTESIAN_POINT('Ctrl Pts',(3.56633257192288,-2.59401694108847,4.73343777321536));
#21019=CARTESIAN_POINT('Ctrl Pts',(3.41873610365217,-2.47693808564983,4.72232398415856));
#21020=CARTESIAN_POINT('Ctrl Pts',(3.43705253538103,-2.28943692787866,4.71121019510175));
#21021=CARTESIAN_POINT('Ctrl Pts',(3.60451662942557,-2.20313540389068,4.70009640604496));
#21022=CARTESIAN_POINT('Ctrl Pts',(3.76784660133481,-2.29702627731791,4.68898261698814));
#21023=CARTESIAN_POINT('Ctrl Pts',(3.7775446755324,-2.48517016691753,4.67786882793135));
#21024=CARTESIAN_POINT('Ctrl Pts',(3.62473409472155,-2.59535683684209,4.66675503887453));
#21025=CARTESIAN_POINT('Ctrl Pts',(3.44928411650849,-2.526731178508,4.65564124981774));
#21026=CARTESIAN_POINT('Ctrl Pts',(3.4117860956893,-2.34210703525596,4.64452746076092));
#21027=CARTESIAN_POINT('Ctrl Pts',(3.5465623959771,-2.21047297918554,4.63341367170413));
#21028=CARTESIAN_POINT('Ctrl Pts',(3.73025074124959,-2.25231515464815,4.62229988264732));
#21029=CARTESIAN_POINT('Ctrl Pts',(3.79471910591469,-2.42933494392347,4.61118609359052));
#21030=CARTESIAN_POINT('Ctrl Pts',(3.68095886466676,-2.57950412634054,4.60007230453372));
#21031=CARTESIAN_POINT('Ctrl Pts',(3.49309605646229,-2.56537114621128,4.5889585154769));
#21032=CARTESIAN_POINT('Ctrl Pts',(3.40308364013322,-2.39987208050163,4.57784472642011));
#21033=CARTESIAN_POINT('Ctrl Pts',(3.49331100120934,-2.23449010099328,4.56673093736329));
#21034=CARTESIAN_POINT('Ctrl Pts',(3.68119201274259,-2.22060120898816,4.5556171483065));
#21035=CARTESIAN_POINT('Ctrl Pts',(3.79475705437564,-2.37091806505204,4.54450335924969));
#21036=CARTESIAN_POINT('Ctrl Pts',(3.73005875515687,-2.5478539457147,4.53338957019289));
#21037=CARTESIAN_POINT('Ctrl Pts',(3.54631620295015,-2.58945743362876,4.52227578113609));
#21038=CARTESIAN_POINT('Ctrl Pts',(3.4117110378502,-2.45764838286418,4.51116199207927));
#21039=CARTESIAN_POINT('Ctrl Pts',(3.4494488974476,-2.27307311565868,4.50004820302248));
#21040=CARTESIAN_POINT('Ctrl Pts',(3.62498788397304,-2.20467546079158,4.48893441396567));
#21041=CARTESIAN_POINT('Ctrl Pts',(3.77765518613299,-2.31506058049763,4.47782062490887));
#21042=CARTESIAN_POINT('Ctrl Pts',(3.76771266322612,-2.50319169672563,4.46670683585206));
#21043=CARTESIAN_POINT('Ctrl Pts',(3.60426087461964,-2.59687031755667,4.45559304679526));
#21044=CARTESIAN_POINT('Ctrl Pts',(3.43690898519305,-2.51035123421737,4.44447925773846));
#21045=CARTESIAN_POINT('Ctrl Pts',(3.41883629926506,-2.32282655457101,4.43336546868165));
#21046=CARTESIAN_POINT('Ctrl Pts',(3.56658450672058,-2.20593932476892,4.42225167962485));
#21047=CARTESIAN_POINT('Ctrl Pts',(3.74491888760239,-2.26667859229642,4.41113789056804));
#21048=CARTESIAN_POINT('Ctrl Pts',(3.79060617902903,-2.4494473341432,4.40002410151123));
#21049=CARTESIAN_POINT('Ctrl Pts',(3.66183185185417,-2.58695861678637,4.38891031245443));
#21050=CARTESIAN_POINT('Ctrl Pts',(3.47645736727312,-2.55334005966823,4.37779652339763));
#21051=CARTESIAN_POINT('Ctrl Pts',(3.40417238952257,-2.37937661117104,4.36668273434082));
#21052=CARTESIAN_POINT('Ctrl Pts',(3.51111155676555,-2.22427195756156,4.35556894528402));
#21053=CARTESIAN_POINT('Ctrl Pts',(3.69944954322327,-2.2300492657403,4.34445515622722));
#21054=CARTESIAN_POINT('Ctrl Pts',(3.79668365296711,-2.39131213050928,4.33334136717041));
#21055=CARTESIAN_POINT('Ctrl Pts',(3.71404522611737,-2.56067208765049,4.32222757811361));
#21056=CARTESIAN_POINT('Ctrl Pts',(3.5267002840363,-2.58267282875636,4.31111378905681));
#21057=CARTESIAN_POINT('Ctrl Pts',(3.44710223937223,-2.48629498572918,4.30370459635227));
#21058=CARTESIAN_POINT('Ctrl Pts',(3.43648706727485,-2.43192304546281,4.3));
#21059=CARTESIAN_POINT('Ctrl Pts',(3.43361559198215,-2.39990578567643,5.13785196366098));
#21060=CARTESIAN_POINT('Ctrl Pts',(3.43350388051965,-2.378317282854,5.13641270219409));
#21061=CARTESIAN_POINT('Ctrl Pts',(3.43740296507651,-2.35676746744261,5.1349734407272));
#21062=CARTESIAN_POINT('Ctrl Pts',(3.44550005695817,-2.33693142446689,5.13353417926032));
#21063=CARTESIAN_POINT('Ctrl Pts',(3.4663416189251,-2.28587431348193,5.12982958290805));
#21064=CARTESIAN_POINT('Ctrl Pts',(3.51499603674961,-2.24617137652238,5.12612498655578));
#21065=CARTESIAN_POINT('Ctrl Pts',(3.56919529988925,-2.23599162387719,5.12242039020351));
#21066=CARTESIAN_POINT('Ctrl Pts',(3.62339456302889,-2.225811871232,5.11871579385124));
#21067=CARTESIAN_POINT('Ctrl Pts',(3.68313867148366,-2.24515530290117,5.11501119749898));
#21068=CARTESIAN_POINT('Ctrl Pts',(3.72108591488939,-2.28516991902867,5.11130660114671));
#21069=CARTESIAN_POINT('Ctrl Pts',(3.75903315829512,-2.32518453515617,5.10760200479444));
#21070=CARTESIAN_POINT('Ctrl Pts',(3.7751835366518,-2.38587033574201,5.10389740844217));
#21071=CARTESIAN_POINT('Ctrl Pts',(3.76214547816699,-2.43945380468907,5.1001928120899));
#21072=CARTESIAN_POINT('Ctrl Pts',(3.74910741968218,-2.49303727363614,5.09648821573763));
#21073=CARTESIAN_POINT('Ctrl Pts',(3.70688092435589,-2.53951841094443,5.09278361938536));
#21074=CARTESIAN_POINT('Ctrl Pts',(3.65479131686289,-2.55762501807309,5.0890790230331));
#21075=CARTESIAN_POINT('Ctrl Pts',(3.60270170936989,-2.57573162520175,5.08537442668083));
#21076=CARTESIAN_POINT('Ctrl Pts',(3.5407489897102,-2.56546370215076,5.08166983032856));
#21077=CARTESIAN_POINT('Ctrl Pts',(3.49728610657327,-2.53152034344996,5.0779652339763));
#21078=CARTESIAN_POINT('Ctrl Pts',(3.45773596902793,-2.50063273525474,5.07459414387119));
#21079=CARTESIAN_POINT('Ctrl Pts',(3.43349642418942,-2.45014057555659,5.07122305376608));
#21080=CARTESIAN_POINT('Ctrl Pts',(3.43317939237559,-2.39991359865598,5.06785196366098));
#21081=CARTESIAN_POINT('Ctrl Pts',(3.54698297828114,-2.59851743256717,5.2));
#21082=CARTESIAN_POINT('Ctrl Pts',(3.53457951946873,-2.59392489162072,5.2));
#21083=CARTESIAN_POINT('Ctrl Pts',(3.52273021669441,-2.5880656264448,5.2));
#21084=CARTESIAN_POINT('Ctrl Pts',(3.51155282078554,-2.58110287559691,5.2));
#21085=CARTESIAN_POINT('Ctrl Pts',(3.50588661273558,-2.57757321670087,5.2));
#21086=CARTESIAN_POINT('Ctrl Pts',(3.50039351027032,-2.5737592340707,5.2));
#21087=CARTESIAN_POINT('Ctrl Pts',(3.49509228904167,-2.56967861696227,5.2));
#21088=CARTESIAN_POINT('Ctrl Pts',(3.4905050126104,-2.5661475591401,5.2));
#21089=CARTESIAN_POINT('Ctrl Pts',(3.48606143928385,-2.56241679614242,5.2));
#21090=CARTESIAN_POINT('Ctrl Pts',(3.48177554227615,-2.55849690369355,5.2));
#21091=CARTESIAN_POINT('Ctrl Pts',(3.47866533036506,-2.55565229586402,5.2));
#21092=CARTESIAN_POINT('Ctrl Pts',(3.47564434245519,-2.5527135073757,5.2));
#21093=CARTESIAN_POINT('Ctrl Pts',(3.47272197556915,-2.54969075241385,5.2));
#21094=CARTESIAN_POINT('Ctrl Pts',(3.4637769959157,-2.54043849809891,5.2));
#21095=CARTESIAN_POINT('Ctrl Pts',(3.45573629551605,-2.5303863939551,5.2));
#21096=CARTESIAN_POINT('Ctrl Pts',(3.44873891503949,-2.51966547725229,5.2));
#21097=CARTESIAN_POINT('Ctrl Pts',(3.44420807340926,-2.51272362581603,5.2));
#21098=CARTESIAN_POINT('Ctrl Pts',(3.44011549441187,-2.50550078770205,5.2));
#21099=CARTESIAN_POINT('Ctrl Pts',(3.43651065828778,-2.49802988469159,5.2));
#21100=CARTESIAN_POINT('Ctrl Pts',(3.43484392828386,-2.49457564217533,5.2));
#21101=CARTESIAN_POINT('Ctrl Pts',(3.43328559790363,-2.49107645830187,5.2));
#21102=CARTESIAN_POINT('Ctrl Pts',(3.43184079842385,-2.48753928615204,5.2));
#21103=CARTESIAN_POINT('Ctrl Pts',(3.4278386851231,-2.47774127341323,5.2));
#21104=CARTESIAN_POINT('Ctrl Pts',(3.42470153714545,-2.46764377419319,5.2));
#21105=CARTESIAN_POINT('Ctrl Pts',(3.42252346903458,-2.4573201729425,5.2));
#21106=CARTESIAN_POINT('Ctrl Pts',(3.42066967900374,-2.44853358404506,5.2));
#21107=CARTESIAN_POINT('Ctrl Pts',(3.41951138514856,-2.43958272486992,5.2));
#21108=CARTESIAN_POINT('Ctrl Pts',(3.4190359581172,-2.43054589510015,5.2));
#21109=CARTESIAN_POINT('Ctrl Pts',(3.41886681623208,-2.42733087718605,5.2));
#21110=CARTESIAN_POINT('Ctrl Pts',(3.41878446710974,-2.42410641682356,5.2));
#21111=CARTESIAN_POINT('Ctrl Pts',(3.4187879805801,-2.42088574908536,5.2));
#21112=CARTESIAN_POINT('Ctrl Pts',(3.41880075373106,-2.40917707615745,5.2));
#21113=CARTESIAN_POINT('Ctrl Pts',(3.41994281751926,-2.39748218187535,5.2));
#21114=CARTESIAN_POINT('Ctrl Pts',(3.42216878576612,-2.38597338048412,5.2));
#21115=CARTESIAN_POINT('Ctrl Pts',(3.42331180295367,-2.38006370148633,5.2));
#21116=CARTESIAN_POINT('Ctrl Pts',(3.4247413109463,-2.37420327369848,5.2));
#21117=CARTESIAN_POINT('Ctrl Pts',(3.42645509270942,-2.36841769265549,5.2));
#21118=CARTESIAN_POINT('Ctrl Pts',(3.42814232412983,-2.36272174330468,5.2));
#21119=CARTESIAN_POINT('Ctrl Pts',(3.430107844827,-2.35709290248798,5.2));
#21120=CARTESIAN_POINT('Ctrl Pts',(3.43233768211765,-2.35158848883877,5.2));
#21121=CARTESIAN_POINT('Ctrl Pts',(3.43579440103488,-2.34305548471816,5.2));
#21122=CARTESIAN_POINT('Ctrl Pts',(3.4398879741905,-2.33480787202203,5.2));
#21123=CARTESIAN_POINT('Ctrl Pts',(3.44460905895211,-2.32694151527758,5.2));
#21124=CARTESIAN_POINT('Ctrl Pts',(3.44702307993388,-2.32291922989401,5.2));
#21125=CARTESIAN_POINT('Ctrl Pts',(3.44960209197192,-2.31899653386197,5.2));
#21126=CARTESIAN_POINT('Ctrl Pts',(3.45233605539852,-2.31519993624376,5.2));
#21127=CARTESIAN_POINT('Ctrl Pts',(3.45777066118573,-2.30765301327221,5.2));
#21128=CARTESIAN_POINT('Ctrl Pts',(3.46382416246759,-2.30058959612096,5.2));
#21129=CARTESIAN_POINT('Ctrl Pts',(3.47049190863519,-2.29412081302041,5.2));
#21130=CARTESIAN_POINT('Ctrl Pts',(3.47127037804276,-2.29336557285059,5.2));
#21131=CARTESIAN_POINT('Ctrl Pts',(3.472057234472,-2.29261846360327,5.2));
#21132=CARTESIAN_POINT('Ctrl Pts',(3.47285232078577,-2.29187955100915,5.2));
#21133=CARTESIAN_POINT('Origin',(3.6,-2.4,4.7));
#21134=CARTESIAN_POINT('Origin',(-3.6,-2.4,4.3));
#21135=CARTESIAN_POINT('Ctrl Pts',(-3.76351293272515,-2.4319230454628,4.3));
#21136=CARTESIAN_POINT('Ctrl Pts',(-3.76286871316703,-2.44021936733959,
4.3));
#21137=CARTESIAN_POINT('Ctrl Pts',(-3.76155560816075,-2.4484297641735,4.3));
#21138=CARTESIAN_POINT('Ctrl Pts',(-3.75963220162413,-2.45650290122813,
4.3));
#21139=CARTESIAN_POINT('Ctrl Pts',(-3.75857027465495,-2.46096013988305,
4.3));
#21140=CARTESIAN_POINT('Ctrl Pts',(-3.75732202640333,-2.4653756041272,4.3));
#21141=CARTESIAN_POINT('Ctrl Pts',(-3.75589532148576,-2.46974082414556,
4.3));
#21142=CARTESIAN_POINT('Ctrl Pts',(-3.75435560354459,-2.47445182464518,
4.3));
#21143=CARTESIAN_POINT('Ctrl Pts',(-3.75261043098936,-2.47909640157799,
4.3));
#21144=CARTESIAN_POINT('Ctrl Pts',(-3.75067343320617,-2.48365784346818,
4.3));
#21145=CARTESIAN_POINT('Ctrl Pts',(-3.74745266086646,-2.49124244991258,
4.3));
#21146=CARTESIAN_POINT('Ctrl Pts',(-3.74370038620747,-2.49860287239871,
4.3));
#21147=CARTESIAN_POINT('Ctrl Pts',(-3.73945960595045,-2.50569089060563,
4.3));
#21148=CARTESIAN_POINT('Ctrl Pts',(-3.73760643937826,-2.50878826363795,
4.3));
#21149=CARTESIAN_POINT('Ctrl Pts',(-3.73566012601582,-2.511832700902,4.3));
#21150=CARTESIAN_POINT('Ctrl Pts',(-3.73363013483138,-2.51481171247594,
4.3));
#21151=CARTESIAN_POINT('Ctrl Pts',(-3.72675413466501,-2.52490224106299,
4.3));
#21152=CARTESIAN_POINT('Ctrl Pts',(-3.71890630233768,-2.53427022723708,
4.3));
#21153=CARTESIAN_POINT('Ctrl Pts',(-3.710220437496,-2.54276718643201,4.3));
#21154=CARTESIAN_POINT('Ctrl Pts',(-3.70599062580354,-2.54690500552178,
4.3));
#21155=CARTESIAN_POINT('Ctrl Pts',(-3.70156129932866,-2.55083607679561,
4.3));
#21156=CARTESIAN_POINT('Ctrl Pts',(-3.69694397352711,-2.55454119955382,
4.3));
#21157=CARTESIAN_POINT('Ctrl Pts',(-3.69303800092373,-2.55767550469228,
4.3));
#21158=CARTESIAN_POINT('Ctrl Pts',(-3.68899293859581,-2.56065058734466,
4.3));
#21159=CARTESIAN_POINT('Ctrl Pts',(-3.68484116924407,-2.56343733372212,
4.3));
#21160=CARTESIAN_POINT('Ctrl Pts',(-3.67976588279258,-2.56684396230261,
4.3));
#21161=CARTESIAN_POINT('Ctrl Pts',(-3.67452566755957,-2.56997445255576,
4.3));
#21162=CARTESIAN_POINT('Ctrl Pts',(-3.66913578324553,-2.57281068802155,
4.3));
#21163=CARTESIAN_POINT('Ctrl Pts',(-3.66156268589167,-2.57679576192101,
4.3));
#21164=CARTESIAN_POINT('Ctrl Pts',(-3.6536944302201,-2.58020053259861,4.3));
#21165=CARTESIAN_POINT('Ctrl Pts',(-3.64559780863821,-2.58304072868827,
4.3));
#21166=CARTESIAN_POINT('Ctrl Pts',(-3.63968764062526,-2.58511394353595,
4.3));
#21167=CARTESIAN_POINT('Ctrl Pts',(-3.633655561192,-2.58688612240617,4.3));
#21168=CARTESIAN_POINT('Ctrl Pts',(-3.6275253141649,-2.58835973744293,4.3));
#21169=CARTESIAN_POINT('Ctrl Pts',(-3.62399736219549,-2.58920780164787,
4.3));
#21170=CARTESIAN_POINT('Ctrl Pts',(-3.62044138799033,-2.58995568069818,
4.3));
#21171=CARTESIAN_POINT('Ctrl Pts',(-3.61687019594187,-2.59060310935882,
4.3));
#21172=CARTESIAN_POINT('Ctrl Pts',(-3.6053532973959,-2.59269103129053,4.3));
#21173=CARTESIAN_POINT('Ctrl Pts',(-3.5936552916365,-2.5937426794922,4.3));
#21174=CARTESIAN_POINT('Ctrl Pts',(-3.58193296271379,-2.5937913460953,4.3));
#21175=CARTESIAN_POINT('Ctrl Pts',(-3.57526861453522,-2.59381901390686,
4.3));
#21176=CARTESIAN_POINT('Ctrl Pts',(-3.56859601622939,-2.59352191446421,
4.3));
#21177=CARTESIAN_POINT('Ctrl Pts',(-3.56194230797419,-2.5929013482942,4.3));
#21178=CARTESIAN_POINT('Ctrl Pts',(-3.55784543918526,-2.59251924885793,
4.3));
#21179=CARTESIAN_POINT('Ctrl Pts',(-3.55375366053793,-2.59201412364595,
4.3));
#21180=CARTESIAN_POINT('Ctrl Pts',(-3.54967980921583,-2.59138661988454,
4.3));
#21181=CARTESIAN_POINT('Ctrl Pts',(-3.53642388866962,-2.5893447829725,4.3));
#21182=CARTESIAN_POINT('Ctrl Pts',(-3.52344434481125,-2.58602557270852,
4.3));
#21183=CARTESIAN_POINT('Ctrl Pts',(-3.51095537008143,-2.58146161840675,
4.3));
#21184=CARTESIAN_POINT('Ctrl Pts',(-3.50062243383895,-2.57768556394,4.3));
#21185=CARTESIAN_POINT('Ctrl Pts',(-3.49062430896861,-2.57305657702062,
4.3));
#21186=CARTESIAN_POINT('Ctrl Pts',(-3.48108410771908,-2.56756616374223,
4.3));
#21187=CARTESIAN_POINT('Ctrl Pts',(-3.47992982857924,-2.56690187277492,
4.3));
#21188=CARTESIAN_POINT('Ctrl Pts',(-3.47878226433178,-2.56622494144235,
4.3));
#21189=CARTESIAN_POINT('Ctrl Pts',(-3.47764149510761,-2.56553553810743,
4.3));
#21190=CARTESIAN_POINT('Ctrl Pts',(-3.41173724903364,-2.48232321801034,
4.3));
#21191=CARTESIAN_POINT('Ctrl Pts',(-3.40908132671273,-2.474270631223,4.3));
#21192=CARTESIAN_POINT('Ctrl Pts',(-3.40697195813618,-2.46606039521676,
4.3));
#21193=CARTESIAN_POINT('Ctrl Pts',(-3.40539675699364,-2.45774386680553,
4.3));
#21194=CARTESIAN_POINT('Ctrl Pts',(-3.40421043018009,-2.45148046311471,
4.3));
#21195=CARTESIAN_POINT('Ctrl Pts',(-3.40332727350005,-2.44515671203471,
4.3));
#21196=CARTESIAN_POINT('Ctrl Pts',(-3.40274510705531,-2.43879482091291,
4.3));
#21197=CARTESIAN_POINT('Ctrl Pts',(-3.40230912033401,-2.4340303758362,4.3));
#21198=CARTESIAN_POINT('Ctrl Pts',(-3.40204240567473,-2.42924590842869,
4.3));
#21199=CARTESIAN_POINT('Ctrl Pts',(-3.40194407560279,-2.42446300988855,
4.3));
#21200=CARTESIAN_POINT('Ctrl Pts',(-3.4017383892304,-2.41445816568562,4.3));
#21201=CARTESIAN_POINT('Ctrl Pts',(-3.40226690961593,-2.40444523502109,
4.3));
#21202=CARTESIAN_POINT('Ctrl Pts',(-3.40352193796024,-2.39451254861871,
4.3));
#21203=CARTESIAN_POINT('Ctrl Pts',(-3.40417749889618,-2.3893242345667,4.3));
#21204=CARTESIAN_POINT('Ctrl Pts',(-3.4050325722576,-2.38415490381948,4.3));
#21205=CARTESIAN_POINT('Ctrl Pts',(-3.40608153527603,-2.37904223030681,
4.3));
#21206=CARTESIAN_POINT('Ctrl Pts',(-3.40864847953637,-2.36653087604773,
4.3));
#21207=CARTESIAN_POINT('Ctrl Pts',(-3.41237572714265,-2.35432631626979,
4.3));
#21208=CARTESIAN_POINT('Ctrl Pts',(-3.41724961050618,-2.34261710559519,
4.3));
#21209=CARTESIAN_POINT('Ctrl Pts',(-3.41948718042203,-2.33724147889476,
4.3));
#21210=CARTESIAN_POINT('Ctrl Pts',(-3.42196704076708,-2.33197060519316,
4.3));
#21211=CARTESIAN_POINT('Ctrl Pts',(-3.42469079211682,-2.32682518779718,
4.3));
#21212=CARTESIAN_POINT('Ctrl Pts',(-3.42647141933207,-2.32346141883567,
4.3));
#21213=CARTESIAN_POINT('Ctrl Pts',(-3.42835738874669,-2.3201495667824,4.3));
#21214=CARTESIAN_POINT('Ctrl Pts',(-3.430346105223,-2.31690145647487,4.3));
#21215=CARTESIAN_POINT('Ctrl Pts',(-3.43461852095602,-2.30992344943073,
4.3));
#21216=CARTESIAN_POINT('Ctrl Pts',(-3.43934738846969,-2.3032660957291,4.3));
#21217=CARTESIAN_POINT('Ctrl Pts',(-3.44453058590951,-2.29698173842211,
4.3));
#21218=CARTESIAN_POINT('Ctrl Pts',(-3.4502359337428,-2.29006430092116,4.3));
#21219=CARTESIAN_POINT('Ctrl Pts',(-3.45649195144988,-2.28359849259699,
4.3));
#21220=CARTESIAN_POINT('Ctrl Pts',(-3.4632263722909,-2.27761731307503,4.3));
#21221=CARTESIAN_POINT('Ctrl Pts',(-3.46747035511976,-2.27384801742411,
4.3));
#21222=CARTESIAN_POINT('Ctrl Pts',(-3.47190450284819,-2.27027143263625,
4.3));
#21223=CARTESIAN_POINT('Ctrl Pts',(-3.47651159455371,-2.26689859050011,
4.3));
#21224=CARTESIAN_POINT('Ctrl Pts',(-3.4793251060266,-2.26483882467541,4.3));
#21225=CARTESIAN_POINT('Ctrl Pts',(-3.48219970787858,-2.26285776645565,
4.3));
#21226=CARTESIAN_POINT('Ctrl Pts',(-3.48512436737332,-2.26096157786103,
4.3));
#21227=CARTESIAN_POINT('Ctrl Pts',(-3.49373619954507,-2.25537813884111,
4.3));
#21228=CARTESIAN_POINT('Ctrl Pts',(-3.50279847994849,-2.25051611152294,
4.3));
#21229=CARTESIAN_POINT('Ctrl Pts',(-3.51220227087042,-2.24642657080492,
4.3));
#21230=CARTESIAN_POINT('Ctrl Pts',(-3.5210281717619,-2.24258834413989,4.3));
#21231=CARTESIAN_POINT('Ctrl Pts',(-3.53015556945347,-2.23943063412497,
4.3));
#21232=CARTESIAN_POINT('Ctrl Pts',(-3.53949489532435,-2.23701751505981,
4.3));
#21233=CARTESIAN_POINT('Ctrl Pts',(-3.54298225084135,-2.23611644316218,
4.3));
#21234=CARTESIAN_POINT('Ctrl Pts',(-3.54649061678302,-2.23532167500438,
4.3));
#21235=CARTESIAN_POINT('Ctrl Pts',(-3.5500119948057,-2.23463615769257,4.3));
#21236=CARTESIAN_POINT('Ctrl Pts',(-3.5610932074021,-2.23247894451586,4.3));
#21237=CARTESIAN_POINT('Ctrl Pts',(-3.57231428638466,-2.23139729676061,
4.3));
#21238=CARTESIAN_POINT('Ctrl Pts',(-3.58352462409827,-2.2314877485142,4.3));
#21239=CARTESIAN_POINT('Ctrl Pts',(-3.58970653876345,-2.23153762792339,
4.3));
#21240=CARTESIAN_POINT('Ctrl Pts',(-3.59588508216706,-2.23194477463139,
4.3));
#21241=CARTESIAN_POINT('Ctrl Pts',(-3.60203269161667,-2.23273189903069,
4.3));
#21242=CARTESIAN_POINT('Ctrl Pts',(-3.60310835631345,-2.23286962442383,
4.3));
#21243=CARTESIAN_POINT('Ctrl Pts',(-3.60418306761235,-2.23301899515145,
4.3));
#21244=CARTESIAN_POINT('Ctrl Pts',(-3.60525667255607,-2.23317994016621,
4.3));
#21245=CARTESIAN_POINT('Origin',(-3.6,-2.4,5.35459252805377));
#21246=CARTESIAN_POINT('Ctrl Pts',(-3.80565733457988,-2.39985006589818,
5.17959252805377));
#21247=CARTESIAN_POINT('Ctrl Pts',(-3.8057391516022,-2.39002097154438,5.17905813053169));
#21248=CARTESIAN_POINT('Ctrl Pts',(-3.80062938506941,-2.31213685567809,
5.17481913665734));
#21249=CARTESIAN_POINT('Ctrl Pts',(-3.70109554203788,-2.17915701647198,
5.16687554643073));
#21250=CARTESIAN_POINT('Ctrl Pts',(-3.46929950206046,-2.19531102353728,
5.15576175737392));
#21251=CARTESIAN_POINT('Ctrl Pts',(-3.35713783153282,-2.39878694399818,
5.14464796831711));
#21252=CARTESIAN_POINT('Ctrl Pts',(-3.46726929886284,-2.60338928299931,
5.13353417926032));
#21253=CARTESIAN_POINT('Ctrl Pts',(-3.69889136100131,-2.62181906697108,
5.12242039020351));
#21254=CARTESIAN_POINT('Ctrl Pts',(-3.80021578451737,-2.48926235936684,
5.11443983980133));
#21255=CARTESIAN_POINT('Ctrl Pts',(-3.80572902589707,-2.41067410853188,
5.11016388575141));
#21256=CARTESIAN_POINT('Ctrl Pts',(-3.8056388038084,-2.40016037433918,5.10959252805377));
#21257=CARTESIAN_POINT('Ctrl Pts',(-3.80526708169851,-2.40022955265959,
5.18540747194623));
#21258=CARTESIAN_POINT('Ctrl Pts',(-3.80491230300414,-2.3532097525552,5.18286245525962));
#21259=CARTESIAN_POINT('Ctrl Pts',(-3.76565541968849,-2.23704708335906,
5.17661284222073));
#21260=CARTESIAN_POINT('Ctrl Pts',(-3.5727867642971,-2.15871465280967,5.16665863282959));
#21261=CARTESIAN_POINT('Ctrl Pts',(-3.38252461999799,-2.29190667528476,
5.15554484377278));
#21262=CARTESIAN_POINT('Ctrl Pts',(-3.39123766053156,-2.52413789941101,
5.14443105471598));
#21263=CARTESIAN_POINT('Ctrl Pts',(-3.59107442597796,-2.64269432067786,
5.13331726565918));
#21264=CARTESIAN_POINT('Ctrl Pts',(-3.77212564872883,-2.55254602634109,
5.12364273806926));
#21265=CARTESIAN_POINT('Ctrl Pts',(-3.80499226553068,-2.44179202539712,
5.11767280683161));
#21266=CARTESIAN_POINT('Ctrl Pts',(-3.80520912268496,-2.39988380060309,
5.11540747194623));
#21267=CARTESIAN_POINT('Ctrl Pts',(-3.47309291201476,-2.29206413469515,
5.2));
#21268=CARTESIAN_POINT('Ctrl Pts',(-3.43720166889934,-2.33426376069605,
5.19629540364773));
#21269=CARTESIAN_POINT('Ctrl Pts',(-3.4114791580674,-2.45658678033172,5.1888862109432));
#21270=CARTESIAN_POINT('Ctrl Pts',(-3.54548746492724,-2.5893415011903,5.17777242188639));
#21271=CARTESIAN_POINT('Ctrl Pts',(-3.72942274690437,-2.54835673318009,
5.16665863282959));
#21272=CARTESIAN_POINT('Ctrl Pts',(-3.79487861290014,-2.37179020383286,
5.15554484377278));
#21273=CARTESIAN_POINT('Ctrl Pts',(-3.68196869353212,-2.22093957388603,
5.14443105471598));
#21274=CARTESIAN_POINT('Ctrl Pts',(-3.49402748287272,-2.23403731121212,
5.13331726565918));
#21275=CARTESIAN_POINT('Ctrl Pts',(-3.40308632550611,-2.39901644905753,
5.12220347660237));
#21276=CARTESIAN_POINT('Ctrl Pts',(-3.49238138552402,-2.56490889182472,
5.11108968754557));
#21277=CARTESIAN_POINT('Ctrl Pts',(-3.68018153421496,-2.57985183870243,
5.09997589848876));
#21278=CARTESIAN_POINT('Ctrl Pts',(-3.79459034046341,-2.43017761257843,
5.08886210943196));
#21279=CARTESIAN_POINT('Ctrl Pts',(-3.73088853854501,-2.25287985005212,
5.07774832037516));
#21280=CARTESIAN_POINT('Ctrl Pts',(-3.5473829043692,-2.21024364094684,5.06663453131835));
#21281=CARTESIAN_POINT('Ctrl Pts',(-3.41203832877697,-2.34129317389102,
5.05552074226154));
#21282=CARTESIAN_POINT('Ctrl Pts',(-3.44873718538878,-2.52607793299967,
5.04440695320475));
#21283=CARTESIAN_POINT('Ctrl Pts',(-3.62388862018941,-2.59546202911018,
5.03329316414794));
#21284=CARTESIAN_POINT('Ctrl Pts',(-3.77717452575129,-2.48593756377701,
5.02217937509113));
#21285=CARTESIAN_POINT('Ctrl Pts',(-3.76829058072669,-2.29775344650504,
5.01106558603433));
#21286=CARTESIAN_POINT('Ctrl Pts',(-3.6053683575545,-2.20315677179449,4.99995179697753));
#21287=CARTESIAN_POINT('Ctrl Pts',(-3.43753241636245,-2.28873292992563,
4.98883800792072));
#21288=CARTESIAN_POINT('Ctrl Pts',(-3.41840489671633,-2.47615310229093,
4.97772421886392));
#21289=CARTESIAN_POINT('Ctrl Pts',(-3.56549343466676,-2.59386947492594,
4.96661042980711));
#21290=CARTESIAN_POINT('Ctrl Pts',(-3.74416622313161,-2.53413491931517,
4.95549664075031));
#21291=CARTESIAN_POINT('Ctrl Pts',(-3.79088203264097,-2.35162515047058,
4.9443828516935));
#21292=CARTESIAN_POINT('Ctrl Pts',(-3.66288135290806,-2.21339343020375,
4.9332690626367));
#21293=CARTESIAN_POINT('Ctrl Pts',(-3.47732465774361,-2.24596481943629,
4.9221552735799));
#21294=CARTESIAN_POINT('Ctrl Pts',(-3.40405409457531,-2.41952635636528,
4.91104148452309));
#21295=CARTESIAN_POINT('Ctrl Pts',(-3.51013504082201,-2.57521519784486,
4.89992769546629));
#21296=CARTESIAN_POINT('Ctrl Pts',(-3.69847040334124,-2.57052758167369,
4.88881390640948));
#21297=CARTESIAN_POINT('Ctrl Pts',(-3.79667468895243,-2.40975413607622,
4.87770011735268));
#21298=CARTESIAN_POINT('Ctrl Pts',(-3.71486040132253,-2.24005261911178,
4.86658632829587));
#21299=CARTESIAN_POINT('Ctrl Pts',(-3.5279130857567,-2.2167527537995,4.85547253923907));
#21300=CARTESIAN_POINT('Ctrl Pts',(-3.40694774031892,-2.3611811711004,4.84435875018227));
#21301=CARTESIAN_POINT('Ctrl Pts',(-3.46268531752878,-2.5411409027282,4.83324496112546));
#21302=CARTESIAN_POINT('Ctrl Pts',(-3.64410858085897,-2.59191276544236,
4.82213117206866));
#21303=CARTESIAN_POINT('Ctrl Pts',(-3.7851587599036,-2.46702469750825,4.81101738301185));
#21304=CARTESIAN_POINT('Ctrl Pts',(-3.75673102616532,-2.28078816383312,
4.79990359395505));
#21305=CARTESIAN_POINT('Ctrl Pts',(-3.58484560672719,-2.20366757575568,
4.78878980489824));
#21306=CARTESIAN_POINT('Ctrl Pts',(-3.42683117531417,-2.30625228215021,
4.77767601584145));
#21307=CARTESIAN_POINT('Ctrl Pts',(-3.42732013300413,-2.49464533786407,
4.76656222678464));
#21308=CARTESIAN_POINT('Ctrl Pts',(-3.5858649312783,-2.59640844247982,4.75544843772783));
#21309=CARTESIAN_POINT('Ctrl Pts',(-3.75734771825602,-2.51839667227055,
4.74433464867103));
#21310=CARTESIAN_POINT('Ctrl Pts',(-3.78480835426951,-2.33201508522246,
4.73322085961423));
#21311=CARTESIAN_POINT('Ctrl Pts',(-3.64311180775084,-2.20786086167162,
4.72210707055742));
#21312=CARTESIAN_POINT('Ctrl Pts',(-3.46195453467666,-2.25957377043879,
4.71099328150062));
#21313=CARTESIAN_POINT('Ctrl Pts',(-3.407151841555,-2.43982039966509,4.69987949244381));
#21314=CARTESIAN_POINT('Ctrl Pts',(-3.52886525490491,-2.58361896548389,
4.68876570338701));
#21315=CARTESIAN_POINT('Ctrl Pts',(-3.71568910716324,-2.55934900981458,
4.6776519143302));
#21316=CARTESIAN_POINT('Ctrl Pts',(-3.79662140763134,-2.38922509832133,
4.6665381252734));
#21317=CARTESIAN_POINT('Ctrl Pts',(-3.69758390385606,-2.22896357653021,
4.65542433621659));
#21318=CARTESIAN_POINT('Ctrl Pts',(-3.50922674620458,-2.22525363282606,
4.64431054715979));
#21319=CARTESIAN_POINT('Ctrl Pts',(-3.40395537719079,-2.38149102075462,
4.63319675810299));
#21320=CARTESIAN_POINT('Ctrl Pts',(-3.47812587473144,-2.55466988729295,
4.62208296904618));
#21321=CARTESIAN_POINT('Ctrl Pts',(-3.66384914127714,-2.58627765191548,
4.61096917998938));
#21322=CARTESIAN_POINT('Ctrl Pts',(-3.79113056471305,-2.447383369209,4.59985539093257));
#21323=CARTESIAN_POINT('Ctrl Pts',(-3.74346801469971,-2.26511855129859,
4.58874160187577));
#21324=CARTESIAN_POINT('Ctrl Pts',(-3.56448756379251,-2.20631225305021,
4.57762781281896));
#21325=CARTESIAN_POINT('Ctrl Pts',(-3.41801204848697,-2.32479054614148,
4.56651402376216));
#21326=CARTESIAN_POINT('Ctrl Pts',(-3.43811216908,-2.51210890530657,4.55540023470536));
#21327=CARTESIAN_POINT('Ctrl Pts',(-3.60639005725709,-2.59681271199525,
4.54428644564855));
#21328=CARTESIAN_POINT('Ctrl Pts',(-3.76881905353834,-2.50137161148251,
4.53317265659175));
#21329=CARTESIAN_POINT('Ctrl Pts',(-3.77672605561821,-2.31314392515575,
4.52205886753495));
#21330=CARTESIAN_POINT('Ctrl Pts',(-3.62287369469976,-2.2044165895329,4.51094507847814));
#21331=CARTESIAN_POINT('Ctrl Pts',(-3.44808478177985,-2.27470896680823,
4.49983128942134));
#21332=CARTESIAN_POINT('Ctrl Pts',(-3.41234559060706,-2.45968164920097,
4.48871750036453));
#21333=CARTESIAN_POINT('Ctrl Pts',(-3.54836860914922,-2.5900270381604,4.47760371130773));
#21334=CARTESIAN_POINT('Ctrl Pts',(-3.73165042397165,-2.54643853021323,
4.46648992225092));
#21335=CARTESIAN_POINT('Ctrl Pts',(-3.79443111532907,-2.36881316247168,
4.45537613319412));
#21336=CARTESIAN_POINT('Ctrl Pts',(-3.67924679659355,-2.21973348556073,
4.44426234413731));
#21337=CARTESIAN_POINT('Ctrl Pts',(-3.49152699669547,-2.23565374410205,
4.43314855508051));
#21338=CARTESIAN_POINT('Ctrl Pts',(-3.40309374590592,-2.40200209374894,
4.4220347660237));
#21339=CARTESIAN_POINT('Ctrl Pts',(-3.49489106457482,-2.5665177055076,4.41092097696691));
#21340=CARTESIAN_POINT('Ctrl Pts',(-3.68289569971986,-2.57861817099917,
4.39980718791009));
#21341=CARTESIAN_POINT('Ctrl Pts',(-3.79502512928071,-2.42722660191142,
4.3886933988533));
#21342=CARTESIAN_POINT('Ctrl Pts',(-3.72864550893249,-2.25091581121659,
4.37757960979648));
#21343=CARTESIAN_POINT('Ctrl Pts',(-3.54451587080997,-2.21106027365159,
4.36646582073969));
#21344=CARTESIAN_POINT('Ctrl Pts',(-3.41117013277341,-2.34414980914689,
4.35535203168287));
#21345=CARTESIAN_POINT('Ctrl Pts',(-3.45066522211898,-2.5283468448043,4.34423824262609));
#21346=CARTESIAN_POINT('Ctrl Pts',(-3.62684270366593,-2.59509221455348,
4.33312445356927));
#21347=CARTESIAN_POINT('Ctrl Pts',(-3.77846161739066,-2.4832160890933,4.32201066451248));
#21348=CARTESIAN_POINT('Ctrl Pts',(-3.76671079422265,-2.29527426875025,
4.31089687545566));
#21349=CARTESIAN_POINT('Ctrl Pts',(-3.60241192612029,-2.2029822262702,4.29978308639886));
#21350=CARTESIAN_POINT('Ctrl Pts',(-3.43581020892599,-2.29144640006724,
4.28866929734205));
#21351=CARTESIAN_POINT('Ctrl Pts',(-3.42516046182893,-2.41599017382995,
4.28126010463752));
#21352=CARTESIAN_POINT('Ctrl Pts',(-3.44735576439472,-2.46674801372685,
4.27755550828525));
#21353=CARTESIAN_POINT('Ctrl Pts',(-3.46322193753412,-2.28366876301903,
5.20748149723825));
#21354=CARTESIAN_POINT('Ctrl Pts',(-3.42453903360214,-2.32915072287504,
5.20377690088598));
#21355=CARTESIAN_POINT('Ctrl Pts',(-3.39681579726281,-2.4609881630556,5.19636770818145));
#21356=CARTESIAN_POINT('Ctrl Pts',(-3.54124741930709,-2.60406869378488,
5.18525391912464));
#21357=CARTESIAN_POINT('Ctrl Pts',(-3.73948939213428,-2.55989608492554,
5.17414013006784));
#21358=CARTESIAN_POINT('Ctrl Pts',(-3.81003648820324,-2.36959601450513,
5.16302634101103));
#21359=CARTESIAN_POINT('Ctrl Pts',(-3.68834430970071,-2.20701205474802,
5.15191255195423));
#21360=CARTESIAN_POINT('Ctrl Pts',(-3.48578482260197,-2.22112854865384,
5.14079876289742));
#21361=CARTESIAN_POINT('Ctrl Pts',(-3.38777016084835,-2.39893994737108,
5.12968497384062));
#21362=CARTESIAN_POINT('Ctrl Pts',(-3.4840106899703,-2.57773568888292,5.11857118478382));
#21363=CARTESIAN_POINT('Ctrl Pts',(-3.68641814314374,-2.59384091479198,
5.10745739572701));
#21364=CARTESIAN_POINT('Ctrl Pts',(-3.8097257936157,-2.43252486085572,5.0963436066702));
#21365=CARTESIAN_POINT('Ctrl Pts',(-3.74106919467933,-2.2414366811261,5.08522981761341));
#21366=CARTESIAN_POINT('Ctrl Pts',(-3.54329028813742,-2.19548418024617,
5.0741160285566));
#21367=CARTESIAN_POINT('Ctrl Pts',(-3.39741846089223,-2.33672689164815,
5.06300223949979));
#21368=CARTESIAN_POINT('Ctrl Pts',(-3.43697179539676,-2.53588441488314,
5.051888450443));
#21369=CARTESIAN_POINT('Ctrl Pts',(-3.62574670364252,-2.61066528317513,
5.04077466138618));
#21370=CARTESIAN_POINT('Ctrl Pts',(-3.79095535746114,-2.4926218830884,5.02966087232938));
#21371=CARTESIAN_POINT('Ctrl Pts',(-3.78138040930963,-2.28980059583054,
5.01854708327258));
#21372=CARTESIAN_POINT('Ctrl Pts',(-3.60578591437709,-2.1878460865274,5.00743329421578));
#21373=CARTESIAN_POINT('Ctrl Pts',(-3.42489550697087,-2.28007845343676,
4.99631950515897));
#21374=CARTESIAN_POINT('Ctrl Pts',(-3.40428022756837,-2.48207637530325,
4.98520571610216));
#21375=CARTESIAN_POINT('Ctrl Pts',(-3.56280947562848,-2.60894885835481,
4.97409192704536));
#21376=CARTESIAN_POINT('Ctrl Pts',(-3.75537963234378,-2.54456808255722,
4.96297813798856));
#21377=CARTESIAN_POINT('Ctrl Pts',(-3.80572904948554,-2.34786250085983,
4.95186434893175));
#21378=CARTESIAN_POINT('Ctrl Pts',(-3.6677723344893,-2.19887896361545,4.94075055987495));
#21379=CARTESIAN_POINT('Ctrl Pts',(-3.46778283315333,-2.23398379173638,
4.92963677081814));
#21380=CARTESIAN_POINT('Ctrl Pts',(-3.38881320407234,-2.42104513808537,
4.91852298176134));
#21381=CARTESIAN_POINT('Ctrl Pts',(-3.50314524432732,-2.5888436308505,4.90740919270454));
#21382=CARTESIAN_POINT('Ctrl Pts',(-3.70612954085602,-2.58379140667882,
4.89629540364773));
#21383=CARTESIAN_POINT('Ctrl Pts',(-3.81197226504892,-2.41051282363117,
4.88518161459093));
#21384=CARTESIAN_POINT('Ctrl Pts',(-3.72379437111327,-2.22761173389364,
4.87406782553412));
#21385=CARTESIAN_POINT('Ctrl Pts',(-3.52230608537413,-2.20249957913754,
4.86295403647732));
#21386=CARTESIAN_POINT('Ctrl Pts',(-3.3919319208009,-2.35816179940478,4.85184024742052));
#21387=CARTESIAN_POINT('Ctrl Pts',(-3.45200482877115,-2.55211899915388,
4.84072645836371));
#21388=CARTESIAN_POINT('Ctrl Pts',(-3.64753939534654,-2.60683995383086,
4.82961266930691));
#21389=CARTESIAN_POINT('Ctrl Pts',(-3.79956061422784,-2.47223795304173,
4.8184988802501));
#21390=CARTESIAN_POINT('Ctrl Pts',(-3.7689217397351,-2.27151573459945,4.8073850911933));
#21391=CARTESIAN_POINT('Ctrl Pts',(-3.58366688116,-2.18839662138894,4.79627130213649));
#21392=CARTESIAN_POINT('Ctrl Pts',(-3.41336191148932,-2.29896048036668,
4.78515751307969));
#21393=CARTESIAN_POINT('Ctrl Pts',(-3.41388890085234,-2.50200695753087,
4.77404372402289));
#21394=CARTESIAN_POINT('Ctrl Pts',(-3.58476548990864,-2.61168530962949,
4.76292993496608));
#21395=CARTESIAN_POINT('Ctrl Pts',(-3.76958639882265,-2.52760569714953,
4.75181614590928));
#21396=CARTESIAN_POINT('Ctrl Pts',(-3.79918295365372,-2.32672714292159,
4.74070235685248));
#21397=CARTESIAN_POINT('Ctrl Pts',(-3.64646509211721,-2.19291606574822,
4.72958856779567));
#21398=CARTESIAN_POINT('Ctrl Pts',(-3.45121720481583,-2.24865126208706,
4.71847477873887));
#21399=CARTESIAN_POINT('Ctrl Pts',(-3.39215189725818,-2.44291767464904,
4.70736098968205));
#21400=CARTESIAN_POINT('Ctrl Pts',(-3.52333231529793,-2.59790105288522,
4.69624720062526));
#21401=CARTESIAN_POINT('Ctrl Pts',(-3.72468753461616,-2.57174335306496,
4.68513341156845));
#21402=CARTESIAN_POINT('Ctrl Pts',(-3.8119148394474,-2.38838701448227,4.67401962251165));
#21403=CARTESIAN_POINT('Ctrl Pts',(-3.70517408845471,-2.21566017324412,
4.66290583345485));
#21404=CARTESIAN_POINT('Ctrl Pts',(-3.50216630154411,-2.21166166599155,
4.65179204439804));
#21405=CARTESIAN_POINT('Ctrl Pts',(-3.38870680833984,-2.38005137175869,
4.64067825534123));
#21406=CARTESIAN_POINT('Ctrl Pts',(-3.46864636968979,-2.56670028318833,
4.62956446628443));
#21407=CARTESIAN_POINT('Ctrl Pts',(-3.66881539851434,-2.6007665349051,4.61845067722763));
#21408=CARTESIAN_POINT('Ctrl Pts',(-3.80599691265867,-2.45106890037747,
4.60733688817082));
#21409=CARTESIAN_POINT('Ctrl Pts',(-3.75462711648332,-2.25462732217041,
4.59622309911401));
#21410=CARTESIAN_POINT('Ctrl Pts',(-3.56172536699866,-2.1912470046255,4.58510931005722));
#21411=CARTESIAN_POINT('Ctrl Pts',(-3.4038568231667,-2.31894067115399,4.57399552100041));
#21412=CARTESIAN_POINT('Ctrl Pts',(-3.42552035349974,-2.5208288606763,4.56288173194361));
#21413=CARTESIAN_POINT('Ctrl Pts',(-3.60688708301913,-2.61212102367755,
4.5517679428868));
#21414=CARTESIAN_POINT('Ctrl Pts',(-3.78194998732446,-2.50925640819396,
4.54065415383));
#21415=CARTESIAN_POINT('Ctrl Pts',(-3.79047200482221,-2.30638816303176,
4.52954036477319));
#21416=CARTESIAN_POINT('Ctrl Pts',(-3.62465283611923,-2.18920389429099,
4.51842657571639));
#21417=CARTESIAN_POINT('Ctrl Pts',(-3.43626864710937,-2.2649636908672,4.50731278665958));
#21418=CARTESIAN_POINT('Ctrl Pts',(-3.39774962188927,-2.46432375426836,
4.49619899760278));
#21419=CARTESIAN_POINT('Ctrl Pts',(-3.54435266213177,-2.60480755258314,
4.48508520854598));
#21420=CARTESIAN_POINT('Ctrl Pts',(-3.74189034040202,-2.55782868199802,
4.47397141948917));
#21421=CARTESIAN_POINT('Ctrl Pts',(-3.80955418377328,-2.36638741555509,
4.46285763043236));
#21422=CARTESIAN_POINT('Ctrl Pts',(-3.68541070059029,-2.20571215553106,
4.45174384137557));
#21423=CARTESIAN_POINT('Ctrl Pts',(-3.4830898458282,-2.22287070949214,4.44063005231875));
#21424=CARTESIAN_POINT('Ctrl Pts',(-3.3877781584151,-2.40215781882795,4.42951626326196));
#21425=CARTESIAN_POINT('Ctrl Pts',(-3.48671557464955,-2.57946963788377,
4.41840247420515));
#21426=CARTESIAN_POINT('Ctrl Pts',(-3.68934341946097,-2.59251129104238,
4.40728868514835));
#21427=CARTESIAN_POINT('Ctrl Pts',(-3.81019440079089,-2.42934431729619,
4.39617489609154));
#21428=CARTESIAN_POINT('Ctrl Pts',(-3.73865169972831,-2.23931987716506,
4.38506110703474));
#21429=CARTESIAN_POINT('Ctrl Pts',(-3.54020025351852,-2.19636433155117,
4.37394731797794));
#21430=CARTESIAN_POINT('Ctrl Pts',(-3.39648273563768,-2.33980571917207,
4.36283352892113));
#21431=CARTESIAN_POINT('Ctrl Pts',(-3.43904979696867,-2.53832980517198,
4.35171973986433));
#21432=CARTESIAN_POINT('Ctrl Pts',(-3.6289305590181,-2.6102667040308,4.34060595080752));
#21433=CARTESIAN_POINT('Ctrl Pts',(-3.79234256052004,-2.48968872907629,
4.32949216175072));
#21434=CARTESIAN_POINT('Ctrl Pts',(-3.77967774525388,-2.28712858487203,
4.31837837269391));
#21435=CARTESIAN_POINT('Ctrl Pts',(-3.60259952841706,-2.18765796465806,
4.30726458363711));
#21436=CARTESIAN_POINT('Ctrl Pts',(-3.42303934432415,-2.28300298030457,
4.29615079458031));
#21437=CARTESIAN_POINT('Ctrl Pts',(-3.41156124805061,-2.41723390733863,
4.28874160187577));
#21438=CARTESIAN_POINT('Ctrl Pts',(-3.43548292594103,-2.47193974848801,
4.2850370055235));
#21439=CARTESIAN_POINT('Ctrl Pts',(-3.45335096305347,-2.2752733913429,5.2149629944765));
#21440=CARTESIAN_POINT('Ctrl Pts',(-3.41187639830495,-2.32403768505403,
5.21125839812423));
#21441=CARTESIAN_POINT('Ctrl Pts',(-3.38215243645823,-2.46538954577948,
5.20384920541969));
#21442=CARTESIAN_POINT('Ctrl Pts',(-3.53700737368693,-2.61879588637947,
5.19273541636289));
#21443=CARTESIAN_POINT('Ctrl Pts',(-3.74955603736419,-2.571435436671,5.18162162730609));
#21444=CARTESIAN_POINT('Ctrl Pts',(-3.82519436350635,-2.3674018251774,5.17050783824928));
#21445=CARTESIAN_POINT('Ctrl Pts',(-3.69471992586929,-2.19308453561,5.15939404919247));
#21446=CARTESIAN_POINT('Ctrl Pts',(-3.47754216233122,-2.20821978609556,
5.14828026013568));
#21447=CARTESIAN_POINT('Ctrl Pts',(-3.37245399619058,-2.39886344568463,
5.13716647107886));
#21448=CARTESIAN_POINT('Ctrl Pts',(-3.47563999441657,-2.59056248594111,
5.12605268202207));
#21449=CARTESIAN_POINT('Ctrl Pts',(-3.69265475207253,-2.60782999088153,
5.11493889296526));
#21450=CARTESIAN_POINT('Ctrl Pts',(-3.82486124676799,-2.434872109133,5.10382510390846));
#21451=CARTESIAN_POINT('Ctrl Pts',(-3.75124985081366,-2.22999351220008,
5.09271131485165));
#21452=CARTESIAN_POINT('Ctrl Pts',(-3.53919767190563,-2.18072471954551,
5.08159752579485));
#21453=CARTESIAN_POINT('Ctrl Pts',(-3.38279859300748,-2.33216060940528,
5.07048373673804));
#21454=CARTESIAN_POINT('Ctrl Pts',(-3.42520640540474,-2.54569089676662,
5.05936994768124));
#21455=CARTESIAN_POINT('Ctrl Pts',(-3.62760478709563,-2.62586853724007,
5.04825615862444));
#21456=CARTESIAN_POINT('Ctrl Pts',(-3.80473618917098,-2.49930620239979,
5.03714236956763));
#21457=CARTESIAN_POINT('Ctrl Pts',(-3.79447023789256,-2.28184774515603,
5.02602858051083));
#21458=CARTESIAN_POINT('Ctrl Pts',(-3.60620347119968,-2.17253540126032,
5.01491479145402));
#21459=CARTESIAN_POINT('Ctrl Pts',(-3.4122585975793,-2.27142397694788,5.00380100239722));
#21460=CARTESIAN_POINT('Ctrl Pts',(-3.39015555842041,-2.48799964831557,
4.99268721334041));
#21461=CARTESIAN_POINT('Ctrl Pts',(-3.56012551659021,-2.62402824178367,
4.98157342428361));
#21462=CARTESIAN_POINT('Ctrl Pts',(-3.76659304155595,-2.55500124579927,
4.97045963522681));
#21463=CARTESIAN_POINT('Ctrl Pts',(-3.82057606633011,-2.34409985124907,
4.95934584617));
#21464=CARTESIAN_POINT('Ctrl Pts',(-3.67266331607053,-2.18436449702716,
4.9482320571132));
#21465=CARTESIAN_POINT('Ctrl Pts',(-3.45824100856306,-2.22200276403647,
4.93711826805639));
#21466=CARTESIAN_POINT('Ctrl Pts',(-3.37357231356937,-2.42256391980546,
4.92600447899959));
#21467=CARTESIAN_POINT('Ctrl Pts',(-3.49615544783263,-2.60247206385614,
4.91489068994279));
#21468=CARTESIAN_POINT('Ctrl Pts',(-3.71378867837081,-2.59705523168396,
4.90377690088598));
#21469=CARTESIAN_POINT('Ctrl Pts',(-3.82726984114541,-2.41127151118611,
4.89266311182918));
#21470=CARTESIAN_POINT('Ctrl Pts',(-3.73272834090401,-2.21517084867549,
4.88154932277237));
#21471=CARTESIAN_POINT('Ctrl Pts',(-3.51669908499156,-2.18824640447558,
4.87043553371557));
#21472=CARTESIAN_POINT('Ctrl Pts',(-3.37691610128289,-2.35514242770916,
4.85932174465877));
#21473=CARTESIAN_POINT('Ctrl Pts',(-3.44132434001351,-2.56309709557957,
4.84820795560196));
#21474=CARTESIAN_POINT('Ctrl Pts',(-3.65097020983412,-2.62176714221935,
4.83709416654516));
#21475=CARTESIAN_POINT('Ctrl Pts',(-3.81396246855208,-2.47745120857521,
4.82598037748835));
#21476=CARTESIAN_POINT('Ctrl Pts',(-3.78111245330488,-2.26224330536578,
4.81486658843155));
#21477=CARTESIAN_POINT('Ctrl Pts',(-3.58248815559281,-2.1731256670222,4.80375279937474));
#21478=CARTESIAN_POINT('Ctrl Pts',(-3.39989264766446,-2.29166867858314,
4.79263901031794));
#21479=CARTESIAN_POINT('Ctrl Pts',(-3.40045766870055,-2.50936857719767,
4.78152522126113));
#21480=CARTESIAN_POINT('Ctrl Pts',(-3.58366604853898,-2.62696217677915,
4.77041143220433));
#21481=CARTESIAN_POINT('Ctrl Pts',(-3.78182507938928,-2.53681472202852,
4.75929764314753));
#21482=CARTESIAN_POINT('Ctrl Pts',(-3.81355755303793,-2.32143920062071,
4.74818385409072));
#21483=CARTESIAN_POINT('Ctrl Pts',(-3.64981837648358,-2.17797126982482,
4.73707006503392));
#21484=CARTESIAN_POINT('Ctrl Pts',(-3.440479874955,-2.23772875373533,4.72595627597712));
#21485=CARTESIAN_POINT('Ctrl Pts',(-3.37715195296136,-2.44601494963299,
4.71484248692031));
#21486=CARTESIAN_POINT('Ctrl Pts',(-3.51779937569094,-2.61218314028655,
4.7037286978635));
#21487=CARTESIAN_POINT('Ctrl Pts',(-3.73368596206909,-2.58413769631535,
4.69261490880671));
#21488=CARTESIAN_POINT('Ctrl Pts',(-3.82720827126346,-2.38754893064322,
4.68150111974989));
#21489=CARTESIAN_POINT('Ctrl Pts',(-3.71276427305336,-2.20235676995803,
4.6703873306931));
#21490=CARTESIAN_POINT('Ctrl Pts',(-3.49510585688365,-2.19806969915704,
4.65927354163628));
#21491=CARTESIAN_POINT('Ctrl Pts',(-3.37345823948888,-2.37861172276277,
4.64815975257949));
#21492=CARTESIAN_POINT('Ctrl Pts',(-3.45916686464814,-2.57873067908372,
4.63704596352267));
#21493=CARTESIAN_POINT('Ctrl Pts',(-3.67378165575153,-2.61525541789472,
4.62593217446588));
#21494=CARTESIAN_POINT('Ctrl Pts',(-3.82086326060429,-2.45475443154594,
4.61481838540906));
#21495=CARTESIAN_POINT('Ctrl Pts',(-3.76578621826694,-2.24413609304223,
4.60370459635227));
#21496=CARTESIAN_POINT('Ctrl Pts',(-3.55896317020481,-2.17618175620078,
4.59259080729546));
#21497=CARTESIAN_POINT('Ctrl Pts',(-3.38970159784644,-2.3130907961665,4.58147701823866));
#21498=CARTESIAN_POINT('Ctrl Pts',(-3.41292853791948,-2.52954881604603,
4.57036322918185));
#21499=CARTESIAN_POINT('Ctrl Pts',(-3.60738410878117,-2.62742933535986,
4.55924944012506));
#21500=CARTESIAN_POINT('Ctrl Pts',(-3.79508092111058,-2.51714120490541,
4.54813565106824));
#21501=CARTESIAN_POINT('Ctrl Pts',(-3.8042179540262,-2.29963240090777,4.53702186201145));
#21502=CARTESIAN_POINT('Ctrl Pts',(-3.62643197753871,-2.17399119904908,
4.52590807295463));
#21503=CARTESIAN_POINT('Ctrl Pts',(-3.42445251243888,-2.25521841492616,
4.51479428389784));
#21504=CARTESIAN_POINT('Ctrl Pts',(-3.38315365317149,-2.46896585933577,
4.50368049484102));
#21505=CARTESIAN_POINT('Ctrl Pts',(-3.54033671511431,-2.61958806700588,
4.49256670578423));
#21506=CARTESIAN_POINT('Ctrl Pts',(-3.75213025683239,-2.56921883378282,
4.48145291672742));
#21507=CARTESIAN_POINT('Ctrl Pts',(-3.82467725221749,-2.3639616686385,4.47033912767062));
#21508=CARTESIAN_POINT('Ctrl Pts',(-3.69157460458704,-2.1916908255014,4.45922533861381));
#21509=CARTESIAN_POINT('Ctrl Pts',(-3.47465269496093,-2.21008767488223,
4.44811154955701));
#21510=CARTESIAN_POINT('Ctrl Pts',(-3.37246257092429,-2.40231354390696,
4.4369977605002));
#21511=CARTESIAN_POINT('Ctrl Pts',(-3.47854008472427,-2.59242157025994,
4.4258839714434));
#21512=CARTESIAN_POINT('Ctrl Pts',(-3.69579113920209,-2.60640441108558,
4.41477018238659));
#21513=CARTESIAN_POINT('Ctrl Pts',(-3.82536367230107,-2.43146203268096,
4.4036563933298));
#21514=CARTESIAN_POINT('Ctrl Pts',(-3.74865789052413,-2.22772394311352,
4.39254260427298));
#21515=CARTESIAN_POINT('Ctrl Pts',(-3.53588463622708,-2.18166838945074,
4.38142881521619));
#21516=CARTESIAN_POINT('Ctrl Pts',(-3.38179533850196,-2.33546162919725,
4.37031502615938));
#21517=CARTESIAN_POINT('Ctrl Pts',(-3.42743437181836,-2.54831276553967,
4.35920123710258));
#21518=CARTESIAN_POINT('Ctrl Pts',(-3.63101841437027,-2.62544119350812,
4.34808744804577));
#21519=CARTESIAN_POINT('Ctrl Pts',(-3.80622350364941,-2.49616136905929,
4.33697365898897));
#21520=CARTESIAN_POINT('Ctrl Pts',(-3.7926446962851,-2.27898290099381,4.32585986993216));
#21521=CARTESIAN_POINT('Ctrl Pts',(-3.60278713071383,-2.17233370304593,
4.31474608087535));
#21522=CARTESIAN_POINT('Ctrl Pts',(-3.4102684797223,-2.27455956054189,4.30363229181856));
#21523=CARTESIAN_POINT('Ctrl Pts',(-3.3979620342723,-2.41847764084731,4.29622309911402));
#21524=CARTESIAN_POINT('Ctrl Pts',(-3.42361008748733,-2.47713148324918,
4.29251850276175));
#21525=CARTESIAN_POINT('Ctrl Pts',(-3.44347998857283,-2.26687801966678,
5.22244449171475));
#21526=CARTESIAN_POINT('Ctrl Pts',(-3.39921376300775,-2.31892464723302,
5.21873989536248));
#21527=CARTESIAN_POINT('Ctrl Pts',(-3.36748907565365,-2.46979092850336,
5.21133070265795));
#21528=CARTESIAN_POINT('Ctrl Pts',(-3.53276732806678,-2.63352307897406,
5.20021691360113));
#21529=CARTESIAN_POINT('Ctrl Pts',(-3.75962268259409,-2.58297478841644,
5.18910312454434));
#21530=CARTESIAN_POINT('Ctrl Pts',(-3.84035223880946,-2.36520763584968,
5.17798933548753));
#21531=CARTESIAN_POINT('Ctrl Pts',(-3.70109554203788,-2.17915701647198,
5.16687554643073));
#21532=CARTESIAN_POINT('Ctrl Pts',(-3.46929950206046,-2.19531102353728,
5.15576175737392));
#21533=CARTESIAN_POINT('Ctrl Pts',(-3.35713783153282,-2.39878694399818,
5.14464796831711));
#21534=CARTESIAN_POINT('Ctrl Pts',(-3.46726929886284,-2.60338928299931,
5.13353417926032));
#21535=CARTESIAN_POINT('Ctrl Pts',(-3.69889136100131,-2.62181906697108,
5.12242039020351));
#21536=CARTESIAN_POINT('Ctrl Pts',(-3.83999669992028,-2.43721935741029,
5.1113066011467));
#21537=CARTESIAN_POINT('Ctrl Pts',(-3.76143050694799,-2.21855034327406,
5.10019281208991));
#21538=CARTESIAN_POINT('Ctrl Pts',(-3.53510505567384,-2.16596525884485,
5.0890790230331));
#21539=CARTESIAN_POINT('Ctrl Pts',(-3.36817872512274,-2.32759432716241,
5.07796523397629));
#21540=CARTESIAN_POINT('Ctrl Pts',(-3.41344101541272,-2.5554973786501,5.06685144491949));
#21541=CARTESIAN_POINT('Ctrl Pts',(-3.62946287054873,-2.64107179130501,
5.05573765586269));
#21542=CARTESIAN_POINT('Ctrl Pts',(-3.81851702088083,-2.50599052171118,
5.04462386680588));
#21543=CARTESIAN_POINT('Ctrl Pts',(-3.8075600664755,-2.27389489448153,5.03351007774907));
#21544=CARTESIAN_POINT('Ctrl Pts',(-3.60662102802227,-2.15722471599323,
5.02239628869228));
#21545=CARTESIAN_POINT('Ctrl Pts',(-3.39962168818772,-2.262769500459,5.01128249963546));
#21546=CARTESIAN_POINT('Ctrl Pts',(-3.37603088927244,-2.49392292132789,
5.00016871057867));
#21547=CARTESIAN_POINT('Ctrl Pts',(-3.55744155755193,-2.63910762521254,
4.98905492152185));
#21548=CARTESIAN_POINT('Ctrl Pts',(-3.77780645076812,-2.56543440904132,
4.97794113246506));
#21549=CARTESIAN_POINT('Ctrl Pts',(-3.83542308317469,-2.34033720163832,
4.96682734340825));
#21550=CARTESIAN_POINT('Ctrl Pts',(-3.67755429765177,-2.16985003043886,
4.95571355435145));
#21551=CARTESIAN_POINT('Ctrl Pts',(-3.44869918397279,-2.21002173633656,
4.94459976529464));
#21552=CARTESIAN_POINT('Ctrl Pts',(-3.3583314230664,-2.42408270152555,4.93348597623784));
#21553=CARTESIAN_POINT('Ctrl Pts',(-3.48916565133794,-2.61610049686178,
4.92237218718103));
#21554=CARTESIAN_POINT('Ctrl Pts',(-3.7214478158856,-2.61031905668909,4.91125839812423));
#21555=CARTESIAN_POINT('Ctrl Pts',(-3.8425674172419,-2.41203019874106,4.90014460906743));
#21556=CARTESIAN_POINT('Ctrl Pts',(-3.74166231069475,-2.20272996345734,
4.88903082001062));
#21557=CARTESIAN_POINT('Ctrl Pts',(-3.511092084609,-2.17399322981363,4.87791703095382));
#21558=CARTESIAN_POINT('Ctrl Pts',(-3.36190028176488,-2.35212305601353,
4.86680324189701));
#21559=CARTESIAN_POINT('Ctrl Pts',(-3.43064385125587,-2.57407519200526,
4.85568945284021));
#21560=CARTESIAN_POINT('Ctrl Pts',(-3.6544010243217,-2.63669433060785,4.84457566378341));
#21561=CARTESIAN_POINT('Ctrl Pts',(-3.82836432287631,-2.48266446410869,
4.8334618747266));
#21562=CARTESIAN_POINT('Ctrl Pts',(-3.79330316687467,-2.25297087613211,
4.8223480856698));
#21563=CARTESIAN_POINT('Ctrl Pts',(-3.58130943002562,-2.15785471265546,
4.81123429661298));
#21564=CARTESIAN_POINT('Ctrl Pts',(-3.38642338383962,-2.28437687679961,
4.8001205075562));
#21565=CARTESIAN_POINT('Ctrl Pts',(-3.38702643654876,-2.51673019686447,
4.78900671849938));
#21566=CARTESIAN_POINT('Ctrl Pts',(-3.58256660716932,-2.64223904392882,
4.77789292944258));
#21567=CARTESIAN_POINT('Ctrl Pts',(-3.79406375995591,-2.54602374690751,
4.76677914038577));
#21568=CARTESIAN_POINT('Ctrl Pts',(-3.82793215242214,-2.31615125831984,
4.75566535132897));
#21569=CARTESIAN_POINT('Ctrl Pts',(-3.65317166084996,-2.16302647390142,
4.74455156227217));
#21570=CARTESIAN_POINT('Ctrl Pts',(-3.42974254509416,-2.22680624538361,
4.73343777321536));
#21571=CARTESIAN_POINT('Ctrl Pts',(-3.36215200866455,-2.44911222461694,
4.72232398415856));
#21572=CARTESIAN_POINT('Ctrl Pts',(-3.51226643608395,-2.62646522768789,
4.71121019510176));
#21573=CARTESIAN_POINT('Ctrl Pts',(-3.74268438952201,-2.59653203956573,
4.70009640604495));
#21574=CARTESIAN_POINT('Ctrl Pts',(-3.84250170307953,-2.38671084680417,
4.68898261698815));
#21575=CARTESIAN_POINT('Ctrl Pts',(-3.72035445765201,-2.18905336667194,
4.67786882793134));
#21576=CARTESIAN_POINT('Ctrl Pts',(-3.4880454122232,-2.18447773232253,4.66675503887454));
#21577=CARTESIAN_POINT('Ctrl Pts',(-3.35820967063793,-2.37717207376684,
4.65564124981773));
#21578=CARTESIAN_POINT('Ctrl Pts',(-3.4496873596065,-2.5907610749791,4.64452746076093));
#21579=CARTESIAN_POINT('Ctrl Pts',(-3.67874791298872,-2.62974430088435,
4.63341367170412));
#21580=CARTESIAN_POINT('Ctrl Pts',(-3.83572960854991,-2.4584399627144,4.62229988264733));
#21581=CARTESIAN_POINT('Ctrl Pts',(-3.77694532005055,-2.23364486391404,
4.61118609359051));
#21582=CARTESIAN_POINT('Ctrl Pts',(-3.55620097341096,-2.16111650777606,
4.60007230453371));
#21583=CARTESIAN_POINT('Ctrl Pts',(-3.37554637252617,-2.307240921179,4.58895851547691));
#21584=CARTESIAN_POINT('Ctrl Pts',(-3.40033672233922,-2.53826877141577,
4.57784472642011));
#21585=CARTESIAN_POINT('Ctrl Pts',(-3.60788113454322,-2.64273764704216,
4.5667309373633));
#21586=CARTESIAN_POINT('Ctrl Pts',(-3.8082118548967,-2.52502600161686,4.5556171483065));
#21587=CARTESIAN_POINT('Ctrl Pts',(-3.8179639032302,-2.29287663878378,4.54450335924969));
#21588=CARTESIAN_POINT('Ctrl Pts',(-3.62821111895818,-2.15877850380716,
4.53338957019289));
#21589=CARTESIAN_POINT('Ctrl Pts',(-3.4126363777684,-2.24547313898512,4.52227578113608));
#21590=CARTESIAN_POINT('Ctrl Pts',(-3.3685576844537,-2.47360796440317,4.51116199207928));
#21591=CARTESIAN_POINT('Ctrl Pts',(-3.53632076809686,-2.63436858142862,
4.50004820302248));
#21592=CARTESIAN_POINT('Ctrl Pts',(-3.76237017326276,-2.5806089855676,4.48893441396567));
#21593=CARTESIAN_POINT('Ctrl Pts',(-3.83980032066171,-2.36153592172191,
4.47782062490887));
#21594=CARTESIAN_POINT('Ctrl Pts',(-3.69773850858379,-2.17766949547173,
4.46670683585206));
#21595=CARTESIAN_POINT('Ctrl Pts',(-3.46621554409366,-2.19730464027232,
4.45559304679525));
#21596=CARTESIAN_POINT('Ctrl Pts',(-3.35714698343348,-2.40246926898597,
4.44447925773846));
#21597=CARTESIAN_POINT('Ctrl Pts',(-3.47036459479899,-2.60537350263611,
4.43336546868164));
#21598=CARTESIAN_POINT('Ctrl Pts',(-3.70223885894321,-2.62029753112878,
4.42225167962485));
#21599=CARTESIAN_POINT('Ctrl Pts',(-3.84053294381125,-2.43357974806573,
4.41113789056804));
#21600=CARTESIAN_POINT('Ctrl Pts',(-3.75866408131995,-2.21612800906199,
4.40002410151124));
#21601=CARTESIAN_POINT('Ctrl Pts',(-3.53156901893564,-2.16697244735031,
4.38891031245443));
#21602=CARTESIAN_POINT('Ctrl Pts',(-3.36710794136624,-2.33111753922242,
4.37779652339762));
#21603=CARTESIAN_POINT('Ctrl Pts',(-3.41581894666805,-2.55829572590735,
4.36668273434083));
#21604=CARTESIAN_POINT('Ctrl Pts',(-3.63310626972243,-2.64061568298545,
4.35556894528402));
#21605=CARTESIAN_POINT('Ctrl Pts',(-3.82010444677879,-2.50263400904229,
4.34445515622722));
#21606=CARTESIAN_POINT('Ctrl Pts',(-3.80561164731632,-2.27083721711559,
4.33334136717041));
#21607=CARTESIAN_POINT('Ctrl Pts',(-3.60297473301061,-2.15700944143379,
4.32222757811361));
#21608=CARTESIAN_POINT('Ctrl Pts',(-3.39749761512046,-2.26611614077921,
4.3111137890568));
#21609=CARTESIAN_POINT('Ctrl Pts',(-3.38436282049399,-2.419721374356,4.30370459635227));
#21610=CARTESIAN_POINT('Ctrl Pts',(-3.41173724903364,-2.48232321801035,
4.3));
#21611=CARTESIAN_POINT('Ctrl Pts',(-3.47309291201476,-2.29206413469515,
5.2));
#21612=CARTESIAN_POINT('Ctrl Pts',(-3.46488110023315,-2.2997248835417,5.2));
#21613=CARTESIAN_POINT('Ctrl Pts',(-3.45756393061001,-2.3082260406838,5.2));
#21614=CARTESIAN_POINT('Ctrl Pts',(-3.45114583189458,-2.31737340047652,
5.2));
#21615=CARTESIAN_POINT('Ctrl Pts',(-3.44637506584917,-2.32417290846779,
5.2));
#21616=CARTESIAN_POINT('Ctrl Pts',(-3.44210141208336,-2.33133076253531,
5.2));
#21617=CARTESIAN_POINT('Ctrl Pts',(-3.43833687158849,-2.33878162457801,
5.2));
#21618=CARTESIAN_POINT('Ctrl Pts',(-3.43611957198332,-2.34317015313494,
5.2));
#21619=CARTESIAN_POINT('Ctrl Pts',(-3.43407750155671,-2.34766554493455,
5.2));
#21620=CARTESIAN_POINT('Ctrl Pts',(-3.43222557143088,-2.35222601439271,
5.2));
#21621=CARTESIAN_POINT('Ctrl Pts',(-3.42766723914997,-2.36345113290954,
5.2));
#21622=CARTESIAN_POINT('Ctrl Pts',(-3.42424191788099,-2.37509439510727,
5.2));
#21623=CARTESIAN_POINT('Ctrl Pts',(-3.42197769676804,-2.38695730471617,
5.2));
#21624=CARTESIAN_POINT('Ctrl Pts',(-3.42053881602809,-2.39449601728207,
5.2));
#21625=CARTESIAN_POINT('Ctrl Pts',(-3.41956956713255,-2.40212431376417,
5.2));
#21626=CARTESIAN_POINT('Ctrl Pts',(-3.41908672349853,-2.40979637190619,
5.2));
#21627=CARTESIAN_POINT('Ctrl Pts',(-3.4188613967758,-2.41337666083611,5.2));
#21628=CARTESIAN_POINT('Ctrl Pts',(-3.41874254028701,-2.41696303084227,
5.2));
#21629=CARTESIAN_POINT('Ctrl Pts',(-3.4187313001846,-2.42054068183377,5.2));
#21630=CARTESIAN_POINT('Ctrl Pts',(-3.41869625236243,-2.43169617411961,
5.2));
#21631=CARTESIAN_POINT('Ctrl Pts',(-3.41970314531555,-2.44279404991157,
5.2));
#21632=CARTESIAN_POINT('Ctrl Pts',(-3.4217856982914,-2.45369315923086,5.2));
#21633=CARTESIAN_POINT('Ctrl Pts',(-3.42294608022389,-2.45976605614203,
5.2));
#21634=CARTESIAN_POINT('Ctrl Pts',(-3.42444095669484,-2.46577748192705,
5.2));
#21635=CARTESIAN_POINT('Ctrl Pts',(-3.42625159798616,-2.47171129566944,
5.2));
#21636=CARTESIAN_POINT('Ctrl Pts',(-3.42738424188737,-2.4754231838156,5.2));
#21637=CARTESIAN_POINT('Ctrl Pts',(-3.4286411006463,-2.47910621955531,5.2));
#21638=CARTESIAN_POINT('Ctrl Pts',(-3.43001647345192,-2.48275158788973,
5.2));
#21639=CARTESIAN_POINT('Ctrl Pts',(-3.43439826051469,-2.49436533198986,
5.2));
#21640=CARTESIAN_POINT('Ctrl Pts',(-3.43994736167241,-2.50551615790537,
5.2));
#21641=CARTESIAN_POINT('Ctrl Pts',(-3.44649835855225,-2.51608152365555,
5.2));
#21642=CARTESIAN_POINT('Ctrl Pts',(-3.45083933347942,-2.52308259366964,
5.2));
#21643=CARTESIAN_POINT('Ctrl Pts',(-3.45562142913928,-2.5298267361278,5.2));
#21644=CARTESIAN_POINT('Ctrl Pts',(-3.46080806253422,-2.53627607801171,
5.2));
#21645=CARTESIAN_POINT('Ctrl Pts',(-3.46351819008795,-2.53964599792162,
5.2));
#21646=CARTESIAN_POINT('Ctrl Pts',(-3.46634016652161,-2.54293674743321,
5.2));
#21647=CARTESIAN_POINT('Ctrl Pts',(-3.46926561316249,-2.5461381198978,5.2));
#21648=CARTESIAN_POINT('Ctrl Pts',(-3.47553204021621,-2.55299559141714,
5.2));
#21649=CARTESIAN_POINT('Ctrl Pts',(-3.48224800724127,-2.55941730873493,
5.2));
#21650=CARTESIAN_POINT('Ctrl Pts',(-3.48935943070669,-2.56535251864156,
5.2));
#21651=CARTESIAN_POINT('Ctrl Pts',(-3.49388595591638,-2.56913036669094,
5.2));
#21652=CARTESIAN_POINT('Ctrl Pts',(-3.49857295100653,-2.57271103243443,
5.2));
#21653=CARTESIAN_POINT('Ctrl Pts',(-3.50340866428261,-2.5760800097667,5.2));
#21654=CARTESIAN_POINT('Ctrl Pts',(-3.50748115648314,-2.57891726109367,
5.2));
#21655=CARTESIAN_POINT('Ctrl Pts',(-3.51165212725609,-2.58159933242901,
5.2));
#21656=CARTESIAN_POINT('Ctrl Pts',(-3.51591076075252,-2.58411660325874,
5.2));
#21657=CARTESIAN_POINT('Ctrl Pts',(-3.52463384142318,-2.58927280102407,
5.2));
#21658=CARTESIAN_POINT('Ctrl Pts',(-3.53372795938425,-2.593741186929,5.2));
#21659=CARTESIAN_POINT('Ctrl Pts',(-3.54313434616876,-2.59744798259885,
5.2));
#21660=CARTESIAN_POINT('Ctrl Pts',(-3.54437365456163,-2.59793635960157,
5.2));
#21661=CARTESIAN_POINT('Ctrl Pts',(-3.54561839868079,-2.59841149645932,
5.2));
#21662=CARTESIAN_POINT('Ctrl Pts',(-3.54686838721289,-2.59887345127292,
5.2));
#21663=CARTESIAN_POINT('Ctrl Pts',(-3.76673281282141,-2.40013003219325,
5.08714803633902));
#21664=CARTESIAN_POINT('Ctrl Pts',(-3.76680596527292,-2.4086546123928,5.08771939403667));
#21665=CARTESIAN_POINT('Ctrl Pts',(-3.76620865763489,-2.417168907206,5.08829075173431));
#21666=CARTESIAN_POINT('Ctrl Pts',(-3.76490523910227,-2.42557368984471,
5.08886210943196));
#21667=CARTESIAN_POINT('Ctrl Pts',(-3.75645407171393,-2.48006902128643,
5.09256670578423));
#21668=CARTESIAN_POINT('Ctrl Pts',(-3.71831780296444,-2.52996042999443,
5.09627130213649));
#21669=CARTESIAN_POINT('Ctrl Pts',(-3.66794964380788,-2.55241564320215,
5.09997589848876));
#21670=CARTESIAN_POINT('Ctrl Pts',(-3.61758148465131,-2.57487085640986,
5.10368049484103));
#21671=CARTESIAN_POINT('Ctrl Pts',(-3.55498143508767,-2.56988987411729,
5.1073850911933));
#21672=CARTESIAN_POINT('Ctrl Pts',(-3.50879890030286,-2.53975064250981,
5.11108968754557));
#21673=CARTESIAN_POINT('Ctrl Pts',(-3.46261636551805,-2.50961141090233,
5.11479428389784));
#21674=CARTESIAN_POINT('Ctrl Pts',(-3.43285134551208,-2.45431392997993,
5.1184988802501));
#21675=CARTESIAN_POINT('Ctrl Pts',(-3.4331256950702,-2.3991686665445,5.12220347660237));
#21676=CARTESIAN_POINT('Ctrl Pts',(-3.43340004462832,-2.34402340310906,
5.12590807295464));
#21677=CARTESIAN_POINT('Ctrl Pts',(-3.46371376375052,-2.28903035716059,
5.12961266930691));
#21678=CARTESIAN_POINT('Ctrl Pts',(-3.51019415842152,-2.25935087796534,
5.13331726565918));
#21679=CARTESIAN_POINT('Ctrl Pts',(-3.55667455309252,-2.22967139877009,
5.13702186201145));
#21680=CARTESIAN_POINT('Ctrl Pts',(-3.61932162331232,-2.22530548632806,
5.14072645836371));
#21681=CARTESIAN_POINT('Ctrl Pts',(-3.66946347831689,-2.24826430176485,
5.14443105471598));
#21682=CARTESIAN_POINT('Ctrl Pts',(-3.71960533332146,-2.27122311720164,
5.14813565106825));
#21683=CARTESIAN_POINT('Ctrl Pts',(-3.7572419731108,-2.32150666051725,5.15184024742051));
#21684=CARTESIAN_POINT('Ctrl Pts',(-3.76515098200617,-2.37607618706626,
5.15554484377278));
#21685=CARTESIAN_POINT('Ctrl Pts',(-3.76629187681735,-2.3839479811825,5.15607924129486));
#21686=CARTESIAN_POINT('Ctrl Pts',(-3.7668141752375,-2.39190896147606,5.15661363881694));
#21687=CARTESIAN_POINT('Ctrl Pts',(-3.76674783764939,-2.3998784327954,5.15714803633902));
#21688=CARTESIAN_POINT('Ctrl Pts',(-3.65301702171886,-2.59851743256717,
5.2));
#21689=CARTESIAN_POINT('Ctrl Pts',(-3.71902879097456,-2.58088801151799,
5.19629540364773));
#21690=CARTESIAN_POINT('Ctrl Pts',(-3.83093278328674,-2.47484748886485,
5.1888862109432));
#21691=CARTESIAN_POINT('Ctrl Pts',(-3.78812295700318,-2.24617213689742,
5.17777242188639));
#21692=CARTESIAN_POINT('Ctrl Pts',(-3.5727867642971,-2.15871465280967,5.16665863282959));
#21693=CARTESIAN_POINT('Ctrl Pts',(-3.38252461999799,-2.29190667528476,
5.15554484377278));
#21694=CARTESIAN_POINT('Ctrl Pts',(-3.39123766053156,-2.52413789941101,
5.14443105471598));
#21695=CARTESIAN_POINT('Ctrl Pts',(-3.59107442597796,-2.64269432067786,
5.13331726565918));
#21696=CARTESIAN_POINT('Ctrl Pts',(-3.79906030223171,-2.53913483234337,
5.12220347660237));
#21697=CARTESIAN_POINT('Ctrl Pts',(-3.82485429799751,-2.30821119218956,
5.11108968754557));
#21698=CARTESIAN_POINT('Ctrl Pts',(-3.64483147519039,-2.16130911215383,
5.09997589848876));
#21699=CARTESIAN_POINT('Ctrl Pts',(-3.42377645640768,-2.23288040078699,
5.08886210943196));
#21700=CARTESIAN_POINT('Ctrl Pts',(-3.36401956629289,-2.45741970591997,
5.07774832037515));
#21701=CARTESIAN_POINT('Ctrl Pts',(-3.52025888222192,-2.62940132794335,
5.06663453131835));
#21702=CARTESIAN_POINT('Ctrl Pts',(-3.74948582853024,-2.5914096999913,5.05552074226155));
#21703=CARTESIAN_POINT('Ctrl Pts',(-3.84188686003135,-2.37821840959849,
5.04440695320474));
#21704=CARTESIAN_POINT('Ctrl Pts',(-3.71288602579316,-2.18496415245566,
5.03329316414794));
#21705=CARTESIAN_POINT('Ctrl Pts',(-3.4805593716682,-2.1885345970333,5.02217937509112));
#21706=CARTESIAN_POINT('Ctrl Pts',(-3.35755805936012,-2.38566174720256,
5.01106558603434));
#21707=CARTESIAN_POINT('Ctrl Pts',(-3.45646661470834,-2.59591285074103,
4.99995179697752));
#21708=CARTESIAN_POINT('Ctrl Pts',(-3.68675290044432,-2.62684270619768,
4.98883800792072));
#21709=CARTESIAN_POINT('Ctrl Pts',(-3.83763327503031,-2.45014085710183,
4.97772421886392));
#21710=CARTESIAN_POINT('Ctrl Pts',(-3.77100521680217,-2.22754451436212,
4.96661042980711));
#21711=CARTESIAN_POINT('Ctrl Pts',(-3.54785414492032,-2.16279863265717,
4.9554966407503));
#21712=CARTESIAN_POINT('Ctrl Pts',(-3.37243276525931,-2.31516585290104,
4.94438285169351));
#21713=CARTESIAN_POINT('Ctrl Pts',(-3.40530625649813,-2.54518272988275,
4.9332690626367));
#21714=CARTESIAN_POINT('Ctrl Pts',(-3.61638513906469,-2.64231220781178,
4.9221552735799));
#21715=CARTESIAN_POINT('Ctrl Pts',(-3.81246651806354,-2.51765057387683,
4.91104148452309));
#21716=CARTESIAN_POINT('Ctrl Pts',(-3.81407488352551,-2.2853020354474,4.89992769546629));
#21717=CARTESIAN_POINT('Ctrl Pts',(-3.61973808033182,-2.15793784472475,
4.88881390640949));
#21718=CARTESIAN_POINT('Ctrl Pts',(-3.4073347883606,-2.25213588990288,4.87770011735268));
#21719=CARTESIAN_POINT('Ctrl Pts',(-3.37128014957741,-2.48167563194308,
4.86658632829587));
#21720=CARTESIAN_POINT('Ctrl Pts',(-3.54457538374435,-2.63645674180255,
4.85547253923907));
#21721=CARTESIAN_POINT('Ctrl Pts',(-3.76860139772859,-2.57480631428759,
4.84435875018227));
#21722=CARTESIAN_POINT('Ctrl Pts',(-3.83830464030165,-2.35315368486712,
4.83324496112546));
#21723=CARTESIAN_POINT('Ctrl Pts',(-3.68988494304833,-2.17438001896094,
4.82213117206866));
#21724=CARTESIAN_POINT('Ctrl Pts',(-3.45919253805822,-2.20211888040452,
4.81101738301185));
#21725=CARTESIAN_POINT('Ctrl Pts',(-3.35738279984868,-2.41098057473832,
4.79990359395505));
#21726=CARTESIAN_POINT('Ctrl Pts',(-3.47764333640382,-2.60979162448597,
4.78878980489824));
#21727=CARTESIAN_POINT('Ctrl Pts',(-3.7098983147675,-2.61657802114276,4.77767601584144));
#21728=CARTESIAN_POINT('Ctrl Pts',(-3.84156211929281,-2.42512809888577,
4.76656222678463));
#21729=CARTESIAN_POINT('Ctrl Pts',(-3.75212137652867,-2.21067814274661,
4.75544843772783));
#21730=CARTESIAN_POINT('Ctrl Pts',(-3.52344221265408,-2.16951662960737,
4.74433464867103));
#21731=CARTESIAN_POINT('Ctrl Pts',(-3.36483725976158,-2.33931915924769,
4.73322085961422));
#21732=CARTESIAN_POINT('Ctrl Pts',(-3.42147942993616,-2.56466355059616,
4.72210707055742));
#21733=CARTESIAN_POINT('Ctrl Pts',(-3.64152350245114,-2.63928952667227,
4.71099328150061));
#21734=CARTESIAN_POINT('Ctrl Pts',(-3.82356064226404,-2.49489108525746,
4.69987949244381));
#21735=CARTESIAN_POINT('Ctrl Pts',(-3.80097019086255,-2.26363775736839,
4.688765703387));
#21736=CARTESIAN_POINT('Ctrl Pts',(-3.59442944460758,-2.15719833661306,
4.6776519143302));
#21737=CARTESIAN_POINT('Ctrl Pts',(-3.3929874908777,-2.27299803191391,4.6665381252734));
#21738=CARTESIAN_POINT('Ctrl Pts',(-3.38102643442896,-2.50504406890429,
4.65542433621659));
#21739=CARTESIAN_POINT('Ctrl Pts',(-3.5694943658766,-2.64094207834572,4.64431054715979));
#21740=CARTESIAN_POINT('Ctrl Pts',(-3.78588445019465,-2.55630307100846,
4.63319675810299));
#21741=CARTESIAN_POINT('Ctrl Pts',(-3.83213238917682,-2.32859809017945,
4.62208296904618));
#21742=CARTESIAN_POINT('Ctrl Pts',(-3.66590691978443,-2.16624808716256,
4.61096917998938));
#21743=CARTESIAN_POINT('Ctrl Pts',(-3.4393560992794,-2.21785386089149,4.59985539093257));
#21744=CARTESIAN_POINT('Ctrl Pts',(-3.35984446292695,-2.43618006142673,
4.58874160187577));
#21745=CARTESIAN_POINT('Ctrl Pts',(-3.50014991321196,-2.62139024142312,
4.57762781281897));
#21746=CARTESIAN_POINT('Ctrl Pts',(-3.73184928030013,-2.60395942271916,
4.56651402376216));
#21747=CARTESIAN_POINT('Ctrl Pts',(-3.84286550587893,-2.3998422313225,4.55540023470536));
#21748=CARTESIAN_POINT('Ctrl Pts',(-3.73158417960078,-2.19586944742698,
4.54428644564855));
#21749=CARTESIAN_POINT('Ctrl Pts',(-3.49986236155564,-2.17873967321655,
4.53317265659175));
#21750=CARTESIAN_POINT('Ctrl Pts',(-3.35979765944108,-2.36413198553984,
4.52205886753494));
#21751=CARTESIAN_POINT('Ctrl Pts',(-3.43959288407154,-2.58235469793693,
4.51094507847814));
#21752=CARTESIAN_POINT('Ctrl Pts',(-3.66621056034765,-2.6336660879353,4.49983128942134));
#21753=CARTESIAN_POINT('Ctrl Pts',(-3.83222496126862,-2.47110025635944,
4.48871750036453));
#21754=CARTESIAN_POINT('Ctrl Pts',(-3.78568121870704,-2.24345555647604,
4.47760371130773));
#21755=CARTESIAN_POINT('Ctrl Pts',(-3.56918135654791,-2.15909775573836,
4.46648992225092));
#21756=CARTESIAN_POINT('Ctrl Pts',(-3.38089013692747,-2.29524052189659,
4.45537613319412));
#21757=CARTESIAN_POINT('Ctrl Pts',(-3.39315268252002,-2.52727080497827,
4.44426234413731));
#21758=CARTESIAN_POINT('Ctrl Pts',(-3.59474487821944,-2.64280871984201,
4.43314855508051));
#21759=CARTESIAN_POINT('Ctrl Pts',(-3.80114723737323,-2.53610097383652,
4.42203476602371));
#21760=CARTESIAN_POINT('Ctrl Pts',(-3.82343706699101,-2.30481863511631,
4.4109209769669));
#21761=CARTESIAN_POINT('Ctrl Pts',(-3.64121277969171,-2.16065653443092,
4.3998071879101));
#21762=CARTESIAN_POINT('Ctrl Pts',(-3.42126523797479,-2.23556891230323,
4.38869339885329));
#21763=CARTESIAN_POINT('Ctrl Pts',(-3.36491711226222,-2.46098554747977,
4.37757960979649));
#21764=CARTESIAN_POINT('Ctrl Pts',(-3.52374009350676,-2.63058418685777,
4.36646582073969));
#21765=CARTESIAN_POINT('Ctrl Pts',(-3.7523704915333,-2.58912096342209,4.35535203168288));
#21766=CARTESIAN_POINT('Ctrl Pts',(-3.84152271736619,-2.3745642740037,4.34423824262608));
#21767=CARTESIAN_POINT('Ctrl Pts',(-3.70962995644976,-2.18326697275372,
4.33312445356927));
#21768=CARTESIAN_POINT('Ctrl Pts',(-3.47734459894833,-2.19039236572141,
4.32201066451247));
#21769=CARTESIAN_POINT('Ctrl Pts',(-3.35742142491826,-2.38928487622609,
4.31089687545566));
#21770=CARTESIAN_POINT('Ctrl Pts',(-3.45934320255763,-2.59816388104693,
4.29978308639886));
#21771=CARTESIAN_POINT('Ctrl Pts',(-3.69040341475663,-2.62529829024268,
4.28866929734205));
#21772=CARTESIAN_POINT('Ctrl Pts',(-3.7885754343637,-2.50643134569448,4.28126010463752));
#21773=CARTESIAN_POINT('Ctrl Pts',(-3.80166758614466,-2.43937207542898,
4.27755550828525));
#21774=CARTESIAN_POINT('Ctrl Pts',(-3.64967348970877,-2.58599788000028,
5.20748149723825));
#21775=CARTESIAN_POINT('Ctrl Pts',(-3.71152220988337,-2.5694802628904,5.20377690088598));
#21776=CARTESIAN_POINT('Ctrl Pts',(-3.81636894835099,-2.47012721287082,
5.19636770818145));
#21777=CARTESIAN_POINT('Ctrl Pts',(-3.77625893469146,-2.25587333035667,
5.18525391912464));
#21778=CARTESIAN_POINT('Ctrl Pts',(-3.57450297395432,-2.17393137483105,
5.17414013006784));
#21779=CARTESIAN_POINT('Ctrl Pts',(-3.39623976035988,-2.29872360840445,
5.16302634101103));
#21780=CARTESIAN_POINT('Ctrl Pts',(-3.40440331076774,-2.5163091110919,5.15191255195424));
#21781=CARTESIAN_POINT('Ctrl Pts',(-3.59163731958239,-2.62738874138378,
5.14079876289742));
#21782=CARTESIAN_POINT('Ctrl Pts',(-3.78650651345082,-2.53036025862013,
5.12968497384062));
#21783=CARTESIAN_POINT('Ctrl Pts',(-3.81067380428838,-2.31399987678807,
5.11857118478382));
#21784=CARTESIAN_POINT('Ctrl Pts',(-3.64200416676191,-2.17636221393428,
5.10745739572701));
#21785=CARTESIAN_POINT('Ctrl Pts',(-3.43489003917469,-2.24341984097745,
5.09634360667021));
#21786=CARTESIAN_POINT('Ctrl Pts',(-3.37890173259108,-2.45379851750672,
5.08522981761341));
#21787=CARTESIAN_POINT('Ctrl Pts',(-3.52528777617272,-2.61493407462981,
5.07411602855659));
#21788=CARTESIAN_POINT('Ctrl Pts',(-3.74005846658983,-2.57933839839392,
5.0630022394998));
#21789=CARTESIAN_POINT('Ctrl Pts',(-3.82663220344909,-2.37959207115806,
5.05188845044299));
#21790=CARTESIAN_POINT('Ctrl Pts',(-3.7057668397564,-2.19852544308029,5.04077466138619));
#21791=CARTESIAN_POINT('Ctrl Pts',(-3.48809192538747,-2.20187071665909,
5.02966087232937));
#21792=CARTESIAN_POINT('Ctrl Pts',(-3.37284772224266,-2.38656599277582,
5.01854708327259));
#21793=CARTESIAN_POINT('Ctrl Pts',(-3.46551858429622,-2.58355755679196,
5.00743329421577));
#21794=CARTESIAN_POINT('Ctrl Pts',(-3.68128180662955,-2.61253681301776,
4.99631950515897));
#21795=CARTESIAN_POINT('Ctrl Pts',(-3.82264687187209,-2.44697871114761,
4.98520571610216));
#21796=CARTESIAN_POINT('Ctrl Pts',(-3.76022072914644,-2.23842046359223,
4.97409192704536));
#21797=CARTESIAN_POINT('Ctrl Pts',(-3.5511427365839,-2.17775779744681,4.96297813798855));
#21798=CARTESIAN_POINT('Ctrl Pts',(-3.38678435101677,-2.32051594004622,
4.95186434893176));
#21799=CARTESIAN_POINT('Ctrl Pts',(-3.41758466713793,-2.53602674395714,
4.94075055987494));
#21800=CARTESIAN_POINT('Ctrl Pts',(-3.6153518060864,-2.62703072656315,4.92963677081815));
#21801=CARTESIAN_POINT('Ctrl Pts',(-3.79906726285858,-2.51023091039877,
4.91852298176134));
#21802=CARTESIAN_POINT('Ctrl Pts',(-3.80057419634206,-2.29253549186461,
4.90740919270453));
#21803=CARTESIAN_POINT('Ctrl Pts',(-3.61849329325651,-2.17320355634632,
4.89629540364773));
#21804=CARTESIAN_POINT('Ctrl Pts',(-3.41948526912059,-2.26146097775627,
4.88518161459093));
#21805=CARTESIAN_POINT('Ctrl Pts',(-3.38570442533712,-2.47652473736257,
4.87406782553412));
#21806=CARTESIAN_POINT('Ctrl Pts',(-3.54807075131856,-2.62154453701271,
4.86295403647732));
#21807=CARTESIAN_POINT('Ctrl Pts',(-3.75796850753643,-2.56378210944851,
4.85184024742052));
#21808=CARTESIAN_POINT('Ctrl Pts',(-3.82327589732119,-2.35610805969097,
4.84072645836371));
#21809=CARTESIAN_POINT('Ctrl Pts',(-3.68421632616712,-2.18860880066658,
4.8296126693069));
#21810=CARTESIAN_POINT('Ctrl Pts',(-3.46807259659411,-2.2145983037314,4.81849888025011));
#21811=CARTESIAN_POINT('Ctrl Pts',(-3.37268351551706,-2.41028808198908,
4.80738509119329));
#21812=CARTESIAN_POINT('Ctrl Pts',(-3.48535979063151,-2.59656106212739,
4.79627130213649));
#21813=CARTESIAN_POINT('Ctrl Pts',(-3.70296754948933,-2.60291947294643,
4.78515751307969));
#21814=CARTESIAN_POINT('Ctrl Pts',(-3.82632794256814,-2.42354338891427,
4.77404372402288));
#21815=CARTESIAN_POINT('Ctrl Pts',(-3.74252780308088,-2.22261777400868,
4.76292993496608));
#21816=CARTESIAN_POINT('Ctrl Pts',(-3.52827034905847,-2.18405212220422,
4.75181614590928));
#21817=CARTESIAN_POINT('Ctrl Pts',(-3.37966785801241,-2.34314601196173,
4.74070235685247));
#21818=CARTESIAN_POINT('Ctrl Pts',(-3.43273787526403,-2.55427900173875,
4.72958856779567));
#21819=CARTESIAN_POINT('Ctrl Pts',(-3.63890481216799,-2.62419867158141,
4.71847477873886));
#21820=CARTESIAN_POINT('Ctrl Pts',(-3.80946173328402,-2.48890675473974,
4.70736098968206));
#21821=CARTESIAN_POINT('Ctrl Pts',(-3.78829595446756,-2.27223747701361,
4.69624720062526));
#21822=CARTESIAN_POINT('Ctrl Pts',(-3.59478075310558,-2.17251068550248,
4.68513341156845));
#21823=CARTESIAN_POINT('Ctrl Pts',(-3.40604278761636,-2.28100744345521,
4.67401962251164));
#21824=CARTESIAN_POINT('Ctrl Pts',(-3.39483605824625,-2.4984194378808,4.66290583345485));
#21825=CARTESIAN_POINT('Ctrl Pts',(-3.57141821148077,-2.62574700466167,
4.65179204439804));
#21826=CARTESIAN_POINT('Ctrl Pts',(-3.77416159988632,-2.54644577793071,
4.64067825534124));
#21827=CARTESIAN_POINT('Ctrl Pts',(-3.81749290078935,-2.33310106985138,
4.62956446628443));
#21828=CARTESIAN_POINT('Ctrl Pts',(-3.66175048306201,-2.18098971122316,
4.61845067722763));
#21829=CARTESIAN_POINT('Ctrl Pts',(-3.44948714789117,-2.22934095365678,
4.60733688817083));
#21830=CARTESIAN_POINT('Ctrl Pts',(-3.37498993318483,-2.43389835661598,
4.59622309911401));
#21831=CARTESIAN_POINT('Ctrl Pts',(-3.50644698442724,-2.60742820932623,
4.58510931005722));
#21832=CARTESIAN_POINT('Ctrl Pts',(-3.72353417177652,-2.59109666965397,
4.57399552100041));
#21833=CARTESIAN_POINT('Ctrl Pts',(-3.82754913074644,-2.39985218104442,
4.56288173194361));
#21834=CARTESIAN_POINT('Ctrl Pts',(-3.72328578972046,-2.20874299284009,
4.5517679428868));
#21835=CARTESIAN_POINT('Ctrl Pts',(-3.50617756728955,-2.19269351221351,
4.54065415383));
#21836=CARTESIAN_POINT('Ctrl Pts',(-3.37494608137275,-2.36639401102897,
4.52954036477319));
#21837=CARTESIAN_POINT('Ctrl Pts',(-3.44970899978995,-2.57085445235588,
4.51842657571639));
#21838=CARTESIAN_POINT('Ctrl Pts',(-3.66203497445559,-2.61892987644406,
4.50731278665958));
#21839=CARTESIAN_POINT('Ctrl Pts',(-3.81757963479854,-2.46661630054004,
4.49619899760278));
#21840=CARTESIAN_POINT('Ctrl Pts',(-3.77397118524436,-2.2533280717731,4.48508520854598));
#21841=CARTESIAN_POINT('Ctrl Pts',(-3.5711249421653,-2.17429031727573,4.47397141948917));
#21842=CARTESIAN_POINT('Ctrl Pts',(-3.39470835638149,-2.30184720512856,
4.46285763043237));
#21843=CARTESIAN_POINT('Ctrl Pts',(-3.40619756140558,-2.51924443916973,
4.45174384137556));
#21844=CARTESIAN_POINT('Ctrl Pts',(-3.59507629381618,-2.62749592593544,
4.44063005231876));
#21845=CARTESIAN_POINT('Ctrl Pts',(-3.78846183549484,-2.52751773117457,
4.42951626326196));
#21846=CARTESIAN_POINT('Ctrl Pts',(-3.80934595131713,-2.31082127219277,
4.41840247420515));
#21847=CARTESIAN_POINT('Ctrl Pts',(-3.63861368521871,-2.17575079119208,
4.40728868514835));
#21848=CARTESIAN_POINT('Ctrl Pts',(-3.43253719137339,-2.24593880082853,
4.39617489609154));
#21849=CARTESIAN_POINT('Ctrl Pts',(-3.37974267459471,-2.45713947835818,
4.38506110703474));
#21850=CARTESIAN_POINT('Ctrl Pts',(-3.52854944397912,-2.61604233624481,
4.37394731797793));
#21851=CARTESIAN_POINT('Ctrl Pts',(-3.74276120758414,-2.57719400158078,
4.36283352892113));
#21852=CARTESIAN_POINT('Ctrl Pts',(-3.82629102553408,-2.37616838455746,
4.35171973986432));
#21853=CARTESIAN_POINT('Ctrl Pts',(-3.70271611525743,-2.19693529644954,
4.34060595080753));
#21854=CARTESIAN_POINT('Ctrl Pts',(-3.48507989312992,-2.2036113246906,4.32949216175072));
#21855=CARTESIAN_POINT('Ctrl Pts',(-3.37271970468676,-2.38996062824249,
4.31837837269391));
#21856=CARTESIAN_POINT('Ctrl Pts',(-3.4682137593984,-2.58566662529692,4.30726458363711));
#21857=CARTESIAN_POINT('Ctrl Pts',(-3.68470210032476,-2.61108979604925,
4.2961507945803));
#21858=CARTESIAN_POINT('Ctrl Pts',(-3.77668287645173,-2.49971922570604,
4.28874160187577));
#21859=CARTESIAN_POINT('Ctrl Pts',(-3.78894936833816,-2.43688906544025,
4.2850370055235));
#21860=CARTESIAN_POINT('Ctrl Pts',(-3.64632995769868,-2.57347832743338,
5.2149629944765));
#21861=CARTESIAN_POINT('Ctrl Pts',(-3.70401562879218,-2.55807251426281,
5.21125839812423));
#21862=CARTESIAN_POINT('Ctrl Pts',(-3.80180511341523,-2.46540693687679,
5.20384920541969));
#21863=CARTESIAN_POINT('Ctrl Pts',(-3.76439491237975,-2.26557452381591,
5.19273541636289));
#21864=CARTESIAN_POINT('Ctrl Pts',(-3.57621918361154,-2.18914809685241,
5.18162162730608));
#21865=CARTESIAN_POINT('Ctrl Pts',(-3.40995490072177,-2.30554054152415,
5.17050783824929));
#21866=CARTESIAN_POINT('Ctrl Pts',(-3.41756896100391,-2.5084803227728,5.15939404919247));
#21867=CARTESIAN_POINT('Ctrl Pts',(-3.59220021318681,-2.6120831620897,5.14828026013568));
#21868=CARTESIAN_POINT('Ctrl Pts',(-3.77395272466994,-2.52158568489689,
5.13716647107886));
#21869=CARTESIAN_POINT('Ctrl Pts',(-3.79649331057924,-2.31978856138657,
5.12605268202207));
#21870=CARTESIAN_POINT('Ctrl Pts',(-3.63917685833343,-2.19141531571474,
5.11493889296526));
#21871=CARTESIAN_POINT('Ctrl Pts',(-3.44600362194169,-2.25395928116791,
5.10382510390846));
#21872=CARTESIAN_POINT('Ctrl Pts',(-3.39378389888927,-2.45017732909347,
5.09271131485166));
#21873=CARTESIAN_POINT('Ctrl Pts',(-3.53031667012352,-2.60046682131627,
5.08159752579484));
#21874=CARTESIAN_POINT('Ctrl Pts',(-3.73063110464943,-2.56726709679655,
5.07048373673805));
#21875=CARTESIAN_POINT('Ctrl Pts',(-3.81137754686683,-2.38096573271764,
5.05936994768124));
#21876=CARTESIAN_POINT('Ctrl Pts',(-3.69864765371964,-2.21208673370492,
5.04825615862444));
#21877=CARTESIAN_POINT('Ctrl Pts',(-3.49562447910673,-2.21520683628489,
5.03714236956762));
#21878=CARTESIAN_POINT('Ctrl Pts',(-3.38813738512521,-2.38747023834909,
5.02602858051084));
#21879=CARTESIAN_POINT('Ctrl Pts',(-3.47457055388411,-2.57120226284288,
5.01491479145402));
#21880=CARTESIAN_POINT('Ctrl Pts',(-3.67581071281477,-2.59823091983783,
5.00380100239722));
#21881=CARTESIAN_POINT('Ctrl Pts',(-3.80766046871388,-2.44381656519338,
4.99268721334042));
#21882=CARTESIAN_POINT('Ctrl Pts',(-3.74943624149071,-2.24929641282234,
4.9815734242836));
#21883=CARTESIAN_POINT('Ctrl Pts',(-3.55443132824748,-2.19271696223645,
4.97045963522681));
#21884=CARTESIAN_POINT('Ctrl Pts',(-3.40113593677424,-2.32586602719142,
4.95934584617));
#21885=CARTESIAN_POINT('Ctrl Pts',(-3.42986307777772,-2.52687075803154,
4.94823205711319));
#21886=CARTESIAN_POINT('Ctrl Pts',(-3.61431847310812,-2.61174924531453,
4.9371182680564));
#21887=CARTESIAN_POINT('Ctrl Pts',(-3.78566800765362,-2.50281124692072,
4.92600447899958));
#21888=CARTESIAN_POINT('Ctrl Pts',(-3.78707350915862,-2.29976894828182,
4.91489068994279));
#21889=CARTESIAN_POINT('Ctrl Pts',(-3.6172485061812,-2.18846926796789,4.90377690088598));
#21890=CARTESIAN_POINT('Ctrl Pts',(-3.43163574988059,-2.27078606560966,
4.89266311182917));
#21891=CARTESIAN_POINT('Ctrl Pts',(-3.40012870109683,-2.47137384278207,
4.88154932277237));
#21892=CARTESIAN_POINT('Ctrl Pts',(-3.55156611889279,-2.60663233222288,
4.87043553371556));
#21893=CARTESIAN_POINT('Ctrl Pts',(-3.74733561734428,-2.55275790460943,
4.85932174465877));
#21894=CARTESIAN_POINT('Ctrl Pts',(-3.80824715434074,-2.35906243451482,
4.84820795560196));
#21895=CARTESIAN_POINT('Ctrl Pts',(-3.6785477092859,-2.2028375823722,4.83709416654515));
#21896=CARTESIAN_POINT('Ctrl Pts',(-3.47695265513,-2.22707772705829,4.82598037748836));
#21897=CARTESIAN_POINT('Ctrl Pts',(-3.38798423118545,-2.40959558923983,
4.81486658843155));
#21898=CARTESIAN_POINT('Ctrl Pts',(-3.49307624485919,-2.5833304997688,4.80375279937474));
#21899=CARTESIAN_POINT('Ctrl Pts',(-3.69603678421119,-2.5892609247501,4.79263901031794));
#21900=CARTESIAN_POINT('Ctrl Pts',(-3.81109376584347,-2.42195867894277,
4.78152522126113));
#21901=CARTESIAN_POINT('Ctrl Pts',(-3.7329342296331,-2.23455740527076,4.77041143220433));
#21902=CARTESIAN_POINT('Ctrl Pts',(-3.53309848546286,-2.19858761480107,
4.75929764314753));
#21903=CARTESIAN_POINT('Ctrl Pts',(-3.39449845626323,-2.34697286467576,
4.74818385409072));
#21904=CARTESIAN_POINT('Ctrl Pts',(-3.4439963205919,-2.54389445288135,4.73707006503392));
#21905=CARTESIAN_POINT('Ctrl Pts',(-3.63628612188485,-2.60910781649055,
4.72595627597711));
#21906=CARTESIAN_POINT('Ctrl Pts',(-3.79536282430398,-2.48292242422203,
4.71484248692031));
#21907=CARTESIAN_POINT('Ctrl Pts',(-3.77562171807257,-2.28083719665882,
4.7037286978635));
#21908=CARTESIAN_POINT('Ctrl Pts',(-3.59513206160358,-2.18782303439192,
4.6926149088067));
#21909=CARTESIAN_POINT('Ctrl Pts',(-3.41909808435503,-2.28901685499652,
4.6815011197499));
#21910=CARTESIAN_POINT('Ctrl Pts',(-3.40864568206353,-2.49179480685731,
4.67038733069309));
#21911=CARTESIAN_POINT('Ctrl Pts',(-3.57334205708494,-2.61055193097763,
4.65927354163629));
#21912=CARTESIAN_POINT('Ctrl Pts',(-3.76243874957797,-2.53658848485295,
4.64815975257949));
#21913=CARTESIAN_POINT('Ctrl Pts',(-3.80285341240188,-2.33760404952332,
4.63704596352268));
#21914=CARTESIAN_POINT('Ctrl Pts',(-3.65759404633958,-2.19573133528376,
4.62593217446587));
#21915=CARTESIAN_POINT('Ctrl Pts',(-3.45961819650295,-2.24082804642207,
4.61481838540908));
#21916=CARTESIAN_POINT('Ctrl Pts',(-3.39013540344272,-2.43161665180523,
4.60370459635226));
#21917=CARTESIAN_POINT('Ctrl Pts',(-3.51274405564254,-2.59346617722935,
4.59259080729546));
#21918=CARTESIAN_POINT('Ctrl Pts',(-3.71521906325291,-2.57823391658879,
4.58147701823866));
#21919=CARTESIAN_POINT('Ctrl Pts',(-3.81223275561396,-2.39986213076634,
4.57036322918186));
#21920=CARTESIAN_POINT('Ctrl Pts',(-3.71498739984013,-2.2216165382532,4.55924944012505));
#21921=CARTESIAN_POINT('Ctrl Pts',(-3.51249277302345,-2.20664735121048,
4.54813565106825));
#21922=CARTESIAN_POINT('Ctrl Pts',(-3.39009450330442,-2.36865603651811,
4.53702186201144));
#21923=CARTESIAN_POINT('Ctrl Pts',(-3.45982511550835,-2.55935420677483,
4.52590807295464));
#21924=CARTESIAN_POINT('Ctrl Pts',(-3.65785938856352,-2.60419366495283,
4.51479428389783));
#21925=CARTESIAN_POINT('Ctrl Pts',(-3.80293430832847,-2.46213234472064,
4.50368049484103));
#21926=CARTESIAN_POINT('Ctrl Pts',(-3.76226115178167,-2.26320058707017,
4.49256670578422));
#21927=CARTESIAN_POINT('Ctrl Pts',(-3.57306852778269,-2.1894828788131,4.48145291672742));
#21928=CARTESIAN_POINT('Ctrl Pts',(-3.40852657583551,-2.30845388836054,
4.47033912767062));
#21929=CARTESIAN_POINT('Ctrl Pts',(-3.41924244029115,-2.51121807336119,
4.45922533861381));
#21930=CARTESIAN_POINT('Ctrl Pts',(-3.59540770941291,-2.61218313202887,
4.44811154955701));
#21931=CARTESIAN_POINT('Ctrl Pts',(-3.77577643361645,-2.51893448851262,
4.4369977605002));
#21932=CARTESIAN_POINT('Ctrl Pts',(-3.79525483564324,-2.31682390926922,
4.42588397144341));
#21933=CARTESIAN_POINT('Ctrl Pts',(-3.63601459074572,-2.19084504795324,
4.41477018238659));
#21934=CARTESIAN_POINT('Ctrl Pts',(-3.44380914477199,-2.25630868935384,
4.4036563933298));
#21935=CARTESIAN_POINT('Ctrl Pts',(-3.3945682369272,-2.45329340923659,4.39254260427298));
#21936=CARTESIAN_POINT('Ctrl Pts',(-3.53335879445148,-2.60150048563184,
4.38142881521619));
#21937=CARTESIAN_POINT('Ctrl Pts',(-3.73315192363498,-2.56526703973946,
4.37031502615937));
#21938=CARTESIAN_POINT('Ctrl Pts',(-3.81105933370197,-2.37777249511123,
4.35920123710258));
#21939=CARTESIAN_POINT('Ctrl Pts',(-3.69580227406509,-2.21060362014537,
4.34808744804577));
#21940=CARTESIAN_POINT('Ctrl Pts',(-3.49281518731151,-2.21683028365978,
4.33697365898897));
#21941=CARTESIAN_POINT('Ctrl Pts',(-3.38801798445527,-2.3906363802589,4.32585986993216));
#21942=CARTESIAN_POINT('Ctrl Pts',(-3.47708431623917,-2.57316936954691,
4.31474608087536));
#21943=CARTESIAN_POINT('Ctrl Pts',(-3.6790007858929,-2.59688130185582,4.30363229181855));
#21944=CARTESIAN_POINT('Ctrl Pts',(-3.76479031853975,-2.4930071057176,4.29622309911402));
#21945=CARTESIAN_POINT('Ctrl Pts',(-3.77623115053166,-2.43440605545153,
4.29251850276175));
#21946=CARTESIAN_POINT('Ctrl Pts',(-3.64298642568859,-2.56095877486649,
5.22244449171475));
#21947=CARTESIAN_POINT('Ctrl Pts',(-3.69650904770099,-2.54666476563522,
5.21873989536248));
#21948=CARTESIAN_POINT('Ctrl Pts',(-3.78724127847948,-2.46068666088276,
5.21133070265795));
#21949=CARTESIAN_POINT('Ctrl Pts',(-3.75253089006804,-2.27527571727515,
5.20021691360113));
#21950=CARTESIAN_POINT('Ctrl Pts',(-3.57793539326875,-2.20436481887379,
5.18910312454434));
#21951=CARTESIAN_POINT('Ctrl Pts',(-3.42367004108366,-2.31235747464383,
5.17798933548752));
#21952=CARTESIAN_POINT('Ctrl Pts',(-3.43073461124009,-2.5006515344537,5.16687554643073));
#21953=CARTESIAN_POINT('Ctrl Pts',(-3.59276310679123,-2.59677758279563,
5.15576175737392));
#21954=CARTESIAN_POINT('Ctrl Pts',(-3.76139893588905,-2.51281111117365,
5.14464796831712));
#21955=CARTESIAN_POINT('Ctrl Pts',(-3.78231281687012,-2.32557724598507,
5.13353417926031));
#21956=CARTESIAN_POINT('Ctrl Pts',(-3.63634954990495,-2.2064684174952,5.12242039020351));
#21957=CARTESIAN_POINT('Ctrl Pts',(-3.4571172047087,-2.26449872135838,5.1113066011467));
#21958=CARTESIAN_POINT('Ctrl Pts',(-3.40866606518746,-2.44655614068022,
5.10019281208991));
#21959=CARTESIAN_POINT('Ctrl Pts',(-3.53534556407432,-2.58599956800273,
5.08907902303309));
#21960=CARTESIAN_POINT('Ctrl Pts',(-3.72120374270903,-2.55519579519918,
5.0779652339763));
#21961=CARTESIAN_POINT('Ctrl Pts',(-3.79612289028458,-2.3823393942772,5.06685144491949));
#21962=CARTESIAN_POINT('Ctrl Pts',(-3.69152846768288,-2.22564802432955,
5.05573765586268));
#21963=CARTESIAN_POINT('Ctrl Pts',(-3.503157032826,-2.22854295591068,5.04462386680587));
#21964=CARTESIAN_POINT('Ctrl Pts',(-3.40342704800776,-2.38837448392236,
5.03351007774909));
#21965=CARTESIAN_POINT('Ctrl Pts',(-3.483622523472,-2.55884696889381,5.02239628869226));
#21966=CARTESIAN_POINT('Ctrl Pts',(-3.670339619,-2.58392502665791,5.01128249963547));
#21967=CARTESIAN_POINT('Ctrl Pts',(-3.79267406555566,-2.44065441923915,
5.00016871057867));
#21968=CARTESIAN_POINT('Ctrl Pts',(-3.73865175383498,-2.26017236205245,
4.98905492152186));
#21969=CARTESIAN_POINT('Ctrl Pts',(-3.55771991991106,-2.20767612702608,
4.97794113246506));
#21970=CARTESIAN_POINT('Ctrl Pts',(-3.4154875225317,-2.3312161143366,4.96682734340825));
#21971=CARTESIAN_POINT('Ctrl Pts',(-3.44214148841752,-2.51771477210593,
4.95571355435145));
#21972=CARTESIAN_POINT('Ctrl Pts',(-3.61328514012983,-2.59646776406591,
4.94459976529465));
#21973=CARTESIAN_POINT('Ctrl Pts',(-3.77226875244865,-2.49539158344266,
4.93348597623784));
#21974=CARTESIAN_POINT('Ctrl Pts',(-3.77357282197517,-2.30700240469905,
4.92237218718103));
#21975=CARTESIAN_POINT('Ctrl Pts',(-3.61600371910589,-2.20373497958946,
4.91125839812423));
#21976=CARTESIAN_POINT('Ctrl Pts',(-3.44378623064059,-2.28011115346305,
4.90014460906743));
#21977=CARTESIAN_POINT('Ctrl Pts',(-3.41455297685654,-2.46622294820157,
4.88903082001062));
#21978=CARTESIAN_POINT('Ctrl Pts',(-3.555061486467,-2.59172012743304,4.87791703095382));
#21979=CARTESIAN_POINT('Ctrl Pts',(-3.73670272715212,-2.54173369977035,
4.86680324189701));
#21980=CARTESIAN_POINT('Ctrl Pts',(-3.79321841136028,-2.36201680933867,
4.85568945284021));
#21981=CARTESIAN_POINT('Ctrl Pts',(-3.67287909240468,-2.21706636407783,
4.8445756637834));
#21982=CARTESIAN_POINT('Ctrl Pts',(-3.48583271366589,-2.23955715038517,
4.83346187472661));
#21983=CARTESIAN_POINT('Ctrl Pts',(-3.40328494685383,-2.40890309649059,
4.82234808566979));
#21984=CARTESIAN_POINT('Ctrl Pts',(-3.50079269908688,-2.57009993741021,
4.811234296613));
#21985=CARTESIAN_POINT('Ctrl Pts',(-3.68910601893303,-2.57560237655376,
4.80012050755619));
#21986=CARTESIAN_POINT('Ctrl Pts',(-3.79585958911879,-2.42037396897126,
4.78900671849938));
#21987=CARTESIAN_POINT('Ctrl Pts',(-3.72334065618531,-2.24649703653284,
4.77789292944258));
#21988=CARTESIAN_POINT('Ctrl Pts',(-3.53792662186724,-2.21312310739792,
4.76677914038578));
#21989=CARTESIAN_POINT('Ctrl Pts',(-3.40932905451407,-2.35079971738979,
4.75566535132897));
#21990=CARTESIAN_POINT('Ctrl Pts',(-3.45525476591977,-2.53350990402394,
4.74455156227217));
#21991=CARTESIAN_POINT('Ctrl Pts',(-3.6336674316017,-2.59401696139969,4.73343777321536));
#21992=CARTESIAN_POINT('Ctrl Pts',(-3.78126391532395,-2.47693809370431,
4.72232398415856));
#21993=CARTESIAN_POINT('Ctrl Pts',(-3.76294748167758,-2.28943691630404,
4.71121019510175));
#21994=CARTESIAN_POINT('Ctrl Pts',(-3.59548337010158,-2.20313538328135,
4.70009640604495));
#21995=CARTESIAN_POINT('Ctrl Pts',(-3.43215338109369,-2.29702626653782,
4.68898261698815));
#21996=CARTESIAN_POINT('Ctrl Pts',(-3.42245530588083,-2.48517017583382,
4.67786882793134));
#21997=CARTESIAN_POINT('Ctrl Pts',(-3.5752659026891,-2.59535685729358,4.66675503887453));
#21998=CARTESIAN_POINT('Ctrl Pts',(-3.75071589926964,-2.5267311917752,4.65564124981774));
#21999=CARTESIAN_POINT('Ctrl Pts',(-3.7882139240144,-2.34210702919526,4.64452746076093));
#22000=CARTESIAN_POINT('Ctrl Pts',(-3.65343760961716,-2.21047295934436,
4.63341367170412));
#22001=CARTESIAN_POINT('Ctrl Pts',(-3.46974924511472,-2.25231513918736,
4.62229988264733));
#22002=CARTESIAN_POINT('Ctrl Pts',(-3.4052808737006,-2.42933494699449,4.61118609359051));
#22003=CARTESIAN_POINT('Ctrl Pts',(-3.51904112685782,-2.57950414513246,
4.60007230453372));
#22004=CARTESIAN_POINT('Ctrl Pts',(-3.7069039547293,-2.5653711635236,4.5889585154769));
#22005=CARTESIAN_POINT('Ctrl Pts',(-3.79691638048147,-2.39987208048827,
4.57784472642011));
#22006=CARTESIAN_POINT('Ctrl Pts',(-3.7066890099598,-2.23449008366631,4.5667309373633));
#22007=CARTESIAN_POINT('Ctrl Pts',(-3.51880797875736,-2.22060119020745,
4.5556171483065));
#22008=CARTESIAN_POINT('Ctrl Pts',(-3.40524292523608,-2.37091806200724,
4.54450335924969));
#22009=CARTESIAN_POINT('Ctrl Pts',(-3.46994123122676,-2.54785396119378,
4.53338957019289));
#22010=CARTESIAN_POINT('Ctrl Pts',(-3.65368380267146,-2.5894574534616,4.52227578113609));
#22011=CARTESIAN_POINT('Ctrl Pts',(-3.78828898185839,-2.45764838890124,
4.51116199207927));
#22012=CARTESIAN_POINT('Ctrl Pts',(-3.75055111831899,-2.27307310236724,
4.50004820302248));
#22013=CARTESIAN_POINT('Ctrl Pts',(-3.57501211340008,-2.20467544035046,
4.48893441396567));
#22014=CARTESIAN_POINT('Ctrl Pts',(-3.42234479528953,-2.31506057159251,
4.47782062490887));
#22015=CARTESIAN_POINT('Ctrl Pts',(-3.43228731917671,-2.50319170755265,
4.46670683585206));
#22016=CARTESIAN_POINT('Ctrl Pts',(-3.59573912500965,-2.5968703381223,4.45559304679526));
#22017=CARTESIAN_POINT('Ctrl Pts',(-3.76309103173807,-2.51035124585066,
4.44447925773846));
#22018=CARTESIAN_POINT('Ctrl Pts',(-3.78116371996935,-2.32282654634568,
4.43336546868165));
#22019=CARTESIAN_POINT('Ctrl Pts',(-3.63341549627273,-2.20593930471439,
4.42225167962485));
#22020=CARTESIAN_POINT('Ctrl Pts',(-3.45508109817058,-2.26667857787915,
4.41113789056804));
#22021=CARTESIAN_POINT('Ctrl Pts',(-3.40939379925969,-2.449447340115,4.40002410151124));
#22022=CARTESIAN_POINT('Ctrl Pts',(-3.53816814492384,-2.58695863501888,
4.38891031245443));
#22023=CARTESIAN_POINT('Ctrl Pts',(-3.72354263968583,-2.55334007789814,
4.37779652339763));
#22024=CARTESIAN_POINT('Ctrl Pts',(-3.79582764186986,-2.379376605665,4.36668273434082));
#22025=CARTESIAN_POINT('Ctrl Pts',(-3.68888843287276,-2.22427194384119,
4.35556894528402));
#22026=CARTESIAN_POINT('Ctrl Pts',(-3.50055048149309,-2.23004924262897,
4.34445515622722));
#22027=CARTESIAN_POINT('Ctrl Pts',(-3.40331626422378,-2.3913121322753,4.33334136717041));
#22028=CARTESIAN_POINT('Ctrl Pts',(-3.48595487307994,-2.5606721137969,4.32222757811361));
#22029=CARTESIAN_POINT('Ctrl Pts',(-3.67329947146103,-2.58267280766239,
4.3111137890568));
#22030=CARTESIAN_POINT('Ctrl Pts',(-3.75289776062778,-2.48629498572916,
4.30370459635227));
#22031=CARTESIAN_POINT('Ctrl Pts',(-3.76351293272515,-2.4319230454628,4.3));
#22032=CARTESIAN_POINT('Ctrl Pts',(-3.76638442554721,-2.39990578503699,
5.13785196366098));
#22033=CARTESIAN_POINT('Ctrl Pts',(-3.76649613683224,-2.3783172805639,5.13641270219409));
#22034=CARTESIAN_POINT('Ctrl Pts',(-3.76259705167907,-2.35676746354197,
5.1349734407272));
#22035=CARTESIAN_POINT('Ctrl Pts',(-3.75449995887908,-2.33693141876819,
5.13353417926032));
#22036=CARTESIAN_POINT('Ctrl Pts',(-3.73365839454839,-2.28587430315511,
5.12982958290805));
#22037=CARTESIAN_POINT('Ctrl Pts',(-3.68500397222667,-2.24617136032516,
5.12612498655578));
#22038=CARTESIAN_POINT('Ctrl Pts',(-3.6308047035331,-2.23599160622071,5.12242039020351));
#22039=CARTESIAN_POINT('Ctrl Pts',(-3.57660543483953,-2.22581185211626,
5.11871579385124));
#22040=CARTESIAN_POINT('Ctrl Pts',(-3.51686131977411,-2.24515528673732,
5.11501119749897));
#22041=CARTESIAN_POINT('Ctrl Pts',(-3.4789140723212,-2.28516990726816,5.1113066011467));
#22042=CARTESIAN_POINT('Ctrl Pts',(-3.44096682486829,-2.32518452779899,
5.10760200479444));
#22043=CARTESIAN_POINT('Ctrl Pts',(-3.42481644502788,-2.3858703342396,5.10389740844217));
#22044=CARTESIAN_POINT('Ctrl Pts',(-3.43785450492215,-2.43945380868033,
5.1001928120899));
#22045=CARTESIAN_POINT('Ctrl Pts',(-3.45089256481642,-2.49303728312105,
5.09648821573763));
#22046=CARTESIAN_POINT('Ctrl Pts',(-3.49311906444537,-2.53951842556189,
5.09278361938536));
#22047=CARTESIAN_POINT('Ctrl Pts',(-3.54520867736563,-2.55762503464839,
5.08907902303309));
#22048=CARTESIAN_POINT('Ctrl Pts',(-3.59729829028589,-2.57573164373488,
5.08537442668083));
#22049=CARTESIAN_POINT('Ctrl Pts',(-3.65925101649746,-2.56546371946703,
5.08166983032856));
#22050=CARTESIAN_POINT('Ctrl Pts',(-3.70271390419917,-2.53152035717944,
5.07796523397629));
#22051=CARTESIAN_POINT('Ctrl Pts',(-3.74226404589835,-2.50063274572034,
5.07459414387119));
#22052=CARTESIAN_POINT('Ctrl Pts',(-3.76650359324528,-2.4501405807959,5.07122305376609));
#22053=CARTESIAN_POINT('Ctrl Pts',(-3.7668206250807,-2.39991359866148,5.06785196366098));
#22054=CARTESIAN_POINT('Ctrl Pts',(-3.65301702171886,-2.59851743256717,
5.2));
#22055=CARTESIAN_POINT('Ctrl Pts',(-3.66542047324148,-2.59392489431986,
5.2));
#22056=CARTESIAN_POINT('Ctrl Pts',(-3.67726976851323,-2.58806562778896,
5.2));
#22057=CARTESIAN_POINT('Ctrl Pts',(-3.6884471572875,-2.58110287343,5.2));
#22058=CARTESIAN_POINT('Ctrl Pts',(-3.69411332072466,-2.57757323829184,
5.2));
#22059=CARTESIAN_POINT('Ctrl Pts',(-3.69960638117381,-2.57375928297626,
5.2));
#22060=CARTESIAN_POINT('Ctrl Pts',(-3.70490756348411,-2.56967869660782,
5.2));
#22061=CARTESIAN_POINT('Ctrl Pts',(-3.7094943667238,-2.56614800370216,5.2));
#22062=CARTESIAN_POINT('Ctrl Pts',(-3.71393749668481,-2.56241764644412,
5.2));
#22063=CARTESIAN_POINT('Ctrl Pts',(-3.71822298464189,-2.55849819748795,
5.2));
#22064=CARTESIAN_POINT('Ctrl Pts',(-3.7213335990699,-2.55565327187038,5.2));
#22065=CARTESIAN_POINT('Ctrl Pts',(-3.72435497328541,-2.55271413748664,
5.2));
#22066=CARTESIAN_POINT('Ctrl Pts',(-3.72727770073803,-2.54969101779411,
5.2));
#22067=CARTESIAN_POINT('Ctrl Pts',(-3.73622270492435,-2.54043876326685,
5.2));
#22068=CARTESIAN_POINT('Ctrl Pts',(-3.7442634301432,-2.53038665580988,5.2));
#22069=CARTESIAN_POINT('Ctrl Pts',(-3.75126083636282,-2.51966573521934,
5.2));
#22070=CARTESIAN_POINT('Ctrl Pts',(-3.75579169616378,-2.51272387896453,
5.2));
#22071=CARTESIAN_POINT('Ctrl Pts',(-3.75988429343086,-2.5055010355982,5.2));
#22072=CARTESIAN_POINT('Ctrl Pts',(-3.76348914806144,-2.49803012759629,
5.2));
#22073=CARTESIAN_POINT('Ctrl Pts',(-3.76515593070928,-2.49457579140323,
5.2));
#22074=CARTESIAN_POINT('Ctrl Pts',(-3.76671430859645,-2.49107651026494,
5.2));
#22075=CARTESIAN_POINT('Ctrl Pts',(-3.76815914917795,-2.48753923965477,
5.2));
#22076=CARTESIAN_POINT('Ctrl Pts',(-3.77216127817835,-2.47774119447769,
5.2));
#22077=CARTESIAN_POINT('Ctrl Pts',(-3.77529843764987,-2.46764366345261,
5.2));
#22078=CARTESIAN_POINT('Ctrl Pts',(-3.77747651250232,-2.45732003292749,
5.2));
#22079=CARTESIAN_POINT('Ctrl Pts',(-3.779330303747,-2.44853344055707,5.2));
#22080=CARTESIAN_POINT('Ctrl Pts',(-3.78048859875581,-2.43958258054595,
5.2));
#22081=CARTESIAN_POINT('Ctrl Pts',(-3.78096402676373,-2.43054575199388,
5.2));
#22082=CARTESIAN_POINT('Ctrl Pts',(-3.78113316899519,-2.42733073453364,
5.2));
#22083=CARTESIAN_POINT('Ctrl Pts',(-3.78121551844131,-2.4241062749112,5.2));
#22084=CARTESIAN_POINT('Ctrl Pts',(-3.78121200526832,-2.42088560814198,
5.2));
#22085=CARTESIAN_POINT('Ctrl Pts',(-3.78119923320481,-2.40917694458053,
5.2));
#22086=CARTESIAN_POINT('Ctrl Pts',(-3.78005717128054,-2.39748206272171,
5.2));
#22087=CARTESIAN_POINT('Ctrl Pts',(-3.77783120534438,-2.38597327518306,
5.2));
#22088=CARTESIAN_POINT('Ctrl Pts',(-3.77668820057652,-2.38006366137664,
5.2));
#22089=CARTESIAN_POINT('Ctrl Pts',(-3.77525871074905,-2.37420329819383,
5.2));
#22090=CARTESIAN_POINT('Ctrl Pts',(-3.77354495279965,-2.36841778018193,
5.2));
#22091=CARTESIAN_POINT('Ctrl Pts',(-3.771857709037,-2.36272177207139,5.2));
#22092=CARTESIAN_POINT('Ctrl Pts',(-3.76989216970551,-2.35709287385817,
5.2));
#22093=CARTESIAN_POINT('Ctrl Pts',(-3.76766230775392,-2.35158840548752,
5.2));
#22094=CARTESIAN_POINT('Ctrl Pts',(-3.76420558159522,-2.34305539303218,
5.2));
#22095=CARTESIAN_POINT('Ctrl Pts',(-3.76011199819993,-2.33480777321703,
5.2));
#22096=CARTESIAN_POINT('Ctrl Pts',(-3.75539090007917,-2.32694141045687,
5.2));
#22097=CARTESIAN_POINT('Ctrl Pts',(-3.75297689160326,-2.32291915421652,
5.2));
#22098=CARTESIAN_POINT('Ctrl Pts',(-3.75039789394566,-2.31899648610286,
5.2));
#22099=CARTESIAN_POINT('Ctrl Pts',(-3.74766394659108,-2.31519991459367,
5.2));
#22100=CARTESIAN_POINT('Ctrl Pts',(-3.7422293448357,-2.30765300475514,5.2));
#22101=CARTESIAN_POINT('Ctrl Pts',(-3.73617584795258,-2.30058959872182,
5.2));
#22102=CARTESIAN_POINT('Ctrl Pts',(-3.7295081063639,-2.29412082362908,5.2));
#22103=CARTESIAN_POINT('Ctrl Pts',(-3.72872963705521,-2.29336558397147,
5.2));
#22104=CARTESIAN_POINT('Ctrl Pts',(-3.72794278071792,-2.29261847520289,
5.2));
#22105=CARTESIAN_POINT('Ctrl Pts',(-3.72714769448934,-2.29187956305505,
5.2));
#22106=CARTESIAN_POINT('Origin',(-3.6,-2.4,4.7));
#22107=CARTESIAN_POINT('Origin',(3.6,-2.4,4.2));
#22108=CARTESIAN_POINT('Origin',(-3.6,-2.4,4.2));
#22109=CARTESIAN_POINT('Origin',(-3.6,2.4,4.2));
#22110=CARTESIAN_POINT('Origin',(3.6,2.4,4.2));
#22111=CARTESIAN_POINT('Origin',(-4.6,0.,0.3));
#22112=CARTESIAN_POINT('',(-4.9,3.67394039744206E-17,0.6));
#22113=CARTESIAN_POINT('Origin',(-4.6,0.,0.6));
#22114=CARTESIAN_POINT('',(-4.9,3.67394039744206E-17,0.));
#22115=CARTESIAN_POINT('',(-4.9,3.67394039744206E-17,0.3));
#22116=CARTESIAN_POINT('Origin',(-4.6,0.,0.));
#22117=CARTESIAN_POINT('Origin',(4.6,0.,0.3));
#22118=CARTESIAN_POINT('',(4.3,3.67394039744206E-17,0.6));
#22119=CARTESIAN_POINT('Origin',(4.6,0.,0.6));
#22120=CARTESIAN_POINT('',(4.3,3.67394039744206E-17,0.));
#22121=CARTESIAN_POINT('',(4.3,3.67394039744206E-17,0.3));
#22122=CARTESIAN_POINT('Origin',(4.6,0.,0.));
#22123=CARTESIAN_POINT('Origin',(5.2,1.,0.));
#22124=CARTESIAN_POINT('',(5.2,1.,0.));
#22125=CARTESIAN_POINT('',(4.,1.,0.));
#22126=CARTESIAN_POINT('',(5.2,1.,0.));
#22127=CARTESIAN_POINT('',(4.,1.,0.6));
#22128=CARTESIAN_POINT('',(4.,1.,0.));
#22129=CARTESIAN_POINT('',(5.2,1.,0.6));
#22130=CARTESIAN_POINT('',(5.2,1.,0.6));
#22131=CARTESIAN_POINT('',(5.2,1.,0.));
#22132=CARTESIAN_POINT('Origin',(5.2,-1.,0.));
#22133=CARTESIAN_POINT('',(5.2,-1.,0.));
#22134=CARTESIAN_POINT('',(5.2,-1.,0.));
#22135=CARTESIAN_POINT('',(5.2,-1.,0.6));
#22136=CARTESIAN_POINT('',(5.2,-1.,0.6));
#22137=CARTESIAN_POINT('',(5.2,-1.,0.));
#22138=CARTESIAN_POINT('Origin',(4.,-1.,0.));
#22139=CARTESIAN_POINT('',(4.,-1.,0.));
#22140=CARTESIAN_POINT('',(4.,-1.,0.));
#22141=CARTESIAN_POINT('',(4.,-1.,0.6));
#22142=CARTESIAN_POINT('',(4.,-1.,0.6));
#22143=CARTESIAN_POINT('',(4.,-1.,0.));
#22144=CARTESIAN_POINT('Origin',(4.6,0.,0.6));
#22145=CARTESIAN_POINT('',(4.,-1.4,0.6));
#22146=CARTESIAN_POINT('Origin',(-4.,1.,0.));
#22147=CARTESIAN_POINT('',(-4.,1.,0.));
#22148=CARTESIAN_POINT('',(-5.2,1.,0.));
#22149=CARTESIAN_POINT('',(-4.,1.,0.));
#22150=CARTESIAN_POINT('',(-5.2,1.,0.6));
#22151=CARTESIAN_POINT('',(-5.2,1.,0.));
#22152=CARTESIAN_POINT('',(-4.,1.,0.6));
#22153=CARTESIAN_POINT('',(-4.,1.,0.6));
#22154=CARTESIAN_POINT('',(-4.,1.,0.));
#22155=CARTESIAN_POINT('Origin',(-5.2,-1.,0.));
#22156=CARTESIAN_POINT('',(-5.2,-1.,0.));
#22157=CARTESIAN_POINT('',(-4.,-1.,0.));
#22158=CARTESIAN_POINT('',(-5.2,-1.,0.));
#22159=CARTESIAN_POINT('',(-4.,-1.,0.6));
#22160=CARTESIAN_POINT('',(-4.,-1.,0.));
#22161=CARTESIAN_POINT('',(-5.2,-1.,0.6));
#22162=CARTESIAN_POINT('',(-5.2,-1.,0.6));
#22163=CARTESIAN_POINT('',(-5.2,-1.,0.));
#22164=CARTESIAN_POINT('Origin',(-5.2,1.,0.));
#22165=CARTESIAN_POINT('',(-5.2,1.,0.));
#22166=CARTESIAN_POINT('',(-5.2,1.,0.6));
#22167=CARTESIAN_POINT('Origin',(-4.6,0.,0.6));
#22168=CARTESIAN_POINT('',(-4.,1.4,0.6));
#22169=CARTESIAN_POINT('Origin',(0.,0.,0.8));
#22170=CARTESIAN_POINT('',(-0.65,-7.9602041944578E-17,1.4));
#22171=CARTESIAN_POINT('Origin',(0.,0.,1.4));
#22172=CARTESIAN_POINT('',(-0.65,-7.9602041944578E-17,0.8));
#22173=CARTESIAN_POINT('',(-0.65,-7.9602041944578E-17,0.8));
#22174=CARTESIAN_POINT('Origin',(0.,0.,0.8));
#22175=CARTESIAN_POINT('Origin',(0.,0.,0.8));
#22176=CARTESIAN_POINT('',(-0.8,-9.79717439317883E-17,1.4));
#22177=CARTESIAN_POINT('Origin',(0.,0.,1.4));
#22178=CARTESIAN_POINT('',(-0.8,-9.79717439317883E-17,0.8));
#22179=CARTESIAN_POINT('',(-0.8,-9.79717439317883E-17,0.8));
#22180=CARTESIAN_POINT('Origin',(0.,0.,0.8));
#22181=CARTESIAN_POINT('Origin',(0.,0.,1.4));
#22182=CARTESIAN_POINT('Origin',(0.,0.,0.8));
#22183=CARTESIAN_POINT('',(-3.,2.,0.8));
#22184=CARTESIAN_POINT('',(-3.2,1.8,0.8));
#22185=CARTESIAN_POINT('Origin',(-3.,1.8,0.8));
#22186=CARTESIAN_POINT('',(-3.2,-1.8,0.8));
#22187=CARTESIAN_POINT('',(-3.2,2.,0.8));
#22188=CARTESIAN_POINT('',(-3.,-2.,0.8));
#22189=CARTESIAN_POINT('Origin',(-3.,-1.8,0.8));
#22190=CARTESIAN_POINT('',(3.,-2.,0.8));
#22191=CARTESIAN_POINT('',(-3.2,-2.,0.8));
#22192=CARTESIAN_POINT('',(3.2,-1.8,0.8));
#22193=CARTESIAN_POINT('Origin',(3.,-1.8,0.8));
#22194=CARTESIAN_POINT('',(3.2,1.8,0.8));
#22195=CARTESIAN_POINT('',(3.2,-2.,0.8));
#22196=CARTESIAN_POINT('',(3.,2.,0.8));
#22197=CARTESIAN_POINT('Origin',(3.,1.8,0.8));
#22198=CARTESIAN_POINT('',(3.2,2.,0.8));
#22199=CARTESIAN_POINT('Origin',(-3.,1.8,5.2));
#22200=CARTESIAN_POINT('',(-3.,2.,5.2));
#22201=CARTESIAN_POINT('',(-3.,2.,5.2));
#22202=CARTESIAN_POINT('',(-3.2,1.8,5.2));
#22203=CARTESIAN_POINT('Origin',(-3.,1.8,5.2));
#22204=CARTESIAN_POINT('',(-3.2,1.8,5.2));
#22205=CARTESIAN_POINT('Origin',(-3.2,2.,5.2));
#22206=CARTESIAN_POINT('',(3.,2.,5.2));
#22207=CARTESIAN_POINT('',(3.,2.,5.2));
#22208=CARTESIAN_POINT('',(-1.6,2.,5.2));
#22209=CARTESIAN_POINT('Origin',(3.,1.8,5.2));
#22210=CARTESIAN_POINT('',(3.2,1.8,5.2));
#22211=CARTESIAN_POINT('',(3.2,1.8,5.2));
#22212=CARTESIAN_POINT('Origin',(3.,1.8,5.2));
#22213=CARTESIAN_POINT('Origin',(3.2,2.,5.2));
#22214=CARTESIAN_POINT('',(3.2,-1.8,5.2));
#22215=CARTESIAN_POINT('',(3.2,-1.8,5.2));
#22216=CARTESIAN_POINT('',(3.2,1.,5.2));
#22217=CARTESIAN_POINT('Origin',(-3.,-1.8,5.2));
#22218=CARTESIAN_POINT('',(-3.2,-1.8,5.2));
#22219=CARTESIAN_POINT('',(-3.2,-1.8,5.2));
#22220=CARTESIAN_POINT('',(-3.,-2.,5.2));
#22221=CARTESIAN_POINT('Origin',(-3.,-1.8,5.2));
#22222=CARTESIAN_POINT('',(-3.,-2.,5.2));
#22223=CARTESIAN_POINT('Origin',(0.,0.,0.8));
#22224=CARTESIAN_POINT('Origin',(3.2,-2.,5.2));
#22225=CARTESIAN_POINT('',(3.,-2.,5.2));
#22226=CARTESIAN_POINT('',(1.6,-2.,5.2));
#22227=CARTESIAN_POINT('',(3.,-2.,5.2));
#22228=CARTESIAN_POINT('Origin',(3.,-1.8,5.2));
#22229=CARTESIAN_POINT('Origin',(3.,-1.8,5.2));
#22230=CARTESIAN_POINT('Origin',(-3.2,-2.,5.2));
#22231=CARTESIAN_POINT('',(-3.2,-1.,5.2));
#22232=CARTESIAN_POINT('Origin',(4.,2.8,0.));
#22233=CARTESIAN_POINT('',(4.,2.8,0.));
#22234=CARTESIAN_POINT('',(-4.,2.8,0.));
#22235=CARTESIAN_POINT('',(4.,2.8,0.));
#22236=CARTESIAN_POINT('',(-4.,2.8,5.2));
#22237=CARTESIAN_POINT('',(-4.,2.8,0.));
#22238=CARTESIAN_POINT('',(4.,2.8,5.2));
#22239=CARTESIAN_POINT('',(4.,2.8,5.2));
#22240=CARTESIAN_POINT('',(4.,2.8,0.));
#22241=CARTESIAN_POINT('Origin',(4.,-2.8,0.));
#22242=CARTESIAN_POINT('',(4.,-2.8,0.));
#22243=CARTESIAN_POINT('',(4.,-2.8,5.2));
#22244=CARTESIAN_POINT('',(4.,-2.8,5.2));
#22245=CARTESIAN_POINT('',(4.,-2.8,0.));
#22246=CARTESIAN_POINT('',(4.,-2.8,0.));
#22247=CARTESIAN_POINT('',(4.,-2.8,0.));
#22248=CARTESIAN_POINT('Origin',(-4.,-2.8,0.));
#22249=CARTESIAN_POINT('',(-4.,-2.8,0.));
#22250=CARTESIAN_POINT('',(-4.,-2.8,0.));
#22251=CARTESIAN_POINT('',(-4.,-2.8,5.2));
#22252=CARTESIAN_POINT('',(-4.,-2.8,5.2));
#22253=CARTESIAN_POINT('',(-4.,-2.8,0.));
#22254=CARTESIAN_POINT('Origin',(-4.,2.8,0.));
#22255=CARTESIAN_POINT('',(-4.,2.8,0.));
#22256=CARTESIAN_POINT('',(-4.,2.8,5.2));
#22257=CARTESIAN_POINT('',(-4.,2.8,0.));
#22258=CARTESIAN_POINT('Origin',(0.,0.,5.2));
#22259=CARTESIAN_POINT('Origin',(0.,0.,0.));
#43944=UNCERTAINTY_MEASURE_WITH_UNIT(LENGTH_MEASURE(0.001),#43981,
'DISTANCE_ACCURACY_VALUE',
'Maximum model space distance between geometric entities at asserted c
onnectivities');
#43961=UNCERTAINTY_MEASURE_WITH_UNIT(LENGTH_MEASURE(0.001),#43981,
'DISTANCE_ACCURACY_VALUE',
'Maximum model space distance between geometric entities at asserted c
onnectivities');
#43963=(
GEOMETRIC_REPRESENTATION_CONTEXT(3)
GLOBAL_UNCERTAINTY_ASSIGNED_CONTEXT((#43944))
GLOBAL_UNIT_ASSIGNED_CONTEXT((#43981,#43983,#43984))
REPRESENTATION_CONTEXT('','3D')
);
#43980=(
GEOMETRIC_REPRESENTATION_CONTEXT(3)
GLOBAL_UNCERTAINTY_ASSIGNED_CONTEXT((#43961))
GLOBAL_UNIT_ASSIGNED_CONTEXT((#43981,#43983,#43984))
REPRESENTATION_CONTEXT('','3D')
);
#43981=(
LENGTH_UNIT()
NAMED_UNIT(*)
SI_UNIT(.CENTI.,.METRE.)
);
#43983=(
NAMED_UNIT(*)
PLANE_ANGLE_UNIT()
SI_UNIT($,.RADIAN.)
);
#43984=(
NAMED_UNIT(*)
SI_UNIT($,.STERADIAN.)
SOLID_ANGLE_UNIT()
);
#43986=SHAPE_DEFINITION_REPRESENTATION(#44004,#44056);
#44004=PRODUCT_DEFINITION_SHAPE('',$,#44075);
#44056=SHAPE_REPRESENTATION('',(#11437),#43963);
#44073=PRODUCT_DEFINITION_CONTEXT('part definition',#44129,'design');
#44075=PRODUCT_DEFINITION('Switch housing','Switch housing',#44093,#44073);
#44093=PRODUCT_DEFINITION_FORMATION('',$,#44132);
#44129=APPLICATION_CONTEXT(
'Core Data for Automotive Mechanical Design Process');
#44130=PRODUCT_CONTEXT('part definition',#44129,'mechanical');
#44132=PRODUCT('Switch housing','Switch housing',$,(#44130));
#44150=PRESENTATION_STYLE_ASSIGNMENT((#44162));
#44162=SURFACE_STYLE_USAGE(.BOTH.,#44174);
#44174=SURFACE_SIDE_STYLE('',(#44186));
#44186=SURFACE_STYLE_FILL_AREA(#44198);
#44198=FILL_AREA_STYLE('Dark blue',(#44210));
#44210=FILL_AREA_STYLE_COLOUR('Dark blue',#44222);
#44222=COLOUR_RGB('Dark blue',0.0901960784313725,0.270588235294118,0.513725490196078);
ENDSEC;
END-ISO-10303-21;
